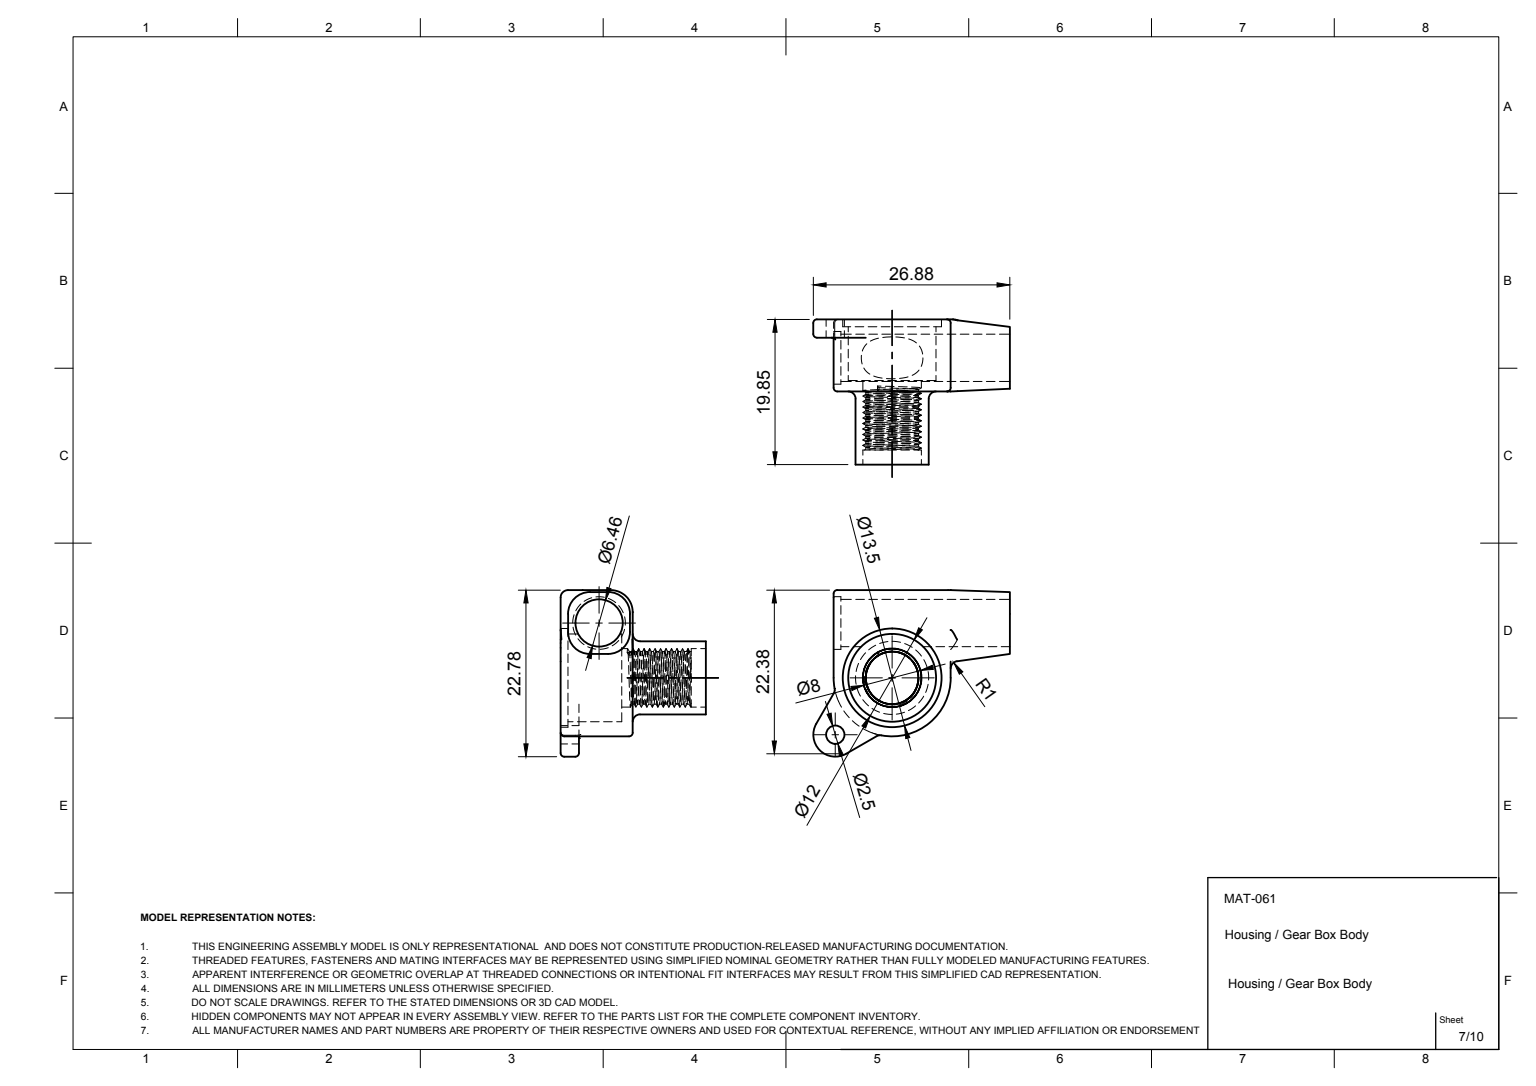
ISO-10303-21;
HEADER;
/* Generated by software containing ST-Developer
 * from STEP Tools, Inc. (www.steptools.com) 
 */

FILE_DESCRIPTION(
/* description */ ('', 'CAx-IF Rec.Pracs.---Representation and Presentation of Product Manufa
cturing Information (PMI)---4.0---2014-10-13'),
/* implementation_level */ '2;1');

FILE_NAME(
/* name */ 'Housing _ Gear Box Body.step',
/* time_stamp */ '2026-10-28T14:45:12+01:00',
/* author */ (''),
/* organization */ (''),
/* preprocessor_version */ 'ST-DEVELOPER v20.2',
/* originating_system */ 'Autodesk Translation Framework v15.17.0.0',
/* authorisation */ '');

FILE_SCHEMA (('AP242_MANAGED_MODEL_BASED_3D_ENGINEERING_MIM_LF { 1 0 10303 442 2 1 4 }'));
ENDSEC;

DATA;
#10=MECHANICAL_DESIGN_GEOMETRIC_PRESENTATION_REPRESENTATION('',(#265),#52164);
#116=ELLIPSE('',#10069,3.09185060411887,2.99998911300292);
#117=ELLIPSE('',#10070,0.558356536433831,0.540529130211527);
#118=ELLIPSE('',#10075,3.02534560825415,3.);
#119=ELLIPSE('',#10096,3.05201365986006,3.);
#120=ELLIPSE('',#10097,3.03164154875039,3.);
#121=ELLIPSE('',#10098,3.00479269659654,3.);
#122=ELLIPSE('',#10104,3.05599112671771,2.99998273953943);
#123=ELLIPSE('',#10106,0.477842904086099,0.430473129723059);
#124=ELLIPSE('',#10110,0.470434252195438,0.436250539297532);
#125=ELLIPSE('',#10111,0.502233427925589,0.501933027798313);
#126=ELLIPSE('',#10115,0.0333294784166319,0.012380355937192);
#180=(
BOUNDED_SURFACE()
B_SPLINE_SURFACE(3,3,((#43761,#43762,#43763,#43764,#43765,#43766,#43767,
#43768,#43769,#43770,#43771,#43772,#43773,#43774,#43775),(#43776,#43777,
#43778,#43779,#43780,#43781,#43782,#43783,#43784,#43785,#43786,#43787,#43788,
#43789,#43790),(#43791,#43792,#43793,#43794,#43795,#43796,#43797,#43798,
#43799,#43800,#43801,#43802,#43803,#43804,#43805),(#43806,#43807,#43808,
#43809,#43810,#43811,#43812,#43813,#43814,#43815,#43816,#43817,#43818,#43819,
#43820)),.UNSPECIFIED.,.F.,.F.,.F.)
B_SPLINE_SURFACE_WITH_KNOTS((4,4),(4,1,1,1,1,1,1,1,1,1,1,1,4),(0.,1.),(-0.02367250505126,
0.,0.1568376273924,0.2958784950045,0.4193835102427,0.5294996966959,0.6286414323947,
0.7182158704286,0.7992496439752,0.8730760680591,0.9399209839788,1.,1.025375300283),
 .UNSPECIFIED.)
GEOMETRIC_REPRESENTATION_ITEM()
RATIONAL_B_SPLINE_SURFACE(((1.19686984414,1.19686984414,1.19686984414,1.19686984414,
1.19686984414,1.19686984414,1.19686984414,1.19686984414,1.19686984414,1.19686984414,
1.19686984414,1.19686984414,1.19686984414,1.19686984414,1.19686984414),
(0.9343767186201,0.9343767186201,0.9343767186201,0.9343767186201,0.9343767186201,
0.9343767186201,0.9343767186201,0.9343767186201,0.9343767186201,0.9343767186201,
0.9343767186201,0.9343767186201,0.9343767186201,0.9343767186201,0.9343767186201),
(0.9343767186201,0.9343767186201,0.9343767186201,0.9343767186201,0.9343767186201,
0.9343767186201,0.9343767186201,0.9343767186201,0.9343767186201,0.9343767186201,
0.9343767186201,0.9343767186201,0.9343767186201,0.9343767186201,0.9343767186201),
(1.19686984414,1.19686984414,1.19686984414,1.19686984414,1.19686984414,
1.19686984414,1.19686984414,1.19686984414,1.19686984414,1.19686984414,1.19686984414,
1.19686984414,1.19686984414,1.19686984414,1.19686984414)))
REPRESENTATION_ITEM('')
SURFACE()
);
#181=(
BOUNDED_SURFACE()
B_SPLINE_SURFACE(3,3,((#43843,#43844,#43845,#43846,#43847,#43848,#43849,
#43850,#43851,#43852,#43853,#43854,#43855,#43856,#43857),(#43858,#43859,
#43860,#43861,#43862,#43863,#43864,#43865,#43866,#43867,#43868,#43869,#43870,
#43871,#43872),(#43873,#43874,#43875,#43876,#43877,#43878,#43879,#43880,
#43881,#43882,#43883,#43884,#43885,#43886,#43887),(#43888,#43889,#43890,
#43891,#43892,#43893,#43894,#43895,#43896,#43897,#43898,#43899,#43900,#43901,
#43902)),.UNSPECIFIED.,.F.,.F.,.F.)
B_SPLINE_SURFACE_WITH_KNOTS((4,4),(4,1,1,1,1,1,1,1,1,1,1,1,4),(0.,1.),(-0.02541201080131,
0.,0.06012137477617,0.127023679674,0.2009097013355,0.2820155865859,0.3717063075714,
0.470928205433,0.5809950476801,0.7044646083568,0.8434955500304,1.,1.023466062398),
 .UNSPECIFIED.)
GEOMETRIC_REPRESENTATION_ITEM()
RATIONAL_B_SPLINE_SURFACE(((1.196861975576,1.196861975576,1.196861975576,
1.196861975576,1.196861975576,1.196861975576,1.196861975576,1.196861975576,
1.196861975576,1.196861975576,1.196861975576,1.196861975576,1.196861975576,
1.196861975576,1.196861975576),(0.9343793414748,0.9343793414748,0.9343793414748,
0.9343793414748,0.9343793414748,0.9343793414748,0.9343793414748,0.9343793414748,
0.9343793414748,0.9343793414748,0.9343793414748,0.9343793414748,0.9343793414748,
0.9343793414748,0.9343793414748),(0.9343793414748,0.9343793414748,0.9343793414748,
0.9343793414748,0.9343793414748,0.9343793414748,0.9343793414748,0.9343793414748,
0.9343793414748,0.9343793414748,0.9343793414748,0.9343793414748,0.9343793414748,
0.9343793414748,0.9343793414748),(1.196861975576,1.196861975576,1.196861975576,
1.196861975576,1.196861975576,1.196861975576,1.196861975576,1.196861975576,
1.196861975576,1.196861975576,1.196861975576,1.196861975576,1.196861975576,
1.196861975576,1.196861975576)))
REPRESENTATION_ITEM('')
SURFACE()
);
#182=(
BOUNDED_SURFACE()
B_SPLINE_SURFACE(3,3,((#44165,#44166,#44167,#44168,#44169,#44170,#44171,
#44172,#44173,#44174,#44175,#44176,#44177,#44178,#44179,#44180,#44181,#44182,
#44183,#44184,#44185),(#44186,#44187,#44188,#44189,#44190,#44191,#44192,
#44193,#44194,#44195,#44196,#44197,#44198,#44199,#44200,#44201,#44202,#44203,
#44204,#44205,#44206),(#44207,#44208,#44209,#44210,#44211,#44212,#44213,
#44214,#44215,#44216,#44217,#44218,#44219,#44220,#44221,#44222,#44223,#44224,
#44225,#44226,#44227),(#44228,#44229,#44230,#44231,#44232,#44233,#44234,
#44235,#44236,#44237,#44238,#44239,#44240,#44241,#44242,#44243,#44244,#44245,
#44246,#44247,#44248)),.UNSPECIFIED.,.F.,.F.,.F.)
B_SPLINE_SURFACE_WITH_KNOTS((4,4),(4,1,1,1,1,1,1,1,1,1,1,1,1,1,1,1,1,1,
4),(0.,1.),(-0.004474348485776,0.,0.02230597305244,0.04333157365729,0.06387325262822,
0.08408116383947,0.1041708278111,0.1243458370088,0.1448121265696,0.1657786860045,
0.187470853701,0.210486087144,0.2358855836333,0.2645487659469,0.2971408212892,
0.3344049750459,0.3761308583034,0.4203483673292,0.4513668076816),
 .UNSPECIFIED.)
GEOMETRIC_REPRESENTATION_ITEM()
RATIONAL_B_SPLINE_SURFACE(((1.162548312769,1.162548312769,1.162548312769,
1.162548312769,1.162548312769,1.162548312769,1.162548312769,1.162548312769,
1.162548312769,1.162548312769,1.162548312769,1.162548312769,1.162548312769,
1.162548312769,1.162548312769,1.162548312769,1.162548312769,1.162548312769,
1.162548312769,1.162548312769,1.162548312769),(0.9458172290769,0.9458172290769,
0.9458172290769,0.9458172290769,0.9458172290769,0.9458172290769,0.9458172290769,
0.9458172290769,0.9458172290769,0.9458172290769,0.9458172290769,0.9458172290769,
0.9458172290769,0.9458172290769,0.9458172290769,0.9458172290769,0.9458172290769,
0.9458172290769,0.9458172290769,0.9458172290769,0.9458172290769),(0.9458172290769,
0.9458172290769,0.9458172290769,0.9458172290769,0.9458172290769,0.9458172290769,
0.9458172290769,0.9458172290769,0.9458172290769,0.9458172290769,0.9458172290769,
0.9458172290769,0.9458172290769,0.9458172290769,0.9458172290769,0.9458172290769,
0.9458172290769,0.9458172290769,0.9458172290769,0.9458172290769,0.9458172290769),
(1.162548312769,1.162548312769,1.162548312769,1.162548312769,1.162548312769,
1.162548312769,1.162548312769,1.162548312769,1.162548312769,1.162548312769,
1.162548312769,1.162548312769,1.162548312769,1.162548312769,1.162548312769,
1.162548312769,1.162548312769,1.162548312769,1.162548312769,1.162548312769,
1.162548312769)))
REPRESENTATION_ITEM('')
SURFACE()
);
#183=(
BOUNDED_SURFACE()
B_SPLINE_SURFACE(3,3,((#44380,#44381,#44382,#44383,#44384,#44385,#44386,
#44387,#44388,#44389,#44390,#44391,#44392,#44393,#44394,#44395,#44396,#44397,
#44398,#44399,#44400,#44401,#44402),(#44403,#44404,#44405,#44406,#44407,
#44408,#44409,#44410,#44411,#44412,#44413,#44414,#44415,#44416,#44417,#44418,
#44419,#44420,#44421,#44422,#44423,#44424,#44425),(#44426,#44427,#44428,
#44429,#44430,#44431,#44432,#44433,#44434,#44435,#44436,#44437,#44438,#44439,
#44440,#44441,#44442,#44443,#44444,#44445,#44446,#44447,#44448),(#44449,
#44450,#44451,#44452,#44453,#44454,#44455,#44456,#44457,#44458,#44459,#44460,
#44461,#44462,#44463,#44464,#44465,#44466,#44467,#44468,#44469,#44470,#44471)),
 .UNSPECIFIED.,.F.,.F.,.F.)
B_SPLINE_SURFACE_WITH_KNOTS((4,4),(4,1,1,1,1,1,1,1,1,1,1,1,1,1,1,1,1,1,
1,1,4),(0.,1.),(0.4402361434422,0.4558088659294,0.476422669633,0.4969107659322,
0.5173847665671,0.5378040004898,0.5584587769075,0.5804853326365,0.6053681688744,
0.6337471320501,0.6648770320844,0.697628000239,0.7315220485564,0.7658606197272,
0.7995217313545,0.8327434657359,0.8676912667687,0.9066066156032,0.9504140537645,
1.,1.005363326625),.UNSPECIFIED.)
GEOMETRIC_REPRESENTATION_ITEM()
RATIONAL_B_SPLINE_SURFACE(((1.224498979605,1.224498979605,1.224498979605,
1.224498979605,1.224498979605,1.224498979605,1.224498979605,1.224498979605,
1.224498979605,1.224498979605,1.224498979605,1.224498979605,1.224498979605,
1.224498979605,1.224498979605,1.224498979605,1.224498979605,1.224498979605,
1.224498979605,1.224498979605,1.224498979605,1.224498979605,1.224498979605),
(0.9251670067983,0.9251670067983,0.9251670067983,0.9251670067983,0.9251670067983,
0.9251670067983,0.9251670067983,0.9251670067983,0.9251670067983,0.9251670067983,
0.9251670067983,0.9251670067983,0.9251670067983,0.9251670067983,0.9251670067983,
0.9251670067983,0.9251670067983,0.9251670067983,0.9251670067983,0.9251670067983,
0.9251670067983,0.9251670067983,0.9251670067983),(0.9251670067983,0.9251670067983,
0.9251670067983,0.9251670067983,0.9251670067983,0.9251670067983,0.9251670067983,
0.9251670067983,0.9251670067983,0.9251670067983,0.9251670067983,0.9251670067983,
0.9251670067983,0.9251670067983,0.9251670067983,0.9251670067983,0.9251670067983,
0.9251670067983,0.9251670067983,0.9251670067983,0.9251670067983,0.9251670067983,
0.9251670067983),(1.224498979605,1.224498979605,1.224498979605,1.224498979605,
1.224498979605,1.224498979605,1.224498979605,1.224498979605,1.224498979605,
1.224498979605,1.224498979605,1.224498979605,1.224498979605,1.224498979605,
1.224498979605,1.224498979605,1.224498979605,1.224498979605,1.224498979605,
1.224498979605,1.224498979605,1.224498979605,1.224498979605)))
REPRESENTATION_ITEM('')
SURFACE()
);
#184=(
BOUNDED_SURFACE()
B_SPLINE_SURFACE(3,3,((#44501,#44502,#44503,#44504,#44505,#44506,#44507,
#44508),(#44509,#44510,#44511,#44512,#44513,#44514,#44515,#44516),(#44517,
#44518,#44519,#44520,#44521,#44522,#44523,#44524),(#44525,#44526,#44527,
#44528,#44529,#44530,#44531,#44532)),.UNSPECIFIED.,.F.,.F.,.F.)
B_SPLINE_SURFACE_WITH_KNOTS((4,4),(4,1,1,1,1,4),(0.,1.),(-0.02000817581934,
0.,0.3335678568848,0.6667501113936,1.,1.020000171272),.UNSPECIFIED.)
GEOMETRIC_REPRESENTATION_ITEM()
RATIONAL_B_SPLINE_SURFACE(((1.001084776474,1.001084776474,1.001084776474,
1.001084776474,1.001084776474,1.001084776474,1.001084776474,1.001084776474),
(0.9996384078421,0.9996384078421,0.9996384078421,0.9996384078421,0.9996384078421,
0.9996384078421,0.9996384078421,0.9996384078421),(0.9996384078421,0.9996384078421,
0.9996384078421,0.9996384078421,0.9996384078421,0.9996384078421,0.9996384078421,
0.9996384078421),(1.001084776474,1.001084776474,1.001084776474,1.001084776474,
1.001084776474,1.001084776474,1.001084776474,1.001084776474)))
REPRESENTATION_ITEM('')
SURFACE()
);
#185=(
BOUNDED_SURFACE()
B_SPLINE_SURFACE(3,3,((#44717,#44718,#44719,#44720,#44721,#44722,#44723,
#44724,#44725),(#44726,#44727,#44728,#44729,#44730,#44731,#44732,#44733,
#44734),(#44735,#44736,#44737,#44738,#44739,#44740,#44741,#44742,#44743),
(#44744,#44745,#44746,#44747,#44748,#44749,#44750,#44751,#44752)),
 .UNSPECIFIED.,.F.,.F.,.F.)
B_SPLINE_SURFACE_WITH_KNOTS((4,4),(4,1,1,1,1,1,4),(0.,1.),(0.01341438395161,
0.2268259504049,0.4456307994234,0.6496269485443,0.8352622055157,1.,1.015518229442),
 .UNSPECIFIED.)
GEOMETRIC_REPRESENTATION_ITEM()
RATIONAL_B_SPLINE_SURFACE(((1.058064131412,1.058064131412,1.058064131412,
1.058064131412,1.058064131412,1.058064131412,1.058064131412,1.058064131412,
1.058064131412),(0.9806452895294,0.9806452895294,0.9806452895294,0.9806452895294,
0.9806452895294,0.9806452895294,0.9806452895294,0.9806452895294,0.9806452895294),
(0.9806452895294,0.9806452895294,0.9806452895294,0.9806452895294,0.9806452895294,
0.9806452895294,0.9806452895294,0.9806452895294,0.9806452895294),(1.058064131412,
1.058064131412,1.058064131412,1.058064131412,1.058064131412,1.058064131412,
1.058064131412,1.058064131412,1.058064131412)))
REPRESENTATION_ITEM('')
SURFACE()
);
#186=(
BOUNDED_SURFACE()
B_SPLINE_SURFACE(3,3,((#44798,#44799,#44800,#44801,#44802,#44803,#44804,
#44805,#44806,#44807,#44808),(#44809,#44810,#44811,#44812,#44813,#44814,
#44815,#44816,#44817,#44818,#44819),(#44820,#44821,#44822,#44823,#44824,
#44825,#44826,#44827,#44828,#44829,#44830),(#44831,#44832,#44833,#44834,
#44835,#44836,#44837,#44838,#44839,#44840,#44841)),.UNSPECIFIED.,.F.,.F.,
 .F.)
B_SPLINE_SURFACE_WITH_KNOTS((4,4),(4,1,1,1,1,1,1,1,4),(0.,1.),(-0.01514694021523,
0.,0.1434382549194,0.2925803126927,0.4539877256396,0.6288947339363,0.8127593843745,
1.,1.01468871823),.UNSPECIFIED.)
GEOMETRIC_REPRESENTATION_ITEM()
RATIONAL_B_SPLINE_SURFACE(((1.091722184379,1.091722184379,1.091722184379,
1.091722184379,1.091722184379,1.091722184379,1.091722184379,1.091722184379,
1.091722184379,1.091722184379,1.091722184379),(0.9694259385405,0.9694259385405,
0.9694259385405,0.9694259385405,0.9694259385405,0.9694259385405,0.9694259385405,
0.9694259385405,0.9694259385405,0.9694259385405,0.9694259385405),(0.9694259385405,
0.9694259385405,0.9694259385405,0.9694259385405,0.9694259385405,0.9694259385405,
0.9694259385405,0.9694259385405,0.9694259385405,0.9694259385405,0.9694259385405),
(1.091722184379,1.091722184379,1.091722184379,1.091722184379,1.091722184379,
1.091722184379,1.091722184379,1.091722184379,1.091722184379,1.091722184379,
1.091722184379)))
REPRESENTATION_ITEM('')
SURFACE()
);
#187=(
BOUNDED_SURFACE()
B_SPLINE_SURFACE(3,3,((#44843,#44844,#44845,#44846,#44847,#44848,#44849,
#44850,#44851,#44852),(#44853,#44854,#44855,#44856,#44857,#44858,#44859,
#44860,#44861,#44862),(#44863,#44864,#44865,#44866,#44867,#44868,#44869,
#44870,#44871,#44872),(#44873,#44874,#44875,#44876,#44877,#44878,#44879,
#44880,#44881,#44882)),.UNSPECIFIED.,.F.,.F.,.F.)
B_SPLINE_SURFACE_WITH_KNOTS((4,4),(4,1,1,1,1,1,1,4),(0.,1.),(-0.1017343672885,
0.,0.1958839083417,0.3858642890747,0.5744654073669,0.7741715521339,1.,1.116420456884),
 .UNSPECIFIED.)
GEOMETRIC_REPRESENTATION_ITEM()
RATIONAL_B_SPLINE_SURFACE(((1.126722516535,1.126722516535,1.126722516535,
1.126722516535,1.126722516535,1.126722516535,1.126722516535,1.126722516535,
1.126722516535,1.126722516535),(0.9577591611551,0.9577591611551,0.9577591611551,
0.9577591611551,0.9577591611551,0.9577591611551,0.9577591611551,0.9577591611551,
0.9577591611551,0.9577591611551),(0.9577591611551,0.9577591611551,0.9577591611551,
0.9577591611551,0.9577591611551,0.9577591611551,0.9577591611551,0.9577591611551,
0.9577591611551,0.9577591611551),(1.126722516535,1.126722516535,1.126722516535,
1.126722516535,1.126722516535,1.126722516535,1.126722516535,1.126722516535,
1.126722516535,1.126722516535)))
REPRESENTATION_ITEM('')
SURFACE()
);
#188=(
BOUNDED_SURFACE()
B_SPLINE_SURFACE(3,3,((#44916,#44917,#44918,#44919,#44920,#44921,#44922,
#44923,#44924,#44925,#44926,#44927,#44928,#44929),(#44930,#44931,#44932,
#44933,#44934,#44935,#44936,#44937,#44938,#44939,#44940,#44941,#44942,#44943),
(#44944,#44945,#44946,#44947,#44948,#44949,#44950,#44951,#44952,#44953,
#44954,#44955,#44956,#44957),(#44958,#44959,#44960,#44961,#44962,#44963,
#44964,#44965,#44966,#44967,#44968,#44969,#44970,#44971)),.UNSPECIFIED.,
 .F.,.F.,.F.)
B_SPLINE_SURFACE_WITH_KNOTS((4,4),(4,1,1,1,1,1,1,1,1,1,1,4),(0.,1.),(-0.01844658935295,
0.,0.1044814008579,0.2134723510049,0.3264520754444,0.4425667333534,0.5596708840584,
0.6752555152391,0.7879010159006,0.8964334098892,1.,1.018329622104),
 .UNSPECIFIED.)
GEOMETRIC_REPRESENTATION_ITEM()
RATIONAL_B_SPLINE_SURFACE(((1.093920437843,1.093920437843,1.093920437843,
1.093920437843,1.093920437843,1.093920437843,1.093920437843,1.093920437843,
1.093920437843,1.093920437843,1.093920437843,1.093920437843,1.093920437843,
1.093920437843),(0.9686931873855,0.9686931873855,0.9686931873855,0.9686931873855,
0.9686931873855,0.9686931873855,0.9686931873855,0.9686931873855,0.9686931873855,
0.9686931873855,0.9686931873855,0.9686931873855,0.9686931873855,0.9686931873855),
(0.9686931873855,0.9686931873855,0.9686931873855,0.9686931873855,0.9686931873855,
0.9686931873855,0.9686931873855,0.9686931873855,0.9686931873855,0.9686931873855,
0.9686931873855,0.9686931873855,0.9686931873855,0.9686931873855),(1.093920437843,
1.093920437843,1.093920437843,1.093920437843,1.093920437843,1.093920437843,
1.093920437843,1.093920437843,1.093920437843,1.093920437843,1.093920437843,
1.093920437843,1.093920437843,1.093920437843)))
REPRESENTATION_ITEM('')
SURFACE()
);
#189=(
BOUNDED_SURFACE()
B_SPLINE_SURFACE(3,3,((#45064,#45065,#45066,#45067,#45068,#45069,#45070,
#45071,#45072,#45073,#45074,#45075),(#45076,#45077,#45078,#45079,#45080,
#45081,#45082,#45083,#45084,#45085,#45086,#45087),(#45088,#45089,#45090,
#45091,#45092,#45093,#45094,#45095,#45096,#45097,#45098,#45099),(#45100,
#45101,#45102,#45103,#45104,#45105,#45106,#45107,#45108,#45109,#45110,#45111)),
 .UNSPECIFIED.,.F.,.F.,.F.)
B_SPLINE_SURFACE_WITH_KNOTS((4,4),(4,1,1,1,1,1,1,1,1,4),(0.,1.),(-0.030614617578,
0.,0.1495462512719,0.2937414136624,0.4389937202877,0.5830269670076,0.7175783131859,
0.8510090101071,1.,1.030661227764),.UNSPECIFIED.)
GEOMETRIC_REPRESENTATION_ITEM()
RATIONAL_B_SPLINE_SURFACE(((1.129761691476,1.129761691476,1.129761691476,
1.129761691476,1.129761691476,1.129761691476,1.129761691476,1.129761691476,
1.129761691476,1.129761691476,1.129761691476,1.129761691476),(0.9567461028415,
0.9567461028415,0.9567461028415,0.9567461028415,0.9567461028415,0.9567461028415,
0.9567461028415,0.9567461028415,0.9567461028415,0.9567461028415,0.9567461028415,
0.9567461028415),(0.9567461028415,0.9567461028415,0.9567461028415,0.9567461028415,
0.9567461028415,0.9567461028415,0.9567461028415,0.9567461028415,0.9567461028415,
0.9567461028415,0.9567461028415,0.9567461028415),(1.129761691476,1.129761691476,
1.129761691476,1.129761691476,1.129761691476,1.129761691476,1.129761691476,
1.129761691476,1.129761691476,1.129761691476,1.129761691476,1.129761691476)))
REPRESENTATION_ITEM('')
SURFACE()
);
#190=(
BOUNDED_SURFACE()
B_SPLINE_SURFACE(2,2,((#45185,#45186,#45187),(#45188,#45189,#45190),(#45191,
#45192,#45193)),.UNSPECIFIED.,.F.,.F.,.F.)
B_SPLINE_SURFACE_WITH_KNOTS((3,3),(3,3),(-1.57079632679603,1.03155351707746E-11),
(-0.78539816371462,0.785398163714621),.UNSPECIFIED.)
GEOMETRIC_REPRESENTATION_ITEM()
RATIONAL_B_SPLINE_SURFACE(((1.,0.707106780962273,1.),(0.707106781182504,
0.499999999838555,0.707106781182504),(1.,0.707106780962273,1.)))
REPRESENTATION_ITEM('')
SURFACE()
);
#191=(
BOUNDED_SURFACE()
B_SPLINE_SURFACE(3,3,((#45244,#45245,#45246,#45247,#45248,#45249,#45250,
#45251,#45252,#45253,#45254,#45255,#45256,#45257,#45258,#45259,#45260,#45261,
#45262,#45263),(#45264,#45265,#45266,#45267,#45268,#45269,#45270,#45271,
#45272,#45273,#45274,#45275,#45276,#45277,#45278,#45279,#45280,#45281,#45282,
#45283),(#45284,#45285,#45286,#45287,#45288,#45289,#45290,#45291,#45292,
#45293,#45294,#45295,#45296,#45297,#45298,#45299,#45300,#45301,#45302,#45303),
(#45304,#45305,#45306,#45307,#45308,#45309,#45310,#45311,#45312,#45313,
#45314,#45315,#45316,#45317,#45318,#45319,#45320,#45321,#45322,#45323)),
 .UNSPECIFIED.,.F.,.F.,.F.)
B_SPLINE_SURFACE_WITH_KNOTS((4,4),(4,1,1,1,1,1,1,1,1,1,1,1,1,1,1,1,1,4),
(0.,1.),(0.5974830130601,0.6214330811425,0.6582317938511,0.6909396382487,
0.7201206288693,0.746316287089,0.7702754291775,0.7929187871877,0.814921182593,
0.8365329597553,0.8579099550699,0.8792500682455,0.9008111437527,0.9227739349606,
0.9458934201391,0.9712943791051,1.,1.003985211551),.UNSPECIFIED.)
GEOMETRIC_REPRESENTATION_ITEM()
RATIONAL_B_SPLINE_SURFACE(((1.163141288766,1.163141288766,1.163141288766,
1.163141288766,1.163141288766,1.163141288766,1.163141288766,1.163141288766,
1.163141288766,1.163141288766,1.163141288766,1.163141288766,1.163141288766,
1.163141288766,1.163141288766,1.163141288766,1.163141288766,1.163141288766,
1.163141288766,1.163141288766),(0.9456195704113,0.9456195704113,0.9456195704113,
0.9456195704113,0.9456195704113,0.9456195704113,0.9456195704113,0.9456195704113,
0.9456195704113,0.9456195704113,0.9456195704113,0.9456195704113,0.9456195704113,
0.9456195704113,0.9456195704113,0.9456195704113,0.9456195704113,0.9456195704113,
0.9456195704113,0.9456195704113),(0.9456195704113,0.9456195704113,0.9456195704113,
0.9456195704113,0.9456195704113,0.9456195704113,0.9456195704113,0.9456195704113,
0.9456195704113,0.9456195704113,0.9456195704113,0.9456195704113,0.9456195704113,
0.9456195704113,0.9456195704113,0.9456195704113,0.9456195704113,0.9456195704113,
0.9456195704113,0.9456195704113),(1.163141288766,1.163141288766,1.163141288766,
1.163141288766,1.163141288766,1.163141288766,1.163141288766,1.163141288766,
1.163141288766,1.163141288766,1.163141288766,1.163141288766,1.163141288766,
1.163141288766,1.163141288766,1.163141288766,1.163141288766,1.163141288766,
1.163141288766,1.163141288766)))
REPRESENTATION_ITEM('')
SURFACE()
);
#192=(
BOUNDED_SURFACE()
B_SPLINE_SURFACE(3,3,((#45441,#45442,#45443,#45444,#45445,#45446,#45447,
#45448,#45449,#45450,#45451,#45452,#45453,#45454,#45455,#45456,#45457,#45458),
(#45459,#45460,#45461,#45462,#45463,#45464,#45465,#45466,#45467,#45468,
#45469,#45470,#45471,#45472,#45473,#45474,#45475,#45476),(#45477,#45478,
#45479,#45480,#45481,#45482,#45483,#45484,#45485,#45486,#45487,#45488,#45489,
#45490,#45491,#45492,#45493,#45494),(#45495,#45496,#45497,#45498,#45499,
#45500,#45501,#45502,#45503,#45504,#45505,#45506,#45507,#45508,#45509,#45510,
#45511,#45512)),.UNSPECIFIED.,.F.,.F.,.F.)
B_SPLINE_SURFACE_WITH_KNOTS((4,4),(4,1,1,1,1,1,1,1,1,1,1,1,1,1,1,4),(0.,
1.),(-0.003641476161696,0.,0.03996584306645,0.07565969810702,0.107705792552,
0.1364673868443,0.1623976598809,0.1860106967015,0.2078779981353,0.2287055315989,
0.2494804366836,0.2705832190163,0.2914915459405,0.3122164361973,0.3338956761934,
0.3478416898621),.UNSPECIFIED.)
GEOMETRIC_REPRESENTATION_ITEM()
RATIONAL_B_SPLINE_SURFACE(((1.224501069917,1.224501069917,1.224501069917,
1.224501069917,1.224501069917,1.224501069917,1.224501069917,1.224501069917,
1.224501069917,1.224501069917,1.224501069917,1.224501069917,1.224501069917,
1.224501069917,1.224501069917,1.224501069917,1.224501069917,1.224501069917),
(0.9251663100277,0.9251663100277,0.9251663100277,0.9251663100277,0.9251663100277,
0.9251663100277,0.9251663100277,0.9251663100277,0.9251663100277,0.9251663100277,
0.9251663100277,0.9251663100277,0.9251663100277,0.9251663100277,0.9251663100277,
0.9251663100277,0.9251663100277,0.9251663100277),(0.9251663100277,0.9251663100277,
0.9251663100277,0.9251663100277,0.9251663100277,0.9251663100277,0.9251663100277,
0.9251663100277,0.9251663100277,0.9251663100277,0.9251663100277,0.9251663100277,
0.9251663100277,0.9251663100277,0.9251663100277,0.9251663100277,0.9251663100277,
0.9251663100277),(1.224501069917,1.224501069917,1.224501069917,1.224501069917,
1.224501069917,1.224501069917,1.224501069917,1.224501069917,1.224501069917,
1.224501069917,1.224501069917,1.224501069917,1.224501069917,1.224501069917,
1.224501069917,1.224501069917,1.224501069917,1.224501069917)))
REPRESENTATION_ITEM('')
SURFACE()
);
#193=(
BOUNDED_SURFACE()
B_SPLINE_SURFACE(3,3,((#45594,#45595,#45596,#45597,#45598,#45599,#45600,
#45601,#45602,#45603,#45604,#45605,#45606),(#45607,#45608,#45609,#45610,
#45611,#45612,#45613,#45614,#45615,#45616,#45617,#45618,#45619),(#45620,
#45621,#45622,#45623,#45624,#45625,#45626,#45627,#45628,#45629,#45630,#45631,
#45632),(#45633,#45634,#45635,#45636,#45637,#45638,#45639,#45640,#45641,
#45642,#45643,#45644,#45645)),.UNSPECIFIED.,.F.,.F.,.F.)
B_SPLINE_SURFACE_WITH_KNOTS((4,4),(4,1,1,1,1,1,1,1,1,1,4),(0.,1.),(-0.0103387915936,
0.,0.1251367424062,0.2492492298603,0.3735032958992,0.4979081598552,0.6224043335643,
0.7477267861541,0.8737422387189,1.,1.010148865997),.UNSPECIFIED.)
GEOMETRIC_REPRESENTATION_ITEM()
RATIONAL_B_SPLINE_SURFACE(((1.000215851129,1.000215851129,1.000215851129,
1.000215851129,1.000215851129,1.000215851129,1.000215851129,1.000215851129,
1.000215851129,1.000215851129,1.000215851129,1.000215851129,1.000215851129),
(0.9999280496237,0.9999280496237,0.9999280496237,0.9999280496237,0.9999280496237,
0.9999280496237,0.9999280496237,0.9999280496237,0.9999280496237,0.9999280496237,
0.9999280496237,0.9999280496237,0.9999280496237),(0.9999280496237,0.9999280496237,
0.9999280496237,0.9999280496237,0.9999280496237,0.9999280496237,0.9999280496237,
0.9999280496237,0.9999280496237,0.9999280496237,0.9999280496237,0.9999280496237,
0.9999280496237),(1.000215851129,1.000215851129,1.000215851129,1.000215851129,
1.000215851129,1.000215851129,1.000215851129,1.000215851129,1.000215851129,
1.000215851129,1.000215851129,1.000215851129,1.000215851129)))
REPRESENTATION_ITEM('')
SURFACE()
);
#194=(
BOUNDED_SURFACE()
B_SPLINE_SURFACE(3,3,((#45713,#45714,#45715,#45716,#45717,#45718,#45719,
#45720),(#45721,#45722,#45723,#45724,#45725,#45726,#45727,#45728),(#45729,
#45730,#45731,#45732,#45733,#45734,#45735,#45736),(#45737,#45738,#45739,
#45740,#45741,#45742,#45743,#45744)),.UNSPECIFIED.,.F.,.F.,.F.)
B_SPLINE_SURFACE_WITH_KNOTS((4,4),(4,1,1,1,1,4),(0.,1.),(-0.02002688240655,
0.,0.3332292460223,0.6664005931354,1.,1.020557756204),.UNSPECIFIED.)
GEOMETRIC_REPRESENTATION_ITEM()
RATIONAL_B_SPLINE_SURFACE(((1.00007870989,1.00007870989,1.00007870989,1.00007870989,
1.00007870989,1.00007870989,1.00007870989,1.00007870989),(0.9999737633701,
0.9999737633701,0.9999737633701,0.9999737633701,0.9999737633701,0.9999737633701,
0.9999737633701,0.9999737633701),(0.9999737633701,0.9999737633701,0.9999737633701,
0.9999737633701,0.9999737633701,0.9999737633701,0.9999737633701,0.9999737633701),
(1.00007870989,1.00007870989,1.00007870989,1.00007870989,1.00007870989,
1.00007870989,1.00007870989,1.00007870989)))
REPRESENTATION_ITEM('')
SURFACE()
);
#195=(
BOUNDED_SURFACE()
B_SPLINE_SURFACE(3,3,((#45748,#45749,#45750,#45751,#45752,#45753,#45754,
#45755,#45756,#45757,#45758,#45759,#45760,#45761,#45762,#45763,#45764,#45765,
#45766),(#45767,#45768,#45769,#45770,#45771,#45772,#45773,#45774,#45775,
#45776,#45777,#45778,#45779,#45780,#45781,#45782,#45783,#45784,#45785),
(#45786,#45787,#45788,#45789,#45790,#45791,#45792,#45793,#45794,#45795,
#45796,#45797,#45798,#45799,#45800,#45801,#45802,#45803,#45804),(#45805,
#45806,#45807,#45808,#45809,#45810,#45811,#45812,#45813,#45814,#45815,#45816,
#45817,#45818,#45819,#45820,#45821,#45822,#45823)),.UNSPECIFIED.,.F.,.F.,
 .F.)
B_SPLINE_SURFACE_WITH_KNOTS((4,4),(4,1,1,1,1,1,1,1,1,1,1,1,1,1,1,1,4),(0.,
1.),(-0.01435280055262,0.,0.1052237534203,0.2024514847669,0.2919074772468,
0.3731001338908,0.4462221459727,0.5125974112795,0.574182113677,0.6331082197362,
0.6912681104287,0.7496322505172,0.8078577516813,0.8672149095682,0.9304407269683,
1.,1.014830854834),.UNSPECIFIED.)
GEOMETRIC_REPRESENTATION_ITEM()
RATIONAL_B_SPLINE_SURFACE(((1.087955100757,1.087955100757,1.087955100757,
1.087955100757,1.087955100757,1.087955100757,1.087955100757,1.087955100757,
1.087955100757,1.087955100757,1.087955100757,1.087955100757,1.087955100757,
1.087955100757,1.087955100757,1.087955100757,1.087955100757,1.087955100757,
1.087955100757),(0.970681633081,0.970681633081,0.970681633081,0.970681633081,
0.970681633081,0.970681633081,0.970681633081,0.970681633081,0.970681633081,
0.970681633081,0.970681633081,0.970681633081,0.970681633081,0.970681633081,
0.970681633081,0.970681633081,0.970681633081,0.970681633081,0.970681633081),
(0.970681633081,0.970681633081,0.970681633081,0.970681633081,0.970681633081,
0.970681633081,0.970681633081,0.970681633081,0.970681633081,0.970681633081,
0.970681633081,0.970681633081,0.970681633081,0.970681633081,0.970681633081,
0.970681633081,0.970681633081,0.970681633081,0.970681633081),(1.087955100757,
1.087955100757,1.087955100757,1.087955100757,1.087955100757,1.087955100757,
1.087955100757,1.087955100757,1.087955100757,1.087955100757,1.087955100757,
1.087955100757,1.087955100757,1.087955100757,1.087955100757,1.087955100757,
1.087955100757,1.087955100757,1.087955100757)))
REPRESENTATION_ITEM('')
SURFACE()
);
#196=(
BOUNDED_SURFACE()
B_SPLINE_SURFACE(3,3,((#45942,#45943,#45944,#45945,#45946,#45947,#45948,
#45949,#45950,#45951),(#45952,#45953,#45954,#45955,#45956,#45957,#45958,
#45959,#45960,#45961),(#45962,#45963,#45964,#45965,#45966,#45967,#45968,
#45969,#45970,#45971),(#45972,#45973,#45974,#45975,#45976,#45977,#45978,
#45979,#45980,#45981)),.UNSPECIFIED.,.F.,.F.,.F.)
B_SPLINE_SURFACE_WITH_KNOTS((4,4),(4,1,1,1,1,1,1,4),(0.,1.),(-0.01569017456562,
0.,0.1634721590841,0.348317956625,0.5531428960446,0.7725802144006,1.,1.008112438365),
 .UNSPECIFIED.)
GEOMETRIC_REPRESENTATION_ITEM()
RATIONAL_B_SPLINE_SURFACE(((1.059581909356,1.059581909356,1.059581909356,
1.059581909356,1.059581909356,1.059581909356,1.059581909356,1.059581909356,
1.059581909356,1.059581909356),(0.9801393635479,0.9801393635479,0.9801393635479,
0.9801393635479,0.9801393635479,0.9801393635479,0.9801393635479,0.9801393635479,
0.9801393635479,0.9801393635479),(0.9801393635479,0.9801393635479,0.9801393635479,
0.9801393635479,0.9801393635479,0.9801393635479,0.9801393635479,0.9801393635479,
0.9801393635479,0.9801393635479),(1.059581909356,1.059581909356,1.059581909356,
1.059581909356,1.059581909356,1.059581909356,1.059581909356,1.059581909356,
1.059581909356,1.059581909356)))
REPRESENTATION_ITEM('')
SURFACE()
);
#197=(
BOUNDED_SURFACE()
B_SPLINE_SURFACE(3,3,((#45982,#45983,#45984,#45985,#45986,#45987,#45988,
#45989,#45990,#45991),(#45992,#45993,#45994,#45995,#45996,#45997,#45998,
#45999,#46000,#46001),(#46002,#46003,#46004,#46005,#46006,#46007,#46008,
#46009,#46010,#46011),(#46012,#46013,#46014,#46015,#46016,#46017,#46018,
#46019,#46020,#46021)),.UNSPECIFIED.,.F.,.F.,.F.)
B_SPLINE_SURFACE_WITH_KNOTS((4,4),(4,1,1,1,1,1,1,4),(0.,1.),(-0.1276752045009,
0.,0.177977214136,0.3579508099613,0.5526671794136,0.7657440822575,1.,1.101553192821),
 .UNSPECIFIED.)
GEOMETRIC_REPRESENTATION_ITEM()
RATIONAL_B_SPLINE_SURFACE(((1.12652088875,1.12652088875,1.12652088875,1.12652088875,
1.12652088875,1.12652088875,1.12652088875,1.12652088875,1.12652088875,1.12652088875),
(0.9578263704167,0.9578263704167,0.9578263704167,0.9578263704167,0.9578263704167,
0.9578263704167,0.9578263704167,0.9578263704167,0.9578263704167,0.9578263704167),
(0.9578263704167,0.9578263704167,0.9578263704167,0.9578263704167,0.9578263704167,
0.9578263704167,0.9578263704167,0.9578263704167,0.9578263704167,0.9578263704167),
(1.12652088875,1.12652088875,1.12652088875,1.12652088875,1.12652088875,
1.12652088875,1.12652088875,1.12652088875,1.12652088875,1.12652088875)))
REPRESENTATION_ITEM('')
SURFACE()
);
#220=TOROIDAL_SURFACE('',#9991,6.,1.);
#221=TOROIDAL_SURFACE('',#10030,9.,1.);
#222=TOROIDAL_SURFACE('',#10036,1.5,0.5);
#223=TOROIDAL_SURFACE('',#10044,2.5,0.5);
#224=TOROIDAL_SURFACE('',#10048,2.5,0.5);
#225=TOROIDAL_SURFACE('',#10055,1.5,0.5);
#226=TOROIDAL_SURFACE('',#10057,7.5,0.5);
#227=TOROIDAL_SURFACE('',#10063,7.5,0.5);
#228=TOROIDAL_SURFACE('',#10121,2.5,0.5);
#229=TOROIDAL_SURFACE('',#10126,7.5,0.5);
#239=SHAPE_REPRESENTATION_RELATIONSHIP('SRR','None',#52218,#252);
#252=ADVANCED_BREP_SHAPE_REPRESENTATION('',(#278),#52158);
#265=STYLED_ITEM('',(#52297),#278);
#278=MANIFOLD_SOLID_BREP('Body1',#9125);
#304=FACE_BOUND('',#1477,.T.);
#305=FACE_BOUND('',#1481,.T.);
#306=FACE_BOUND('',#1499,.T.);
#307=FACE_BOUND('',#1501,.T.);
#308=FACE_BOUND('',#1503,.T.);
#309=FACE_BOUND('',#1506,.T.);
#310=FACE_BOUND('',#1507,.T.);
#311=FACE_BOUND('',#1510,.T.);
#312=FACE_BOUND('',#1545,.T.);
#313=FACE_BOUND('',#1548,.T.);
#314=FACE_BOUND('',#1551,.T.);
#388=B_SPLINE_SURFACE_WITH_KNOTS('',3,3,((#40199,#40200,#40201,#40202,#40203,
#40204,#40205,#40206,#40207,#40208,#40209,#40210,#40211,#40212,#40213,#40214,
#40215,#40216,#40217),(#40218,#40219,#40220,#40221,#40222,#40223,#40224,
#40225,#40226,#40227,#40228,#40229,#40230,#40231,#40232,#40233,#40234,#40235,
#40236),(#40237,#40238,#40239,#40240,#40241,#40242,#40243,#40244,#40245,
#40246,#40247,#40248,#40249,#40250,#40251,#40252,#40253,#40254,#40255),
(#40256,#40257,#40258,#40259,#40260,#40261,#40262,#40263,#40264,#40265,
#40266,#40267,#40268,#40269,#40270,#40271,#40272,#40273,#40274)),
 .UNSPECIFIED.,.F.,.F.,.F.,(4,4),(4,1,1,1,1,1,1,1,1,1,1,1,1,1,1,1,4),(-0.1077744783079,
1.107774478308),(0.7017764360683,0.7207808788678,0.7397853216674,0.758789764467,
0.7777942072665,0.7967986500661,0.8158030928657,0.8348075356653,0.8538119784648,
0.8728164212644,0.891820864064,0.9108253068635,0.9298297496631,0.9488341924627,
0.9678386352623,0.9868430780618,1.005847520861),.UNSPECIFIED.);
#389=B_SPLINE_SURFACE_WITH_KNOTS('',3,3,((#40368,#40369,#40370,#40371,#40372,
#40373,#40374,#40375,#40376,#40377,#40378,#40379,#40380,#40381,#40382,#40383,
#40384,#40385,#40386),(#40387,#40388,#40389,#40390,#40391,#40392,#40393,
#40394,#40395,#40396,#40397,#40398,#40399,#40400,#40401,#40402,#40403,#40404,
#40405),(#40406,#40407,#40408,#40409,#40410,#40411,#40412,#40413,#40414,
#40415,#40416,#40417,#40418,#40419,#40420,#40421,#40422,#40423,#40424),
(#40425,#40426,#40427,#40428,#40429,#40430,#40431,#40432,#40433,#40434,
#40435,#40436,#40437,#40438,#40439,#40440,#40441,#40442,#40443)),
 .UNSPECIFIED.,.F.,.F.,.F.,(4,4),(4,1,1,1,1,1,1,1,1,1,1,1,1,1,1,1,4),(-0.1077744783079,
1.107774478308),(0.49,0.5225,0.555,0.5875,0.62,0.6525,0.685,0.7175,0.75,
0.7825,0.815,0.8475,0.88,0.9125,0.945,0.9775,1.01),.UNSPECIFIED.);
#390=B_SPLINE_SURFACE_WITH_KNOTS('',3,3,((#40584,#40585,#40586,#40587,#40588,
#40589,#40590,#40591,#40592,#40593,#40594,#40595,#40596,#40597,#40598,#40599,
#40600,#40601,#40602),(#40603,#40604,#40605,#40606,#40607,#40608,#40609,
#40610,#40611,#40612,#40613,#40614,#40615,#40616,#40617,#40618,#40619,#40620,
#40621),(#40622,#40623,#40624,#40625,#40626,#40627,#40628,#40629,#40630,
#40631,#40632,#40633,#40634,#40635,#40636,#40637,#40638,#40639,#40640),
(#40641,#40642,#40643,#40644,#40645,#40646,#40647,#40648,#40649,#40650,
#40651,#40652,#40653,#40654,#40655,#40656,#40657,#40658,#40659)),
 .UNSPECIFIED.,.F.,.F.,.F.,(4,4),(4,1,1,1,1,1,1,1,1,1,1,1,1,1,1,1,4),(-0.1727715412221,
1.172771541222),(0.5842235639317,0.6107191211322,0.6372146783326,0.663710235533,
0.6902057927335,0.7167013499339,0.7431969071343,0.7696924643347,0.7961880215352,
0.8226835787356,0.849179135936,0.8756746931365,0.9021702503369,0.9286658075373,
0.9551613647377,0.9816569219382,1.008152479139),.UNSPECIFIED.);
#391=B_SPLINE_SURFACE_WITH_KNOTS('',3,3,((#40661,#40662,#40663,#40664,#40665,
#40666,#40667,#40668,#40669,#40670,#40671,#40672,#40673,#40674,#40675,#40676,
#40677,#40678,#40679,#40680,#40681,#40682,#40683,#40684,#40685,#40686,#40687,
#40688,#40689,#40690,#40691,#40692,#40693,#40694,#40695),(#40696,#40697,
#40698,#40699,#40700,#40701,#40702,#40703,#40704,#40705,#40706,#40707,#40708,
#40709,#40710,#40711,#40712,#40713,#40714,#40715,#40716,#40717,#40718,#40719,
#40720,#40721,#40722,#40723,#40724,#40725,#40726,#40727,#40728,#40729,#40730),
(#40731,#40732,#40733,#40734,#40735,#40736,#40737,#40738,#40739,#40740,
#40741,#40742,#40743,#40744,#40745,#40746,#40747,#40748,#40749,#40750,#40751,
#40752,#40753,#40754,#40755,#40756,#40757,#40758,#40759,#40760,#40761,#40762,
#40763,#40764,#40765),(#40766,#40767,#40768,#40769,#40770,#40771,#40772,
#40773,#40774,#40775,#40776,#40777,#40778,#40779,#40780,#40781,#40782,#40783,
#40784,#40785,#40786,#40787,#40788,#40789,#40790,#40791,#40792,#40793,#40794,
#40795,#40796,#40797,#40798,#40799,#40800)),.UNSPECIFIED.,.F.,.F.,.F.,(4,
4),(4,1,1,1,1,1,1,1,1,1,1,1,1,1,1,1,1,1,1,1,1,1,1,1,1,1,1,1,1,1,1,1,4),
(-0.1727715412221,1.172771541222),(-0.02,0.0125,0.045,0.0775,0.11,0.1425,
0.175,0.2075,0.24,0.2725,0.305,0.3375,0.37,0.4025,0.435,0.4675,0.5,0.5325,
0.565,0.5975,0.63,0.6625,0.695,0.7275,0.76,0.7925,0.825,0.8575,0.89,0.9225,
0.955,0.9875,1.02),.UNSPECIFIED.);
#392=B_SPLINE_SURFACE_WITH_KNOTS('',3,3,((#41024,#41025,#41026,#41027,#41028,
#41029,#41030,#41031,#41032,#41033,#41034,#41035,#41036,#41037,#41038,#41039,
#41040,#41041,#41042,#41043,#41044,#41045,#41046,#41047,#41048,#41049,#41050,
#41051,#41052,#41053,#41054,#41055,#41056,#41057,#41058),(#41059,#41060,
#41061,#41062,#41063,#41064,#41065,#41066,#41067,#41068,#41069,#41070,#41071,
#41072,#41073,#41074,#41075,#41076,#41077,#41078,#41079,#41080,#41081,#41082,
#41083,#41084,#41085,#41086,#41087,#41088,#41089,#41090,#41091,#41092,#41093),
(#41094,#41095,#41096,#41097,#41098,#41099,#41100,#41101,#41102,#41103,
#41104,#41105,#41106,#41107,#41108,#41109,#41110,#41111,#41112,#41113,#41114,
#41115,#41116,#41117,#41118,#41119,#41120,#41121,#41122,#41123,#41124,#41125,
#41126,#41127,#41128),(#41129,#41130,#41131,#41132,#41133,#41134,#41135,
#41136,#41137,#41138,#41139,#41140,#41141,#41142,#41143,#41144,#41145,#41146,
#41147,#41148,#41149,#41150,#41151,#41152,#41153,#41154,#41155,#41156,#41157,
#41158,#41159,#41160,#41161,#41162,#41163)),.UNSPECIFIED.,.F.,.F.,.F.,(4,
4),(4,1,1,1,1,1,1,1,1,1,1,1,1,1,1,1,1,1,1,1,1,1,1,1,1,1,1,1,1,1,1,1,4),
(-0.1077744783079,1.107774478308),(-0.02,0.0125,0.045,0.0775,0.11,0.1425,
0.175,0.2075,0.24,0.2725,0.305,0.3375,0.37,0.4025,0.435,0.4675,0.5,0.5325,
0.565,0.5975,0.63,0.6625,0.695,0.7275,0.76,0.7925,0.825,0.8575,0.89,0.9225,
0.955,0.9875,1.02),.UNSPECIFIED.);
#393=B_SPLINE_SURFACE_WITH_KNOTS('',3,3,((#41346,#41347,#41348,#41349,#41350,
#41351,#41352,#41353,#41354,#41355,#41356,#41357,#41358,#41359,#41360,#41361,
#41362,#41363,#41364,#41365,#41366,#41367,#41368,#41369,#41370,#41371,#41372,
#41373,#41374,#41375,#41376,#41377,#41378,#41379,#41380),(#41381,#41382,
#41383,#41384,#41385,#41386,#41387,#41388,#41389,#41390,#41391,#41392,#41393,
#41394,#41395,#41396,#41397,#41398,#41399,#41400,#41401,#41402,#41403,#41404,
#41405,#41406,#41407,#41408,#41409,#41410,#41411,#41412,#41413,#41414,#41415),
(#41416,#41417,#41418,#41419,#41420,#41421,#41422,#41423,#41424,#41425,
#41426,#41427,#41428,#41429,#41430,#41431,#41432,#41433,#41434,#41435,#41436,
#41437,#41438,#41439,#41440,#41441,#41442,#41443,#41444,#41445,#41446,#41447,
#41448,#41449,#41450),(#41451,#41452,#41453,#41454,#41455,#41456,#41457,
#41458,#41459,#41460,#41461,#41462,#41463,#41464,#41465,#41466,#41467,#41468,
#41469,#41470,#41471,#41472,#41473,#41474,#41475,#41476,#41477,#41478,#41479,
#41480,#41481,#41482,#41483,#41484,#41485)),.UNSPECIFIED.,.F.,.F.,.F.,(4,
4),(4,1,1,1,1,1,1,1,1,1,1,1,1,1,1,1,1,1,1,1,1,1,1,1,1,1,1,1,1,1,1,1,4),
(-0.1077744783079,1.107774478308),(-0.02,0.0125,0.045,0.0775,0.11,0.1425,
0.175,0.2075,0.24,0.2725,0.305,0.3375,0.37,0.4025,0.435,0.4675,0.5,0.5325,
0.565,0.5975,0.63,0.6625,0.695,0.7275,0.76,0.7925,0.825,0.8575,0.89,0.9225,
0.955,0.9875,1.02),.UNSPECIFIED.);
#394=B_SPLINE_SURFACE_WITH_KNOTS('',3,3,((#41598,#41599,#41600,#41601,#41602,
#41603,#41604,#41605,#41606,#41607,#41608,#41609,#41610,#41611,#41612,#41613,
#41614,#41615,#41616,#41617,#41618,#41619,#41620,#41621,#41622,#41623,#41624,
#41625,#41626,#41627,#41628,#41629,#41630,#41631,#41632),(#41633,#41634,
#41635,#41636,#41637,#41638,#41639,#41640,#41641,#41642,#41643,#41644,#41645,
#41646,#41647,#41648,#41649,#41650,#41651,#41652,#41653,#41654,#41655,#41656,
#41657,#41658,#41659,#41660,#41661,#41662,#41663,#41664,#41665,#41666,#41667),
(#41668,#41669,#41670,#41671,#41672,#41673,#41674,#41675,#41676,#41677,
#41678,#41679,#41680,#41681,#41682,#41683,#41684,#41685,#41686,#41687,#41688,
#41689,#41690,#41691,#41692,#41693,#41694,#41695,#41696,#41697,#41698,#41699,
#41700,#41701,#41702),(#41703,#41704,#41705,#41706,#41707,#41708,#41709,
#41710,#41711,#41712,#41713,#41714,#41715,#41716,#41717,#41718,#41719,#41720,
#41721,#41722,#41723,#41724,#41725,#41726,#41727,#41728,#41729,#41730,#41731,
#41732,#41733,#41734,#41735,#41736,#41737)),.UNSPECIFIED.,.F.,.F.,.F.,(4,
4),(4,1,1,1,1,1,1,1,1,1,1,1,1,1,1,1,1,1,1,1,1,1,1,1,1,1,1,1,1,1,1,1,4),
(-0.1077744783079,1.107774478308),(-0.02,0.0125,0.045,0.0775,0.11,0.1425,
0.175,0.2075,0.24,0.2725,0.305,0.3375,0.37,0.4025,0.435,0.4675,0.5,0.5325,
0.565,0.5975,0.63,0.6625,0.695,0.7275,0.76,0.7925,0.825,0.8575,0.89,0.9225,
0.955,0.9875,1.02),.UNSPECIFIED.);
#395=B_SPLINE_SURFACE_WITH_KNOTS('',3,3,((#42140,#42141,#42142,#42143,#42144,
#42145,#42146,#42147,#42148,#42149,#42150,#42151,#42152,#42153,#42154,#42155,
#42156,#42157,#42158,#42159,#42160,#42161,#42162,#42163,#42164,#42165,#42166,
#42167,#42168,#42169,#42170,#42171,#42172,#42173,#42174),(#42175,#42176,
#42177,#42178,#42179,#42180,#42181,#42182,#42183,#42184,#42185,#42186,#42187,
#42188,#42189,#42190,#42191,#42192,#42193,#42194,#42195,#42196,#42197,#42198,
#42199,#42200,#42201,#42202,#42203,#42204,#42205,#42206,#42207,#42208,#42209),
(#42210,#42211,#42212,#42213,#42214,#42215,#42216,#42217,#42218,#42219,
#42220,#42221,#42222,#42223,#42224,#42225,#42226,#42227,#42228,#42229,#42230,
#42231,#42232,#42233,#42234,#42235,#42236,#42237,#42238,#42239,#42240,#42241,
#42242,#42243,#42244),(#42245,#42246,#42247,#42248,#42249,#42250,#42251,
#42252,#42253,#42254,#42255,#42256,#42257,#42258,#42259,#42260,#42261,#42262,
#42263,#42264,#42265,#42266,#42267,#42268,#42269,#42270,#42271,#42272,#42273,
#42274,#42275,#42276,#42277,#42278,#42279)),.UNSPECIFIED.,.F.,.F.,.F.,(4,
4),(4,1,1,1,1,1,1,1,1,1,1,1,1,1,1,1,1,1,1,1,1,1,1,1,1,1,1,1,1,1,1,1,4),
(-0.1077744783079,1.107774478308),(-0.02,0.0125,0.045,0.0775,0.11,0.1425,
0.175,0.2075,0.24,0.2725,0.305,0.3375,0.37,0.4025,0.435,0.4675,0.5,0.5325,
0.565,0.5975,0.63,0.6625,0.695,0.7275,0.76,0.7925,0.825,0.8575,0.89,0.9225,
0.955,0.9875,1.02),.UNSPECIFIED.);
#396=B_SPLINE_SURFACE_WITH_KNOTS('',3,3,((#42392,#42393,#42394,#42395,#42396,
#42397,#42398,#42399,#42400,#42401,#42402,#42403,#42404,#42405,#42406,#42407,
#42408,#42409,#42410,#42411,#42412,#42413,#42414,#42415,#42416,#42417,#42418,
#42419,#42420,#42421,#42422,#42423,#42424,#42425,#42426),(#42427,#42428,
#42429,#42430,#42431,#42432,#42433,#42434,#42435,#42436,#42437,#42438,#42439,
#42440,#42441,#42442,#42443,#42444,#42445,#42446,#42447,#42448,#42449,#42450,
#42451,#42452,#42453,#42454,#42455,#42456,#42457,#42458,#42459,#42460,#42461),
(#42462,#42463,#42464,#42465,#42466,#42467,#42468,#42469,#42470,#42471,
#42472,#42473,#42474,#42475,#42476,#42477,#42478,#42479,#42480,#42481,#42482,
#42483,#42484,#42485,#42486,#42487,#42488,#42489,#42490,#42491,#42492,#42493,
#42494,#42495,#42496),(#42497,#42498,#42499,#42500,#42501,#42502,#42503,
#42504,#42505,#42506,#42507,#42508,#42509,#42510,#42511,#42512,#42513,#42514,
#42515,#42516,#42517,#42518,#42519,#42520,#42521,#42522,#42523,#42524,#42525,
#42526,#42527,#42528,#42529,#42530,#42531)),.UNSPECIFIED.,.F.,.F.,.F.,(4,
4),(4,1,1,1,1,1,1,1,1,1,1,1,1,1,1,1,1,1,1,1,1,1,1,1,1,1,1,1,1,1,1,1,4),
(-0.1077744783079,1.107774478308),(-0.02,0.0125,0.045,0.0775,0.11,0.1425,
0.175,0.2075,0.24,0.2725,0.305,0.3375,0.37,0.4025,0.435,0.4675,0.5,0.5325,
0.565,0.5975,0.63,0.6625,0.695,0.7275,0.76,0.7925,0.825,0.8575,0.89,0.9225,
0.955,0.9875,1.02),.UNSPECIFIED.);
#397=B_SPLINE_SURFACE_WITH_KNOTS('',3,3,((#42827,#42828,#42829,#42830,#42831,
#42832,#42833,#42834,#42835,#42836,#42837,#42838,#42839,#42840,#42841,#42842,
#42843,#42844,#42845,#42846,#42847,#42848,#42849,#42850,#42851,#42852,#42853,
#42854,#42855,#42856,#42857,#42858,#42859,#42860,#42861),(#42862,#42863,
#42864,#42865,#42866,#42867,#42868,#42869,#42870,#42871,#42872,#42873,#42874,
#42875,#42876,#42877,#42878,#42879,#42880,#42881,#42882,#42883,#42884,#42885,
#42886,#42887,#42888,#42889,#42890,#42891,#42892,#42893,#42894,#42895,#42896),
(#42897,#42898,#42899,#42900,#42901,#42902,#42903,#42904,#42905,#42906,
#42907,#42908,#42909,#42910,#42911,#42912,#42913,#42914,#42915,#42916,#42917,
#42918,#42919,#42920,#42921,#42922,#42923,#42924,#42925,#42926,#42927,#42928,
#42929,#42930,#42931),(#42932,#42933,#42934,#42935,#42936,#42937,#42938,
#42939,#42940,#42941,#42942,#42943,#42944,#42945,#42946,#42947,#42948,#42949,
#42950,#42951,#42952,#42953,#42954,#42955,#42956,#42957,#42958,#42959,#42960,
#42961,#42962,#42963,#42964,#42965,#42966)),.UNSPECIFIED.,.F.,.F.,.F.,(4,
4),(4,1,1,1,1,1,1,1,1,1,1,1,1,1,1,1,1,1,1,1,1,1,1,1,1,1,1,1,1,1,1,1,4),
(-0.1077744783079,1.107774478308),(-0.02,0.0125,0.045,0.0775,0.11,0.1425,
0.175,0.2075,0.24,0.2725,0.305,0.3375,0.37,0.4025,0.435,0.4675,0.5,0.5325,
0.565,0.5975,0.63,0.6625,0.695,0.7275,0.76,0.7925,0.825,0.8575,0.89,0.9225,
0.955,0.9875,1.02),.UNSPECIFIED.);
#398=B_SPLINE_SURFACE_WITH_KNOTS('',3,3,((#43084,#43085,#43086,#43087,#43088,
#43089,#43090,#43091,#43092,#43093,#43094,#43095,#43096,#43097,#43098,#43099,
#43100,#43101,#43102,#43103,#43104,#43105,#43106,#43107,#43108,#43109,#43110,
#43111,#43112,#43113,#43114,#43115,#43116,#43117,#43118),(#43119,#43120,
#43121,#43122,#43123,#43124,#43125,#43126,#43127,#43128,#43129,#43130,#43131,
#43132,#43133,#43134,#43135,#43136,#43137,#43138,#43139,#43140,#43141,#43142,
#43143,#43144,#43145,#43146,#43147,#43148,#43149,#43150,#43151,#43152,#43153),
(#43154,#43155,#43156,#43157,#43158,#43159,#43160,#43161,#43162,#43163,
#43164,#43165,#43166,#43167,#43168,#43169,#43170,#43171,#43172,#43173,#43174,
#43175,#43176,#43177,#43178,#43179,#43180,#43181,#43182,#43183,#43184,#43185,
#43186,#43187,#43188),(#43189,#43190,#43191,#43192,#43193,#43194,#43195,
#43196,#43197,#43198,#43199,#43200,#43201,#43202,#43203,#43204,#43205,#43206,
#43207,#43208,#43209,#43210,#43211,#43212,#43213,#43214,#43215,#43216,#43217,
#43218,#43219,#43220,#43221,#43222,#43223)),.UNSPECIFIED.,.F.,.F.,.F.,(4,
4),(4,1,1,1,1,1,1,1,1,1,1,1,1,1,1,1,1,1,1,1,1,1,1,1,1,1,1,1,1,1,1,1,4),
(-0.1727715412221,1.172771541222),(-0.02,0.0125,0.045,0.0775,0.11,0.1425,
0.175,0.2075,0.24,0.2725,0.305,0.3375,0.37,0.4025,0.435,0.4675,0.5,0.5325,
0.565,0.5975,0.63,0.6625,0.695,0.7275,0.76,0.7925,0.825,0.8575,0.89,0.9225,
0.955,0.9875,1.02),.UNSPECIFIED.);
#399=B_SPLINE_SURFACE_WITH_KNOTS('',3,3,((#43231,#43232,#43233,#43234,#43235,
#43236,#43237,#43238,#43239,#43240,#43241,#43242,#43243,#43244,#43245,#43246,
#43247,#43248,#43249,#43250,#43251,#43252,#43253,#43254,#43255,#43256,#43257,
#43258,#43259,#43260,#43261,#43262,#43263,#43264,#43265),(#43266,#43267,
#43268,#43269,#43270,#43271,#43272,#43273,#43274,#43275,#43276,#43277,#43278,
#43279,#43280,#43281,#43282,#43283,#43284,#43285,#43286,#43287,#43288,#43289,
#43290,#43291,#43292,#43293,#43294,#43295,#43296,#43297,#43298,#43299,#43300),
(#43301,#43302,#43303,#43304,#43305,#43306,#43307,#43308,#43309,#43310,
#43311,#43312,#43313,#43314,#43315,#43316,#43317,#43318,#43319,#43320,#43321,
#43322,#43323,#43324,#43325,#43326,#43327,#43328,#43329,#43330,#43331,#43332,
#43333,#43334,#43335),(#43336,#43337,#43338,#43339,#43340,#43341,#43342,
#43343,#43344,#43345,#43346,#43347,#43348,#43349,#43350,#43351,#43352,#43353,
#43354,#43355,#43356,#43357,#43358,#43359,#43360,#43361,#43362,#43363,#43364,
#43365,#43366,#43367,#43368,#43369,#43370)),.UNSPECIFIED.,.F.,.F.,.F.,(4,
4),(4,1,1,1,1,1,1,1,1,1,1,1,1,1,1,1,1,1,1,1,1,1,1,1,1,1,1,1,1,1,1,1,4),
(-0.1727715412221,1.172771541222),(-0.02,0.0125,0.045,0.0775,0.11,0.1425,
0.175,0.2075,0.24,0.2725,0.305,0.3375,0.37,0.4025,0.435,0.4675,0.5,0.5325,
0.565,0.5975,0.63,0.6625,0.695,0.7275,0.76,0.7925,0.825,0.8575,0.89,0.9225,
0.955,0.9875,1.02),.UNSPECIFIED.);
#484=PLANE('',#9988);
#485=PLANE('',#9997);
#486=PLANE('',#10004);
#487=PLANE('',#10005);
#488=PLANE('',#10006);
#489=PLANE('',#10010);
#490=PLANE('',#10014);
#491=PLANE('',#10023);
#492=PLANE('',#10041);
#493=PLANE('',#10052);
#494=PLANE('',#10067);
#495=PLANE('',#10086);
#496=PLANE('',#10091);
#497=PLANE('',#10095);
#498=PLANE('',#10100);
#499=PLANE('',#10101);
#500=PLANE('',#10107);
#501=PLANE('',#10114);
#502=PLANE('',#10118);
#923=FACE_OUTER_BOUND('',#1476,.T.);
#924=FACE_OUTER_BOUND('',#1478,.T.);
#925=FACE_OUTER_BOUND('',#1479,.T.);
#926=FACE_OUTER_BOUND('',#1480,.T.);
#927=FACE_OUTER_BOUND('',#1482,.T.);
#928=FACE_OUTER_BOUND('',#1483,.T.);
#929=FACE_OUTER_BOUND('',#1484,.T.);
#930=FACE_OUTER_BOUND('',#1485,.T.);
#931=FACE_OUTER_BOUND('',#1486,.T.);
#932=FACE_OUTER_BOUND('',#1487,.T.);
#933=FACE_OUTER_BOUND('',#1488,.T.);
#934=FACE_OUTER_BOUND('',#1489,.T.);
#935=FACE_OUTER_BOUND('',#1490,.T.);
#936=FACE_OUTER_BOUND('',#1491,.T.);
#937=FACE_OUTER_BOUND('',#1492,.T.);
#938=FACE_OUTER_BOUND('',#1493,.T.);
#939=FACE_OUTER_BOUND('',#1494,.T.);
#940=FACE_OUTER_BOUND('',#1495,.T.);
#941=FACE_OUTER_BOUND('',#1496,.T.);
#942=FACE_OUTER_BOUND('',#1497,.T.);
#943=FACE_OUTER_BOUND('',#1498,.T.);
#944=FACE_OUTER_BOUND('',#1500,.T.);
#945=FACE_OUTER_BOUND('',#1502,.T.);
#946=FACE_OUTER_BOUND('',#1504,.T.);
#947=FACE_OUTER_BOUND('',#1505,.T.);
#948=FACE_OUTER_BOUND('',#1508,.T.);
#949=FACE_OUTER_BOUND('',#1509,.T.);
#950=FACE_OUTER_BOUND('',#1511,.T.);
#951=FACE_OUTER_BOUND('',#1512,.T.);
#952=FACE_OUTER_BOUND('',#1513,.T.);
#953=FACE_OUTER_BOUND('',#1514,.T.);
#954=FACE_OUTER_BOUND('',#1515,.T.);
#955=FACE_OUTER_BOUND('',#1516,.T.);
#956=FACE_OUTER_BOUND('',#1517,.T.);
#957=FACE_OUTER_BOUND('',#1518,.T.);
#958=FACE_OUTER_BOUND('',#1519,.T.);
#959=FACE_OUTER_BOUND('',#1520,.T.);
#960=FACE_OUTER_BOUND('',#1521,.T.);
#961=FACE_OUTER_BOUND('',#1522,.T.);
#962=FACE_OUTER_BOUND('',#1523,.T.);
#963=FACE_OUTER_BOUND('',#1524,.T.);
#964=FACE_OUTER_BOUND('',#1525,.T.);
#965=FACE_OUTER_BOUND('',#1526,.T.);
#966=FACE_OUTER_BOUND('',#1527,.T.);
#967=FACE_OUTER_BOUND('',#1528,.T.);
#968=FACE_OUTER_BOUND('',#1529,.T.);
#969=FACE_OUTER_BOUND('',#1530,.T.);
#970=FACE_OUTER_BOUND('',#1531,.T.);
#971=FACE_OUTER_BOUND('',#1532,.T.);
#972=FACE_OUTER_BOUND('',#1533,.T.);
#973=FACE_OUTER_BOUND('',#1534,.T.);
#974=FACE_OUTER_BOUND('',#1535,.T.);
#975=FACE_OUTER_BOUND('',#1536,.T.);
#976=FACE_OUTER_BOUND('',#1537,.T.);
#977=FACE_OUTER_BOUND('',#1538,.T.);
#978=FACE_OUTER_BOUND('',#1539,.T.);
#979=FACE_OUTER_BOUND('',#1540,.T.);
#980=FACE_OUTER_BOUND('',#1541,.T.);
#981=FACE_OUTER_BOUND('',#1542,.T.);
#982=FACE_OUTER_BOUND('',#1543,.T.);
#983=FACE_OUTER_BOUND('',#1544,.T.);
#984=FACE_OUTER_BOUND('',#1546,.T.);
#985=FACE_OUTER_BOUND('',#1547,.T.);
#986=FACE_OUTER_BOUND('',#1549,.T.);
#987=FACE_OUTER_BOUND('',#1550,.T.);
#988=FACE_OUTER_BOUND('',#1552,.T.);
#989=FACE_OUTER_BOUND('',#1553,.T.);
#990=FACE_OUTER_BOUND('',#1554,.T.);
#991=FACE_OUTER_BOUND('',#1555,.T.);
#992=FACE_OUTER_BOUND('',#1556,.T.);
#993=FACE_OUTER_BOUND('',#1557,.T.);
#994=FACE_OUTER_BOUND('',#1558,.T.);
#995=FACE_OUTER_BOUND('',#1559,.T.);
#996=FACE_OUTER_BOUND('',#1560,.T.);
#997=FACE_OUTER_BOUND('',#1561,.T.);
#998=FACE_OUTER_BOUND('',#1562,.T.);
#999=FACE_OUTER_BOUND('',#1563,.T.);
#1000=FACE_OUTER_BOUND('',#1564,.T.);
#1001=FACE_OUTER_BOUND('',#1565,.T.);
#1002=FACE_OUTER_BOUND('',#1566,.T.);
#1003=FACE_OUTER_BOUND('',#1567,.T.);
#1004=FACE_OUTER_BOUND('',#1568,.T.);
#1005=FACE_OUTER_BOUND('',#1569,.T.);
#1006=FACE_OUTER_BOUND('',#1570,.T.);
#1007=FACE_OUTER_BOUND('',#1571,.T.);
#1008=FACE_OUTER_BOUND('',#1572,.T.);
#1009=FACE_OUTER_BOUND('',#1573,.T.);
#1010=FACE_OUTER_BOUND('',#1574,.T.);
#1011=FACE_OUTER_BOUND('',#1575,.T.);
#1012=FACE_OUTER_BOUND('',#1576,.T.);
#1476=EDGE_LOOP('',(#7732,#7733,#7734,#7735,#7736,#7737));
#1477=EDGE_LOOP('',(#7738));
#1478=EDGE_LOOP('',(#7739,#7740,#7741,#7742,#7743));
#1479=EDGE_LOOP('',(#7744,#7745,#7746,#7747,#7748));
#1480=EDGE_LOOP('',(#7749));
#1481=EDGE_LOOP('',(#7750));
#1482=EDGE_LOOP('',(#7751,#7752,#7753,#7754,#7755));
#1483=EDGE_LOOP('',(#7756,#7757,#7758,#7759,#7760,#7761));
#1484=EDGE_LOOP('',(#7762,#7763,#7764,#7765,#7766));
#1485=EDGE_LOOP('',(#7767,#7768,#7769,#7770,#7771,#7772));
#1486=EDGE_LOOP('',(#7773,#7774,#7775,#7776,#7777,#7778,#7779,#7780));
#1487=EDGE_LOOP('',(#7781,#7782,#7783,#7784));
#1488=EDGE_LOOP('',(#7785,#7786,#7787,#7788));
#1489=EDGE_LOOP('',(#7789,#7790,#7791,#7792,#7793,#7794));
#1490=EDGE_LOOP('',(#7795,#7796,#7797,#7798,#7799));
#1491=EDGE_LOOP('',(#7800,#7801,#7802,#7803,#7804));
#1492=EDGE_LOOP('',(#7805,#7806,#7807,#7808,#7809));
#1493=EDGE_LOOP('',(#7810,#7811,#7812,#7813,#7814));
#1494=EDGE_LOOP('',(#7815,#7816,#7817,#7818,#7819,#7820));
#1495=EDGE_LOOP('',(#7821,#7822,#7823,#7824));
#1496=EDGE_LOOP('',(#7825,#7826,#7827,#7828));
#1497=EDGE_LOOP('',(#7829,#7830,#7831,#7832));
#1498=EDGE_LOOP('',(#7833));
#1499=EDGE_LOOP('',(#7834));
#1500=EDGE_LOOP('',(#7835,#7836,#7837,#7838));
#1501=EDGE_LOOP('',(#7839,#7840));
#1502=EDGE_LOOP('',(#7841));
#1503=EDGE_LOOP('',(#7842));
#1504=EDGE_LOOP('',(#7843,#7844,#7845,#7846));
#1505=EDGE_LOOP('',(#7847,#7848,#7849,#7850,#7851,#7852,#7853,#7854,#7855,
#7856,#7857,#7858,#7859,#7860,#7861));
#1506=EDGE_LOOP('',(#7862));
#1507=EDGE_LOOP('',(#7863));
#1508=EDGE_LOOP('',(#7864,#7865,#7866,#7867));
#1509=EDGE_LOOP('',(#7868,#7869,#7870,#7871));
#1510=EDGE_LOOP('',(#7872));
#1511=EDGE_LOOP('',(#7873,#7874,#7875,#7876));
#1512=EDGE_LOOP('',(#7877,#7878,#7879,#7880));
#1513=EDGE_LOOP('',(#7881,#7882,#7883,#7884));
#1514=EDGE_LOOP('',(#7885,#7886,#7887,#7888));
#1515=EDGE_LOOP('',(#7889,#7890,#7891,#7892));
#1516=EDGE_LOOP('',(#7893,#7894,#7895,#7896));
#1517=EDGE_LOOP('',(#7897,#7898,#7899,#7900));
#1518=EDGE_LOOP('',(#7901,#7902,#7903,#7904));
#1519=EDGE_LOOP('',(#7905,#7906,#7907,#7908));
#1520=EDGE_LOOP('',(#7909,#7910,#7911,#7912));
#1521=EDGE_LOOP('',(#7913,#7914,#7915,#7916));
#1522=EDGE_LOOP('',(#7917,#7918,#7919,#7920));
#1523=EDGE_LOOP('',(#7921,#7922,#7923,#7924));
#1524=EDGE_LOOP('',(#7925,#7926,#7927,#7928));
#1525=EDGE_LOOP('',(#7929,#7930,#7931,#7932));
#1526=EDGE_LOOP('',(#7933,#7934,#7935,#7936));
#1527=EDGE_LOOP('',(#7937,#7938,#7939,#7940));
#1528=EDGE_LOOP('',(#7941,#7942,#7943,#7944,#7945,#7946,#7947,#7948,#7949,
#7950));
#1529=EDGE_LOOP('',(#7951,#7952,#7953,#7954));
#1530=EDGE_LOOP('',(#7955,#7956,#7957,#7958));
#1531=EDGE_LOOP('',(#7959,#7960,#7961,#7962,#7963,#7964));
#1532=EDGE_LOOP('',(#7965,#7966,#7967,#7968,#7969));
#1533=EDGE_LOOP('',(#7970,#7971,#7972,#7973,#7974));
#1534=EDGE_LOOP('',(#7975,#7976,#7977,#7978));
#1535=EDGE_LOOP('',(#7979,#7980,#7981,#7982));
#1536=EDGE_LOOP('',(#7983,#7984,#7985,#7986,#7987,#7988,#7989,#7990));
#1537=EDGE_LOOP('',(#7991,#7992,#7993));
#1538=EDGE_LOOP('',(#7994,#7995,#7996,#7997));
#1539=EDGE_LOOP('',(#7998,#7999,#8000,#8001));
#1540=EDGE_LOOP('',(#8002,#8003,#8004,#8005,#8006,#8007));
#1541=EDGE_LOOP('',(#8008,#8009,#8010,#8011));
#1542=EDGE_LOOP('',(#8012,#8013,#8014,#8015));
#1543=EDGE_LOOP('',(#8016,#8017,#8018,#8019));
#1544=EDGE_LOOP('',(#8020,#8021,#8022,#8023,#8024,#8025));
#1545=EDGE_LOOP('',(#8026));
#1546=EDGE_LOOP('',(#8027,#8028,#8029,#8030));
#1547=EDGE_LOOP('',(#8031));
#1548=EDGE_LOOP('',(#8032));
#1549=EDGE_LOOP('',(#8033,#8034,#8035,#8036,#8037,#8038,#8039,#8040));
#1550=EDGE_LOOP('',(#8041,#8042,#8043,#8044,#8045,#8046,#8047,#8048));
#1551=EDGE_LOOP('',(#8049));
#1552=EDGE_LOOP('',(#8050,#8051,#8052,#8053));
#1553=EDGE_LOOP('',(#8054,#8055,#8056,#8057,#8058,#8059));
#1554=EDGE_LOOP('',(#8060,#8061,#8062,#8063));
#1555=EDGE_LOOP('',(#8064,#8065,#8066,#8067));
#1556=EDGE_LOOP('',(#8068,#8069,#8070,#8071,#8072));
#1557=EDGE_LOOP('',(#8073,#8074,#8075,#8076,#8077));
#1558=EDGE_LOOP('',(#8078,#8079,#8080,#8081,#8082,#8083));
#1559=EDGE_LOOP('',(#8084,#8085,#8086,#8087));
#1560=EDGE_LOOP('',(#8088,#8089,#8090,#8091));
#1561=EDGE_LOOP('',(#8092,#8093,#8094,#8095));
#1562=EDGE_LOOP('',(#8096,#8097,#8098,#8099));
#1563=EDGE_LOOP('',(#8100,#8101,#8102,#8103));
#1564=EDGE_LOOP('',(#8104,#8105,#8106,#8107));
#1565=EDGE_LOOP('',(#8108,#8109,#8110,#8111));
#1566=EDGE_LOOP('',(#8112,#8113,#8114));
#1567=EDGE_LOOP('',(#8115,#8116,#8117,#8118));
#1568=EDGE_LOOP('',(#8119,#8120,#8121,#8122,#8123,#8124,#8125));
#1569=EDGE_LOOP('',(#8126,#8127,#8128,#8129));
#1570=EDGE_LOOP('',(#8130,#8131,#8132,#8133));
#1571=EDGE_LOOP('',(#8134,#8135,#8136,#8137));
#1572=EDGE_LOOP('',(#8138,#8139,#8140,#8141));
#1573=EDGE_LOOP('',(#8142,#8143,#8144,#8145));
#1574=EDGE_LOOP('',(#8146,#8147,#8148,#8149));
#1575=EDGE_LOOP('',(#8150,#8151,#8152,#8153));
#1576=EDGE_LOOP('',(#8154,#8155,#8156,#8157));
#1993=CIRCLE('',#9989,7.5);
#1994=CIRCLE('',#9990,6.);
#1995=CIRCLE('',#9992,5.);
#1996=CIRCLE('',#9993,5.);
#1997=CIRCLE('',#9994,1.);
#1998=CIRCLE('',#9996,5.);
#1999=CIRCLE('',#9998,4.);
#2000=CIRCLE('',#10000,4.);
#2001=CIRCLE('',#10001,4.);
#2002=CIRCLE('',#10003,4.);
#2003=CIRCLE('',#10007,6.);
#2004=CIRCLE('',#10009,6.);
#2005=CIRCLE('',#10011,6.75);
#2006=CIRCLE('',#10013,6.75);
#2007=CIRCLE('',#10015,7.5);
#2008=CIRCLE('',#10016,1.5);
#2009=CIRCLE('',#10017,2.5);
#2010=CIRCLE('',#10018,1.5);
#2011=CIRCLE('',#10019,7.5);
#2012=CIRCLE('',#10020,1.25);
#2013=CIRCLE('',#10022,1.25);
#2014=CIRCLE('',#10024,9.);
#2015=CIRCLE('',#10025,2.5);
#2016=CIRCLE('',#10027,0.5);
#2017=CIRCLE('',#10028,1.);
#2018=CIRCLE('',#10029,1.);
#2019=CIRCLE('',#10031,1.);
#2020=CIRCLE('',#10032,8.);
#2021=CIRCLE('',#10033,1.);
#2022=CIRCLE('',#10035,1.);
#2023=CIRCLE('',#10037,0.5);
#2024=CIRCLE('',#10038,0.5);
#2025=CIRCLE('',#10040,0.5);
#2026=CIRCLE('',#10043,0.5);
#2027=CIRCLE('',#10045,3.);
#2028=CIRCLE('',#10047,3.);
#2029=CIRCLE('',#10049,0.5);
#2030=CIRCLE('',#10051,0.5);
#2031=CIRCLE('',#10054,1.);
#2032=CIRCLE('',#10056,0.5);
#2033=CIRCLE('',#10058,8.);
#2034=CIRCLE('',#10059,0.5);
#2035=CIRCLE('',#10061,8.);
#2036=CIRCLE('',#10062,8.);
#2037=CIRCLE('',#10064,0.5);
#2038=CIRCLE('',#10066,0.5);
#2039=CIRCLE('',#10068,1.);
#2040=CIRCLE('',#10072,0.5);
#2041=CIRCLE('',#10073,0.4999999959631);
#2042=CIRCLE('',#10076,0.9999999999978);
#2043=CIRCLE('',#10077,0.5000000000709);
#2044=CIRCLE('',#10078,0.5);
#2045=CIRCLE('',#10079,1.);
#2046=CIRCLE('',#10080,0.5000000000042);
#2047=CIRCLE('',#10082,1.);
#2048=CIRCLE('',#10083,0.5);
#2049=CIRCLE('',#10084,0.5);
#2050=CIRCLE('',#10085,0.5);
#2051=CIRCLE('',#10087,2.5);
#2052=CIRCLE('',#10088,3.6);
#2053=CIRCLE('',#10090,3.6);
#2054=CIRCLE('',#10092,3.23);
#2055=CIRCLE('',#10094,3.23);
#2056=CIRCLE('',#10103,1.);
#2057=CIRCLE('',#10105,0.50000015263);
#2058=CIRCLE('',#10113,0.5000000000013);
#2059=CIRCLE('',#10116,0.5000003490389);
#2060=CIRCLE('',#10117,0.5000000000992);
#2061=CIRCLE('',#10120,0.5);
#2062=CIRCLE('',#10122,3.);
#2063=CIRCLE('',#10123,0.5);
#2064=CIRCLE('',#10125,0.5);
#2065=CIRCLE('',#10127,0.5);
#2368=B_SPLINE_CURVE_WITH_KNOTS('',3,(#39908,#39909,#39910,#39911,#39912,
#39913,#39914,#39915,#39916,#39917,#39918),.UNSPECIFIED.,.F.,.F.,(4,1,1,
1,1,1,1,1,4),(1.74506463504632E-7,0.125,0.25,0.375,0.5,0.625,0.75,0.875,
1.),.UNSPECIFIED.);
#2369=B_SPLINE_CURVE_WITH_KNOTS('',3,(#39949,#39950,#39951,#39952,#39953,
#39954,#39955,#39956,#39957,#39958,#39959,#39960,#39961,#39962,#39963,#39964,
#39965,#39966,#39967,#39968),.UNSPECIFIED.,.F.,.F.,(4,2,2,2,2,2,2,2,2,4),
(-0.419307317134397,-0.376446924920619,-0.33249018087809,-0.280553953647668,
-0.23721700391194,-0.211165835567419,-0.176188829306431,-0.103876860558225,
-0.0598885228554427,-7.92473299855586E-5),.UNSPECIFIED.);
#2370=B_SPLINE_CURVE_WITH_KNOTS('',3,(#39971,#39972,#39973,#39974,#39975,
#39976,#39977,#39978,#39979,#39980,#39981,#39982,#39983,#39984,#39985,#39986,
#39987,#39988,#39989,#39990,#39991,#39992,#39993,#39994,#39995,#39996,#39997,
#39998,#39999,#40000,#40001,#40002,#40003,#40004,#40005,#40006,#40007,#40008,
#40009,#40010,#40011,#40012,#40013,#40014,#40015,#40016,#40017,#40018,#40019,
#40020,#40021,#40022,#40023,#40024,#40025,#40026,#40027,#40028,#40029,#40030,
#40031,#40032,#40033,#40034,#40035,#40036,#40037,#40038,#40039,#40040,#40041,
#40042,#40043,#40044,#40045,#40046,#40047,#40048,#40049,#40050,#40051,#40052,
#40053,#40054,#40055,#40056,#40057,#40058,#40059,#40060,#40061,#40062,#40063,
#40064),.UNSPECIFIED.,.F.,.F.,(4,2,2,2,2,2,2,2,2,2,2,2,2,2,2,2,2,2,2,2,
2,2,2,2,2,2,2,2,2,2,2,2,2,2,2,2,2,2,2,2,2,2,2,2,2,2,4),(-2.51522491911469,
-2.43371628670848,-2.40614105864553,-2.35503484951906,-2.3067707648452,
-2.26453305057241,-2.20227928383436,-2.16148265557214,-2.13390997902887,
-2.08957850490265,-2.03646371047655,-1.9919948120233,-1.92062186138243,
-1.88521373290542,-1.85899856608694,-1.81624253543225,-1.76404253816429,
-1.72004994921576,-1.64679859763786,-1.61217885105375,-1.58623349108635,
-1.5444488533066,-1.49182130376262,-1.44768968772001,-1.37404101789524,
-1.33957277358892,-1.31365851369137,-1.25749939461323,-1.19246119704988,
-1.14800016017443,-1.09411985945728,-1.05158498284418,-1.02338208188437,
-0.98085216957734,-0.921983788777027,-0.878231883102996,-0.827079325501673,
-0.7819718511449,-0.755826821261395,-0.720496555599507,-0.649110885847386,
-0.60522036792117,-0.553537634951159,-0.509637222343958,-0.483557930911433,
-0.448474158791355,-0.419307317134397),.UNSPECIFIED.);
#2371=B_SPLINE_CURVE_WITH_KNOTS('',3,(#40067,#40068,#40069,#40070,#40071,
#40072,#40073,#40074,#40075,#40076,#40077,#40078,#40079,#40080),
 .UNSPECIFIED.,.F.,.F.,(4,2,2,2,2,2,4),(0.000102940691851845,0.105922775754071,
0.210135463685387,0.343012105338019,0.449458054020239,0.527761272578075,
0.61650116285291),.UNSPECIFIED.);
#2372=B_SPLINE_CURVE_WITH_KNOTS('',3,(#40082,#40083,#40084,#40085,#40086,
#40087,#40088,#40089,#40090,#40091,#40092,#40093,#40094,#40095),
 .UNSPECIFIED.,.F.,.F.,(4,2,2,2,2,2,4),(5.24774905396007E-5,0.102919223275153,
0.200207974164601,0.331136583215735,0.463939911457513,0.553292170439522,
0.637797491354806),.UNSPECIFIED.);
#2373=B_SPLINE_CURVE_WITH_KNOTS('',3,(#40096,#40097,#40098,#40099,#40100,
#40101,#40102,#40103,#40104,#40105,#40106,#40107,#40108,#40109,#40110,#40111,
#40112,#40113,#40114,#40115,#40116,#40117,#40118,#40119,#40120,#40121,#40122,
#40123,#40124,#40125,#40126,#40127,#40128,#40129,#40130,#40131,#40132,#40133,
#40134,#40135,#40136,#40137,#40138,#40139,#40140,#40141,#40142,#40143,#40144,
#40145,#40146,#40147,#40148,#40149,#40150,#40151,#40152,#40153,#40154,#40155,
#40156,#40157,#40158,#40159,#40160,#40161,#40162,#40163,#40164,#40165,#40166,
#40167,#40168,#40169,#40170,#40171,#40172,#40173,#40174,#40175,#40176,#40177,
#40178,#40179,#40180,#40181,#40182,#40183,#40184,#40185,#40186,#40187,#40188,
#40189,#40190,#40191,#40192,#40193,#40194,#40195,#40196,#40197,#40198),
 .UNSPECIFIED.,.F.,.F.,(4,3,3,3,3,3,3,3,3,3,3,3,3,3,3,3,3,3,3,3,3,3,3,3,
3,3,3,3,3,3,3,3,3,3,4),(2.32323281300321E-5,0.0263338187849373,0.0528930048012295,
0.0775527614301843,0.119264862169425,0.151532031317049,0.178160167750092,
0.208545348730825,0.230146401786176,0.259521454361925,0.289979534064853,
0.307566150720886,0.338352589115474,0.370211365474543,0.381353773173637,
0.401064064510986,0.443757841669673,0.487322691796688,0.518553003926838,
0.542684984551173,0.578781121546917,0.611023690584681,0.626943865232523,
0.66435333949954,0.690413260713517,0.720854398171208,0.762829179862876,
0.796341399568512,0.840816408102127,0.873251888090859,0.904910640783385,
0.922121378589668,0.946130264709519,0.973008581785241,0.999886898860964),
 .UNSPECIFIED.);
#2374=B_SPLINE_CURVE_WITH_KNOTS('',3,(#40276,#40277,#40278,#40279,#40280,
#40281,#40282,#40283,#40284,#40285,#40286,#40287,#40288,#40289,#40290,#40291,
#40292,#40293,#40294,#40295,#40296,#40297,#40298,#40299,#40300,#40301,#40302,
#40303,#40304,#40305,#40306,#40307,#40308,#40309,#40310,#40311,#40312,#40313,
#40314,#40315,#40316,#40317,#40318,#40319,#40320,#40321,#40322,#40323,#40324,
#40325),.UNSPECIFIED.,.F.,.F.,(4,2,2,2,2,2,2,2,2,2,2,2,2,2,2,2,2,2,2,2,
2,2,2,2,4),(-0.971724970861776,-0.96224259779374,-0.952818323332198,-0.933893341089848,
-0.921462843293419,-0.89460619776171,-0.871724738068697,-0.85365992165184,
-0.81998862327022,-0.787153942616391,-0.779148549923685,-0.744697301863035,
-0.701771598759441,-0.687301558135749,-0.628830738460491,-0.599891230916682,
-0.570631735013558,-0.517566468648308,-0.458469083445789,-0.384209139007974,
-0.330398146101072,-0.213378846484283,-0.160737820237478,-0.0805171288285796,
-0.00012725556241822),.UNSPECIFIED.);
#2375=B_SPLINE_CURVE_WITH_KNOTS('',3,(#40329,#40330,#40331,#40332,#40333,
#40334,#40335,#40336),.UNSPECIFIED.,.F.,.F.,(4,2,2,4),(-0.209975020768575,
-0.157314244107572,-0.104768532932063,-0.000184589268263047),
 .UNSPECIFIED.);
#2376=B_SPLINE_CURVE_WITH_KNOTS('',3,(#40338,#40339,#40340,#40341,#40342,
#40343,#40344,#40345,#40346,#40347,#40348,#40349,#40350,#40351,#40352,#40353,
#40354,#40355,#40356,#40357,#40358,#40359,#40360,#40361),.UNSPECIFIED.,
 .F.,.F.,(4,2,2,2,2,2,2,2,2,2,2,4),(-1.20838688604733,-1.02839026997692,
-0.883923566776128,-0.809599158177502,-0.752742598652501,-0.622907067493251,
-0.544861408462318,-0.469857238864126,-0.380271098777597,-0.22441099221183,
-0.11473204145142,-6.43510293987729E-5),.UNSPECIFIED.);
#2377=B_SPLINE_CURVE_WITH_KNOTS('',3,(#40362,#40363,#40364,#40365,#40366,
#40367),.UNSPECIFIED.,.F.,.F.,(4,2,4),(-0.210251406797625,-0.104231041931576,
-2.34000127149505E-5),.UNSPECIFIED.);
#2378=B_SPLINE_CURVE_WITH_KNOTS('',3,(#40445,#40446,#40447,#40448,#40449,
#40450,#40451,#40452,#40453,#40454,#40455,#40456,#40457,#40458,#40459,#40460,
#40461,#40462,#40463,#40464,#40465,#40466,#40467,#40468,#40469,#40470,#40471,
#40472),.UNSPECIFIED.,.F.,.F.,(4,2,2,2,2,2,2,2,2,2,2,2,2,4),(0.000185064574131046,
0.0602712190498164,0.0995806517125012,0.155361344960956,0.243764972296806,
0.328938012928217,0.44400330868783,0.523479738663989,0.636194951156639,
0.696271818136377,0.798069126561032,0.914768324732951,0.968509100593359,
1.0452089632934),.UNSPECIFIED.);
#2379=B_SPLINE_CURVE_WITH_KNOTS('',3,(#40474,#40475,#40476,#40477,#40478,
#40479,#40480,#40481,#40482,#40483,#40484,#40485,#40486,#40487,#40488,#40489,
#40490,#40491,#40492,#40493,#40494,#40495,#40496,#40497,#40498,#40499,#40500,
#40501,#40502,#40503,#40504,#40505,#40506,#40507,#40508,#40509,#40510,#40511),
 .UNSPECIFIED.,.F.,.F.,(4,2,2,2,2,2,2,2,2,2,2,2,2,2,2,2,2,2,4),(9.99999997513407E-7,
0.0303667674586334,0.141492987035643,0.19944954580558,0.303623465621176,
0.412366612058417,0.464341609383842,0.616716522689497,0.679112215291004,
0.7325047929673,0.817077506721457,0.960667112020537,1.01645812460288,1.07615291575373,
1.20142634084652,1.23728397080356,1.29083685108454,1.35242730915233,1.46720649961044),
 .UNSPECIFIED.);
#2380=B_SPLINE_CURVE_WITH_KNOTS('',3,(#40514,#40515,#40516,#40517,#40518,
#40519,#40520,#40521,#40522,#40523,#40524,#40525,#40526,#40527,#40528,#40529,
#40530,#40531,#40532,#40533,#40534,#40535,#40536,#40537,#40538,#40539,#40540,
#40541,#40542,#40543,#40544,#40545,#40546,#40547,#40548,#40549,#40550,#40551,
#40552,#40553,#40554,#40555,#40556,#40557,#40558,#40559,#40560,#40561,#40562,
#40563,#40564,#40565,#40566,#40567,#40568,#40569,#40570,#40571,#40572,#40573,
#40574,#40575,#40576,#40577,#40578,#40579,#40580,#40581,#40582,#40583),
 .UNSPECIFIED.,.F.,.F.,(4,2,2,2,2,2,2,2,2,2,2,2,2,2,2,2,2,2,2,2,2,2,2,2,
2,2,2,2,2,2,2,2,2,2,4),(0.000157510224987102,0.0993438493857167,0.188679914346204,
0.251784653428834,0.325862121808707,0.396147813640377,0.465938047156506,
0.526407126825593,0.693172362540282,0.884298387388191,1.03992644234621,
1.1210001397561,1.26371285847868,1.34200253030502,1.42337789123169,1.50196743316852,
1.66711606180234,1.73823621187051,1.81027162284586,1.89143678561552,1.97120519965067,
2.08594346219961,2.16818425450836,2.37346759844623,2.53001217453886,2.68063586602847,
2.89513436904536,3.28430649623881,3.51460467191784,4.14852019298852,4.82236598808902,
5.27439622507704,5.66498526255755,6.25935444338318,6.85318641309348),
 .UNSPECIFIED.);
#2381=B_SPLINE_CURVE_WITH_KNOTS('',3,(#40802,#40803,#40804,#40805,#40806,
#40807,#40808,#40809,#40810,#40811,#40812,#40813,#40814,#40815,#40816,#40817,
#40818,#40819,#40820,#40821,#40822,#40823,#40824,#40825,#40826,#40827,#40828,
#40829,#40830,#40831,#40832,#40833,#40834,#40835,#40836,#40837,#40838,#40839,
#40840,#40841,#40842,#40843,#40844,#40845,#40846,#40847,#40848,#40849,#40850,
#40851,#40852,#40853,#40854,#40855,#40856,#40857,#40858,#40859,#40860,#40861,
#40862,#40863,#40864,#40865,#40866,#40867,#40868,#40869,#40870,#40871,#40872,
#40873,#40874,#40875,#40876,#40877,#40878,#40879,#40880,#40881,#40882,#40883,
#40884,#40885,#40886,#40887,#40888,#40889,#40890,#40891,#40892,#40893,#40894,
#40895,#40896,#40897,#40898,#40899,#40900,#40901,#40902,#40903,#40904,#40905,
#40906,#40907,#40908,#40909,#40910,#40911),.UNSPECIFIED.,.F.,.F.,(4,2,2,
2,2,2,2,2,2,2,2,2,2,2,2,2,2,2,2,2,2,2,2,2,2,2,2,2,2,2,2,2,2,2,2,2,2,2,2,
2,2,2,2,2,2,2,2,2,2,2,2,2,2,2,4),(0.000129114132454983,0.113390093891427,
0.218435321804352,0.324979934352919,0.428164360055101,0.552137859304061,
0.695073909918494,0.846441157571017,0.970455720707209,1.07899479568917,
1.18909049989486,1.29569784196736,1.42371115790198,1.57122215461547,1.72750515786628,
1.85545991638375,1.9674643599747,2.08103983160671,2.1910360991499,2.32304792646442,
2.47507422104983,2.63622907694774,2.76807562998618,2.88350978283409,3.00052157323439,
3.11386868051087,3.24982151808213,3.40628388628472,3.5627462544873,3.69869909205856,
3.81204619933504,3.92905798973533,4.04449214258324,4.17633869562168,4.3374935515196,
4.48951984610501,4.62153167341952,4.73152794096275,4.84510341259479,4.95710785618572,
5.08506261470318,5.24134561795402,5.38885661466752,5.51686993060214,5.62347727267468,
5.7335729768804,5.84211205186234,5.96612661499854,6.11749386265112,6.26042991326557,
6.38440341251452,6.48758783821671,6.59413245076532,6.69917767867827,6.81244210168984),
 .UNSPECIFIED.);
#2382=B_SPLINE_CURVE_WITH_KNOTS('',3,(#40914,#40915,#40916,#40917,#40918,
#40919,#40920,#40921,#40922,#40923,#40924,#40925,#40926,#40927,#40928,#40929,
#40930,#40931,#40932,#40933,#40934,#40935,#40936,#40937,#40938,#40939,#40940,
#40941,#40942,#40943,#40944,#40945,#40946,#40947,#40948,#40949,#40950,#40951,
#40952,#40953,#40954,#40955,#40956,#40957,#40958,#40959,#40960,#40961,#40962,
#40963,#40964,#40965,#40966,#40967,#40968,#40969,#40970,#40971,#40972,#40973,
#40974,#40975,#40976,#40977,#40978,#40979,#40980,#40981,#40982,#40983,#40984,
#40985,#40986,#40987,#40988,#40989,#40990,#40991,#40992,#40993,#40994,#40995,
#40996,#40997,#40998,#40999,#41000,#41001,#41002,#41003,#41004,#41005,#41006,
#41007,#41008,#41009,#41010,#41011,#41012,#41013,#41014,#41015,#41016,#41017,
#41018,#41019,#41020,#41021,#41022,#41023),.UNSPECIFIED.,.F.,.F.,(4,2,2,
2,2,2,2,2,2,2,2,2,2,2,2,2,2,2,2,2,2,2,2,2,2,2,2,2,2,2,2,2,2,2,2,2,2,2,2,
2,2,2,2,2,2,2,2,2,2,2,2,2,2,2,4),(-6.81071791048935,-6.69748642459302,-6.59246866459779,
-6.48595191203587,-6.38279446767657,-6.25885338583429,-6.1159547110793,
-5.96462704393112,-5.84064490893926,-5.73213421546912,-5.6220672998129,
-5.51548783412999,-5.38750799195991,-5.24003556739288,-5.08379343005054,
-4.95587212998563,-4.84389697405391,-4.73035120088386,-4.62038369588879,
-4.48840638789589,-4.33641984614675,-4.17530713008141,-4.04349505314758,
-3.92809108478184,-3.81110989139477,-3.69779242286604,-3.5618751351377,
-3.40545367974512,-3.24903222435254,-3.1131149366242,-2.99979746809548,
-2.8828162747084,-2.76741230634266,-2.63560022940884,-2.47448751334349,
-2.32250097159435,-2.19052366360146,-2.08055615860636,-1.96701038543629,
-1.85503522950457,-1.72711392943967,-1.5708717920973,-1.42339936753026,
-1.29541952536018,-1.18884005967721,-1.07877314402097,-0.970262450550858,
-0.846280315558988,-0.694952648410747,-0.552053973655728,-0.428112891813464,
-0.324955447454145,-0.218438694892192,-0.113420934896934,-0.000186114852025488),
 .UNSPECIFIED.);
#2383=B_SPLINE_CURVE_WITH_KNOTS('',3,(#41166,#41167,#41168,#41169,#41170,
#41171,#41172,#41173,#41174,#41175,#41176,#41177,#41178,#41179,#41180,#41181,
#41182,#41183,#41184,#41185,#41186,#41187,#41188,#41189,#41190,#41191,#41192,
#41193,#41194,#41195,#41196,#41197,#41198,#41199,#41200,#41201,#41202,#41203,
#41204,#41205,#41206,#41207,#41208,#41209,#41210,#41211,#41212,#41213,#41214,
#41215,#41216,#41217,#41218,#41219,#41220,#41221,#41222,#41223,#41224,#41225,
#41226,#41227,#41228,#41229,#41230,#41231,#41232,#41233,#41234,#41235,#41236,
#41237,#41238,#41239,#41240,#41241,#41242,#41243,#41244,#41245,#41246,#41247,
#41248,#41249,#41250,#41251,#41252,#41253,#41254,#41255,#41256,#41257,#41258,
#41259,#41260,#41261,#41262,#41263,#41264,#41265,#41266,#41267,#41268,#41269,
#41270,#41271,#41272,#41273,#41274,#41275,#41276,#41277,#41278,#41279,#41280,
#41281,#41282,#41283,#41284,#41285,#41286,#41287,#41288,#41289,#41290,#41291,
#41292,#41293,#41294,#41295,#41296,#41297,#41298,#41299,#41300,#41301,#41302,
#41303,#41304,#41305,#41306,#41307,#41308,#41309,#41310,#41311,#41312,#41313,
#41314,#41315,#41316,#41317,#41318,#41319,#41320,#41321,#41322,#41323,#41324,
#41325,#41326,#41327,#41328,#41329,#41330,#41331,#41332,#41333,#41334,#41335,
#41336,#41337,#41338,#41339,#41340,#41341,#41342,#41343,#41344,#41345),
 .UNSPECIFIED.,.F.,.F.,(4,2,2,2,2,2,2,2,2,2,2,2,2,2,2,2,2,2,2,2,2,2,2,2,
2,2,2,2,2,2,2,2,2,2,2,2,2,2,2,2,2,2,2,2,2,2,2,2,2,2,2,2,2,2,2,2,2,2,2,2,
2,2,2,2,2,2,2,2,2,2,2,2,2,2,2,2,2,2,2,2,2,2,2,2,2,2,2,2,2,4),(-5.86988290593197,
-5.83799332401546,-5.79410197724347,-5.73947964729276,-5.62977741049655,
-5.57972122260326,-5.51896918907118,-5.47512868052878,-5.35958775805997,
-5.30757022918753,-5.24754404245887,-5.20428195828346,-5.07801471872521,
-5.02875474902955,-4.97324450334103,-4.93014937845045,-4.80416147096541,
-4.7550384082473,-4.6997479903665,-4.65670129543007,-4.53092765933326,-4.48187016125483,
-4.42666019747262,-4.38368480638791,-4.25812788045421,-4.20914763124866,
-4.15399926806423,-4.11109081074757,-3.98580328536774,-3.93688802667624,
-3.88176062631921,-3.83890805816712,-3.71404101847719,-3.66515154462887,
-3.60985929431661,-3.56702816116338,-3.44313083149954,-3.39412861872233,
-3.33802934768471,-3.29508939030358,-3.17422274637664,-3.12456077020254,
-3.06526182537254,-3.02164022195564,-2.91325098632136,-2.85041530839486,
-2.80367996750775,-2.77122802009947,-2.72111557671893,-2.65878038666057,
-2.57421680926107,-2.52981130868839,-2.46204933981601,-2.4091686270665,
-2.30227765142875,-2.25801195797186,-2.19063687866087,-2.1378305403487,
-2.03047221215058,-1.98620174494898,-1.91885234144652,-1.86602471087127,
-1.75851326634842,-1.71421318079729,-1.64682064027922,-1.5939543206139,
-1.48634182173124,-1.4420067412229,-1.37457067592944,-1.32166044695823,
-1.21396913119586,-1.16959665799744,-1.10210581435966,-1.04916806628168,
-0.941379231431628,-0.896990858089643,-0.829343262584152,-0.776309816913608,
-0.668367641255489,-0.623859599579781,-0.556774519076718,-0.503805192902935,
-0.396308068918789,-0.351980356323967,-0.288013742466906,-0.237877191458961,
-0.129159111742741,-0.075595333196945,-0.031302567710868,-0.000193940477510359),
 .UNSPECIFIED.);
#2384=B_SPLINE_CURVE_WITH_KNOTS('',3,(#41487,#41488,#41489,#41490,#41491,
#41492,#41493,#41494,#41495,#41496,#41497,#41498,#41499,#41500,#41501,#41502,
#41503,#41504,#41505,#41506,#41507,#41508,#41509,#41510,#41511,#41512,#41513,
#41514,#41515,#41516,#41517,#41518,#41519,#41520,#41521,#41522,#41523,#41524,
#41525,#41526,#41527,#41528,#41529,#41530,#41531,#41532,#41533,#41534,#41535,
#41536,#41537,#41538,#41539,#41540,#41541,#41542,#41543,#41544,#41545,#41546,
#41547,#41548,#41549,#41550,#41551,#41552,#41553,#41554,#41555,#41556,#41557,
#41558,#41559,#41560,#41561,#41562,#41563,#41564,#41565,#41566,#41567,#41568,
#41569,#41570,#41571,#41572,#41573,#41574,#41575,#41576,#41577,#41578,#41579,
#41580,#41581,#41582,#41583,#41584,#41585,#41586,#41587,#41588,#41589,#41590,
#41591,#41592,#41593,#41594,#41595,#41596),.UNSPECIFIED.,.F.,.F.,(4,2,2,
2,2,2,2,2,2,2,2,2,2,2,2,2,2,2,2,2,2,2,2,2,2,2,2,2,2,2,2,2,2,2,2,2,2,2,2,
2,2,2,2,2,2,2,2,2,2,2,2,2,2,2,4),(-2.49584851444866,-2.42086616323668,-2.38614802829034,
-2.32969252891064,-2.28689945253446,-2.25395120746466,-2.19725039548955,
-2.14933335428152,-2.11468560901464,-2.06295576638154,-2.01712270260594,
-1.9832659184357,-1.92918001564781,-1.87970035978081,-1.84448761932614,
-1.7909980855805,-1.7462609286404,-1.71281222802058,-1.65811618243505,-1.60936580617528,
-1.5744861659387,-1.52084660708105,-1.47650724803446,-1.44321711480835,
-1.38159961844885,-1.33711580712783,-1.3035798530162,-1.2440853340121,-1.19077695863606,
-1.15694577714375,-1.11233093085342,-1.05023681326708,-1.01665656842421,
-0.970997769558366,-0.919431423775674,-0.883873349329957,-0.834016049267621,
-0.780973472692911,-0.747397098791494,-0.702008621311116,-0.649456920662372,
-0.613558084171164,-0.562951419053681,-0.510583395420632,-0.476597773425144,
-0.430104647279553,-0.379361620258774,-0.344100444554333,-0.295183740065816,
-0.240012225361866,-0.207030628428394,-0.163797587969506,-0.107959271216929,
-0.0724909230265645,-0.000105906793946138),.UNSPECIFIED.);
#2385=B_SPLINE_CURVE_WITH_KNOTS('',3,(#41739,#41740,#41741,#41742,#41743,
#41744,#41745,#41746,#41747,#41748,#41749,#41750,#41751,#41752,#41753,#41754,
#41755,#41756,#41757,#41758,#41759,#41760,#41761,#41762,#41763,#41764,#41765,
#41766,#41767,#41768,#41769,#41770,#41771,#41772,#41773,#41774,#41775,#41776,
#41777,#41778,#41779,#41780,#41781,#41782,#41783,#41784,#41785,#41786,#41787,
#41788,#41789,#41790,#41791,#41792,#41793,#41794,#41795,#41796,#41797,#41798,
#41799,#41800,#41801,#41802,#41803,#41804,#41805,#41806,#41807,#41808,#41809,
#41810,#41811,#41812,#41813,#41814,#41815,#41816,#41817,#41818,#41819,#41820,
#41821,#41822,#41823,#41824,#41825,#41826,#41827,#41828,#41829,#41830,#41831,
#41832,#41833,#41834,#41835,#41836,#41837,#41838,#41839,#41840,#41841,#41842,
#41843,#41844,#41845,#41846,#41847,#41848,#41849,#41850,#41851,#41852,#41853,
#41854,#41855,#41856,#41857,#41858,#41859,#41860,#41861,#41862,#41863,#41864,
#41865,#41866,#41867,#41868,#41869,#41870,#41871,#41872,#41873,#41874,#41875,
#41876,#41877,#41878,#41879,#41880,#41881,#41882,#41883,#41884,#41885,#41886,
#41887,#41888,#41889,#41890,#41891,#41892,#41893,#41894,#41895,#41896,#41897,
#41898,#41899,#41900,#41901,#41902,#41903,#41904,#41905,#41906,#41907,#41908,
#41909,#41910,#41911,#41912,#41913,#41914,#41915,#41916),.UNSPECIFIED.,
 .F.,.F.,(4,2,2,2,2,2,2,2,2,2,2,2,2,2,2,2,2,2,2,2,2,2,2,2,2,2,2,2,2,2,2,
2,2,2,2,2,2,2,2,2,2,2,2,2,2,2,2,2,2,2,2,2,2,2,2,2,2,2,2,2,2,2,2,2,2,2,2,
2,2,2,2,2,2,2,2,2,2,2,2,2,2,2,2,2,2,2,2,2,4),(-5.81343192393955,-5.78194346696491,
-5.73860415445271,-5.68466898290961,-5.57634666406845,-5.52692010070965,
-5.46693218365186,-5.4236431138491,-5.30955586922977,-5.25819254093151,
-5.19892102074225,-5.15620304728678,-5.03152512823552,-4.98288452023335,
-4.92807128029553,-4.88551799894344,-4.761118517748,-4.71261244572808,-4.65801319340276,
-4.61550715243308,-4.49132836731065,-4.44288477248686,-4.38835425229245,
-4.34591659340536,-4.22198359917362,-4.17360838650696,-4.11910134060711,
-4.07672268689262,-3.95316704188153,-3.90482827128912,-3.85021123988982,
-3.80786268380277,-3.68511673907705,-3.63670402666718,-3.58146188061304,
-3.53904198777237,-3.41871675745947,-3.36980866685654,-3.31206741735705,
-3.26914721180126,-3.15695262661369,-3.10594423568562,-3.0396793434762,
-2.99407929884949,-2.91424701825505,-2.82416604159401,-2.78115665183707,
-2.71647252526577,-2.66484413909547,-2.55173705551146,-2.51017912487732,
-2.45062249495088,-2.40013388510142,-2.28229703494248,-2.2409509298103,
-2.18252957317486,-2.13221307248469,-2.01310169337678,-1.97173795571909,
-1.91349444879949,-1.86313974466627,-1.74354587650129,-1.70211444989438,
-1.64382017524692,-1.59337849490485,-1.47348244784259,-1.43197037520573,
-1.3735829242948,-1.32304103988193,-1.20289737935556,-1.16130054378407,
-1.10279889411852,-1.05216928238786,-0.931771617962573,-0.890109738866415,
-0.8313818925562,-0.780597212044168,-0.659883751882108,-0.618052880715235,
-0.559845381164947,-0.509078297483705,-0.388637749176731,-0.346952093505117,
-0.286460606447632,-0.235650373603816,-0.127852847589458,-0.0744147835208843,
-0.0312981374707393,-0.000207727027547122),.UNSPECIFIED.);
#2386=B_SPLINE_CURVE_WITH_KNOTS('',3,(#41918,#41919,#41920,#41921,#41922,
#41923,#41924,#41925,#41926,#41927,#41928,#41929,#41930,#41931,#41932,#41933,
#41934,#41935,#41936,#41937,#41938,#41939,#41940,#41941,#41942,#41943,#41944,
#41945,#41946,#41947,#41948,#41949,#41950,#41951,#41952,#41953,#41954,#41955,
#41956,#41957,#41958,#41959,#41960,#41961,#41962,#41963,#41964,#41965,#41966,
#41967,#41968,#41969,#41970,#41971,#41972,#41973,#41974,#41975,#41976,#41977,
#41978,#41979,#41980,#41981,#41982,#41983,#41984,#41985,#41986,#41987,#41988,
#41989,#41990,#41991,#41992,#41993,#41994,#41995,#41996,#41997,#41998,#41999,
#42000,#42001,#42002,#42003,#42004,#42005,#42006,#42007,#42008,#42009,#42010,
#42011,#42012,#42013,#42014,#42015,#42016,#42017,#42018,#42019,#42020,#42021,
#42022,#42023,#42024,#42025,#42026,#42027),.UNSPECIFIED.,.F.,.F.,(4,2,2,
2,2,2,2,2,2,2,2,2,2,2,2,2,2,2,2,2,2,2,2,2,2,2,2,2,2,2,2,2,2,2,2,2,2,2,2,
2,2,2,2,2,2,2,2,2,2,2,2,2,2,2,4),(-2.49855388017476,-2.42342814551093,-2.3886436215689,
-2.33208016642435,-2.28920525988184,-2.25619401022828,-2.19938477359639,
-2.1513761038903,-2.11666210416291,-2.06483328147968,-2.01891261002298,
-1.98499109214821,-1.9308014529537,-1.88122737363105,-1.84594735686781,
-1.79236561780895,-1.74753713913737,-1.71402314799028,-1.65928344444008,
-1.61040262535647,-1.57544496390384,-1.5201610388553,-1.47660780572407,
-1.44344956811401,-1.38267536477288,-1.33782063810444,-1.30413387384197,
-1.24902398769069,-1.18682567208135,-1.1497092469778,-1.09474953306849,
-1.04753155189499,-1.01198397316158,-0.958727816046237,-0.917591786477728,
-0.880296196817386,-0.824910897146943,-0.780056305587087,-0.74596103696419,
-0.698528616918437,-0.649434328880524,-0.613516472675831,-0.562850084374765,
-0.51057844847517,-0.476590111852955,-0.430086093677056,-0.379361558957249,
-0.34410033730707,-0.295183489536067,-0.240012217833707,-0.207030618161296,
-0.163797566109981,-0.107959290444451,-0.0724909555157676,-0.000105906793936821),
 .UNSPECIFIED.);
#2387=B_SPLINE_CURVE_WITH_KNOTS('',3,(#42030,#42031,#42032,#42033,#42034,
#42035,#42036,#42037,#42038,#42039,#42040,#42041,#42042,#42043,#42044,#42045,
#42046,#42047,#42048,#42049,#42050,#42051,#42052,#42053,#42054,#42055,#42056,
#42057,#42058,#42059,#42060,#42061,#42062,#42063,#42064,#42065,#42066,#42067,
#42068,#42069,#42070,#42071,#42072,#42073,#42074,#42075,#42076,#42077,#42078,
#42079,#42080,#42081,#42082,#42083,#42084,#42085,#42086,#42087,#42088,#42089,
#42090,#42091,#42092,#42093,#42094,#42095,#42096,#42097,#42098,#42099,#42100,
#42101,#42102,#42103,#42104,#42105,#42106,#42107,#42108,#42109,#42110,#42111,
#42112,#42113,#42114,#42115,#42116,#42117,#42118,#42119,#42120,#42121,#42122,
#42123,#42124,#42125,#42126,#42127,#42128,#42129,#42130,#42131,#42132,#42133,
#42134,#42135,#42136,#42137,#42138,#42139),.UNSPECIFIED.,.F.,.F.,(4,2,2,
2,2,2,2,2,2,2,2,2,2,2,2,2,2,2,2,2,2,2,2,2,2,2,2,2,2,2,2,2,2,2,2,2,2,2,2,
2,2,2,2,2,2,2,2,2,2,2,2,2,2,2,4),(0.000186114852028536,0.113420934897052,
0.218438694892283,0.32495544745418,0.428112891813475,0.552053973655751,
0.694952648410875,0.846280315559075,0.970262450550931,1.07877314402106,
1.18884005967728,1.29541952536018,1.42339936753021,1.57087179209733,1.72711392943967,
1.85503522950455,1.96701038543624,2.08055615860629,2.19052366360141,2.32250097159434,
2.47448751334346,2.63560022940877,2.76741230634255,2.88281627470825,2.99979746809535,
3.11311493662413,3.2490322243525,3.40545367974495,3.56187513513741,3.69779242286587,
3.81110989139468,3.92809108478164,4.04349505314729,4.17530713008115,4.33641984614643,
4.48840638789552,4.62038369588843,4.73035120088352,4.84389697405351,4.9558721299852,
5.08379343005007,5.24003556739236,5.38750799195943,5.51548783412943,5.6220672998123,
5.7321342154685,5.84064490893866,5.96462704393049,6.11595471107872,6.25885338583376,
6.382794467676,6.48595191203529,6.59246866459722,6.69748642459247,6.81072123047711),
 .UNSPECIFIED.);
#2388=B_SPLINE_CURVE_WITH_KNOTS('',3,(#42281,#42282,#42283,#42284,#42285,
#42286,#42287,#42288,#42289,#42290,#42291,#42292,#42293,#42294,#42295,#42296,
#42297,#42298,#42299,#42300,#42301,#42302,#42303,#42304,#42305,#42306,#42307,
#42308,#42309,#42310,#42311,#42312,#42313,#42314,#42315,#42316,#42317,#42318,
#42319,#42320,#42321,#42322,#42323,#42324,#42325,#42326,#42327,#42328,#42329,
#42330,#42331,#42332,#42333,#42334,#42335,#42336,#42337,#42338,#42339,#42340,
#42341,#42342,#42343,#42344,#42345,#42346,#42347,#42348,#42349,#42350,#42351,
#42352,#42353,#42354,#42355,#42356,#42357,#42358,#42359,#42360,#42361,#42362,
#42363,#42364,#42365,#42366,#42367,#42368,#42369,#42370,#42371,#42372,#42373,
#42374,#42375,#42376,#42377,#42378,#42379,#42380,#42381,#42382,#42383,#42384,
#42385,#42386,#42387,#42388,#42389,#42390),.UNSPECIFIED.,.F.,.F.,(4,2,2,
2,2,2,2,2,2,2,2,2,2,2,2,2,2,2,2,2,2,2,2,2,2,2,2,2,2,2,2,2,2,2,2,2,2,2,2,
2,2,2,2,2,2,2,2,2,2,2,2,2,2,2,4),(-6.81072123047651,-6.69748642459177,-6.59246866459655,
-6.48595191203466,-6.38279446767538,-6.25885338583311,-6.115954711078,-5.96462704392981,
-5.84064490893797,-5.73213421546785,-5.62206729981164,-5.51548783412876,
-5.38750799195874,-5.24003556739163,-5.08379343004931,-4.95587212998444,
-4.84389697405276,-4.73035120088272,-4.6203836958876,-4.4884063878947,-4.33641984614558,
-4.17530713008029,-4.04349505314652,-3.92809108478083,-3.81110989139374,
-3.69779242286497,-3.56187513513662,-3.40545367974418,-3.24903222435173,
-3.11311493662328,-2.99979746809448,-2.88281627470753,-2.76741230634189,
-2.63560022940804,-2.47448751334277,-2.3225009715937,-2.1905236636008,-2.08055615860572,
-1.96701038543575,-1.85503522950406,-1.7271139294392,-1.57087179209693,
-1.42339936752987,-1.29541952535988,-1.18884005967702,-1.07877314402082,
-0.970262450550672,-0.84628031555885,-0.694952648410639,-0.552053973655609,
-0.428112891813383,-0.324955447454098,-0.218438694892172,-0.113420934896926,
-0.000186114852029566),.UNSPECIFIED.);
#2389=B_SPLINE_CURVE_WITH_KNOTS('',3,(#42533,#42534,#42535,#42536,#42537,
#42538,#42539,#42540,#42541,#42542,#42543,#42544,#42545,#42546,#42547,#42548,
#42549,#42550,#42551,#42552,#42553,#42554,#42555,#42556,#42557,#42558,#42559,
#42560,#42561,#42562,#42563,#42564,#42565,#42566,#42567,#42568,#42569,#42570,
#42571,#42572,#42573,#42574,#42575,#42576,#42577,#42578,#42579,#42580,#42581,
#42582,#42583,#42584,#42585,#42586,#42587,#42588,#42589,#42590,#42591,#42592,
#42593,#42594,#42595,#42596,#42597,#42598,#42599,#42600,#42601,#42602,#42603,
#42604,#42605,#42606,#42607,#42608,#42609,#42610,#42611,#42612,#42613,#42614,
#42615,#42616,#42617,#42618,#42619,#42620,#42621,#42622,#42623,#42624,#42625,
#42626,#42627,#42628,#42629,#42630,#42631,#42632,#42633,#42634,#42635,#42636,
#42637,#42638,#42639,#42640,#42641,#42642),.UNSPECIFIED.,.F.,.F.,(4,2,2,
2,2,2,2,2,2,2,2,2,2,2,2,2,2,2,2,2,2,2,2,2,2,2,2,2,2,2,2,2,2,2,2,2,2,2,2,
2,2,2,2,2,2,2,2,2,2,2,2,2,2,2,4),(-6.81072186467709,-6.69748703256578,-6.59246924824708,
-6.48595247101454,-6.38279500276269,-6.25885389221412,-6.11595518436193,
-5.9646274821643,-5.84064531845661,-5.73213459985401,-5.62206765870493,
-5.51548816833691,-5.38750829652513,-5.24003583780158,-5.0837936642716,
-4.95587233457851,-4.84389715271197,-4.73035135324333,-4.62038382277836,
-4.48840648421781,-4.33641990726669,-4.17530715388565,-4.04349504642242,
-3.9280910513277,-3.81110983084635,-3.69779233607186,-3.56187501686334,
-3.40545352524158,-3.24903203361983,-3.11311471441129,-2.99979721963673,
-2.88281599915529,-2.76741200406055,-2.63559989659742,-2.47448714321635,
-2.32250056626518,-2.19052322770464,-2.08055569723965,-1.96700989777096,
-1.85503471590438,-1.72711338621126,-1.57087121268124,-1.42339875395765,
-1.29541888214586,-1.18883939177779,-1.07877245062866,-0.970261732026059,
-0.84627956831836,-0.694951866120717,-0.552053158268449,-0.428112047719832,
-0.324954579467925,-0.218437802235375,-0.113420017916685,-0.000184814530532018),
 .UNSPECIFIED.);
#2390=B_SPLINE_CURVE_WITH_KNOTS('',3,(#42643,#42644,#42645,#42646,#42647,
#42648),.UNSPECIFIED.,.F.,.F.,(4,2,4),(-0.0463376484595311,-0.0232792425040161,
-2.35223677633965E-5),.UNSPECIFIED.);
#2391=B_SPLINE_CURVE_WITH_KNOTS('',3,(#42649,#42650,#42651,#42652,#42653,
#42654,#42655,#42656,#42657,#42658,#42659,#42660,#42661,#42662,#42663,#42664,
#42665,#42666,#42667,#42668,#42669,#42670,#42671,#42672,#42673,#42674,#42675,
#42676,#42677,#42678,#42679,#42680,#42681,#42682,#42683,#42684,#42685,#42686,
#42687,#42688,#42689,#42690,#42691,#42692,#42693,#42694,#42695,#42696,#42697,
#42698,#42699,#42700,#42701,#42702,#42703,#42704,#42705,#42706,#42707,#42708,
#42709,#42710,#42711,#42712,#42713,#42714,#42715,#42716,#42717,#42718,#42719,
#42720,#42721,#42722,#42723,#42724,#42725,#42726,#42727,#42728,#42729,#42730,
#42731,#42732,#42733,#42734,#42735,#42736,#42737,#42738,#42739,#42740,#42741,
#42742,#42743,#42744,#42745,#42746,#42747,#42748,#42749,#42750,#42751,#42752,
#42753,#42754,#42755,#42756,#42757,#42758,#42759,#42760,#42761,#42762,#42763,
#42764,#42765,#42766,#42767,#42768,#42769,#42770,#42771,#42772,#42773,#42774,
#42775,#42776,#42777,#42778,#42779,#42780,#42781,#42782,#42783,#42784,#42785,
#42786,#42787,#42788,#42789,#42790,#42791,#42792,#42793,#42794,#42795,#42796,
#42797,#42798,#42799,#42800,#42801,#42802,#42803,#42804,#42805,#42806,#42807,
#42808,#42809,#42810,#42811,#42812,#42813,#42814,#42815,#42816,#42817,#42818,
#42819,#42820,#42821,#42822,#42823,#42824,#42825,#42826),.UNSPECIFIED.,
 .F.,.F.,(4,2,2,2,2,2,2,2,2,2,2,2,2,2,2,2,2,2,2,2,2,2,2,2,2,2,2,2,2,2,2,
2,2,2,2,2,2,2,2,2,2,2,2,2,2,2,2,2,2,2,2,2,2,2,2,2,2,2,2,2,2,2,2,2,2,2,2,
2,2,2,2,2,2,2,2,2,2,2,2,2,2,2,2,2,2,2,2,2,4),(-5.81158509839654,-5.78007408364135,
-5.73690027962185,-5.68285782741762,-5.57464154317438,-5.5252442398387,
-5.46529189609478,-5.42202845680168,-5.30800824915912,-5.25667545783596,
-5.19743952887423,-5.15474692022444,-5.03014130861183,-4.98152983756949,
-4.92675073446084,-4.88422295126807,-4.75989199425356,-4.7114158759881,
-4.65685488190427,-4.61437511286984,-4.49025212361444,-4.44184157097751,
-4.38736406263288,-4.3449554315813,-4.22103416306194,-4.17270285247783,
-4.11830038804471,-4.07596050565412,-3.95226274312296,-3.90400608326453,
-3.84967403192356,-3.80739874540725,-3.68396757439753,-3.6357733449824,
-3.58145273720433,-3.53923214088518,-3.41623040582683,-3.36805825972575,
-3.31355917139572,-3.27135621400733,-3.14936222041352,-3.10106551523939,
-3.03930670133814,-2.9934508296899,-2.91534231128656,-2.8237282641102,-2.78088320114212,
-2.71668216090014,-2.66517461717443,-2.55168867130034,-2.51014507494687,
-2.45064697615994,-2.40017133277286,-2.28228599391634,-2.2409429664815,
-2.1825352375726,-2.13222166770922,-2.0130990851343,-1.97173606397672,-1.91349579123466,
-1.8631417778932,-1.74354525541854,-1.70211399882852,-1.64382049510977,
-1.59337897915575,-1.47348229965046,-1.43197026753863,-1.37358300059391,
-1.32304115540395,-1.20289734397171,-1.1613005180707,-1.10279891231429,
-1.052169309939,-0.931771609500933,-0.890109732715275,-0.831381896884102,
-0.78059721860677,-0.659883749855692,-0.618052879239476,-0.559845382197793,
-0.50907829905577,-0.388637748692026,-0.346952093154151,-0.286460606693424,
-0.235650373973567,-0.127852847812578,-0.074414783243345,-0.031298137464462,
-0.000207727027570367),.UNSPECIFIED.);
#2392=B_SPLINE_CURVE_WITH_KNOTS('',3,(#42968,#42969,#42970,#42971,#42972,
#42973),.UNSPECIFIED.,.F.,.F.,(4,2,4),(-0.0464673921126319,-0.0232138500385779,
-5.92302360825546E-5),.UNSPECIFIED.);
#2393=B_SPLINE_CURVE_WITH_KNOTS('',3,(#42974,#42975,#42976,#42977,#42978,
#42979,#42980,#42981,#42982,#42983,#42984,#42985,#42986,#42987,#42988,#42989,
#42990,#42991,#42992,#42993,#42994,#42995,#42996,#42997,#42998,#42999,#43000,
#43001,#43002,#43003,#43004,#43005,#43006,#43007,#43008,#43009,#43010,#43011,
#43012,#43013,#43014,#43015,#43016,#43017,#43018,#43019,#43020,#43021,#43022,
#43023,#43024,#43025,#43026,#43027,#43028,#43029,#43030,#43031,#43032,#43033,
#43034,#43035,#43036,#43037,#43038,#43039,#43040,#43041,#43042,#43043,#43044,
#43045,#43046,#43047,#43048,#43049,#43050,#43051,#43052,#43053,#43054,#43055,
#43056,#43057,#43058,#43059,#43060,#43061,#43062,#43063,#43064,#43065,#43066,
#43067,#43068,#43069,#43070,#43071,#43072,#43073,#43074,#43075,#43076,#43077,
#43078,#43079,#43080,#43081,#43082,#43083),.UNSPECIFIED.,.F.,.F.,(4,2,2,
2,2,2,2,2,2,2,2,2,2,2,2,2,2,2,2,2,2,2,2,2,2,2,2,2,2,2,2,2,2,2,2,2,2,2,2,
2,2,2,2,2,2,2,2,2,2,2,2,2,2,2,4),(0.000186114852028654,0.113420934896994,
0.218438694892263,0.324955447454189,0.428112891813479,0.552053973655729,
0.69495264841079,0.846280315559027,0.970262450550892,1.07877314402105,1.18884005967725,
1.29541952536013,1.42339936753017,1.57087179209725,1.72711392943958,1.85503522950449,
1.96701038543619,2.08055615860619,2.1905236636013,2.32250097159425,2.47448751334338,
2.63560022940869,2.76741230634258,2.8828162747083,2.99979746809533,3.11311493662407,
3.24903222435243,3.40545367974502,3.56187513513759,3.69779242286599,3.81110989139479,
3.92809108478191,4.04349505314765,4.17530713008144,4.33641984614678,4.48840638789596,
4.6203836958889,4.73035120088403,4.84389697405409,4.95587212998582,5.08379343005076,
5.24003556739313,5.38750799196026,5.51548783413032,5.62206729981324,5.73213421546949,
5.84064490893965,5.96462704393152,6.11595471107978,6.25885338583492,6.38279446767723,
6.48595191203657,6.59246866459851,6.69748642459376,6.81072158854588),
 .UNSPECIFIED.);
#2394=B_SPLINE_CURVE_WITH_KNOTS('',3,(#43225,#43226,#43227,#43228,#43229,
#43230),.UNSPECIFIED.,.F.,.F.,(4,2,4),(-0.0289951303379412,-0.014591319104119,
-0.000183151741413589),.UNSPECIFIED.);
#2395=B_SPLINE_CURVE_WITH_KNOTS('',3,(#43381,#43382,#43383,#43384,#43385,
#43386,#43387,#43388,#43389,#43390,#43391,#43392,#43393,#43394,#43395,#43396,
#43397,#43398,#43399,#43400,#43401,#43402,#43403),.UNSPECIFIED.,.F.,.F.,
(4,2,2,2,2,3,2,2,2,2,4),(-0.599381390807594,-0.519369386765995,-0.439357382724396,
-0.329518037043297,-0.219678691362198,0.,0.219678691362198,0.329518037043297,
0.439357382724396,0.519369386765995,0.599381390807594),.UNSPECIFIED.);
#2396=B_SPLINE_CURVE_WITH_KNOTS('',3,(#43404,#43405,#43406,#43407,#43408,
#43409,#43410,#43411,#43412,#43413,#43414,#43415,#43416,#43417,#43418,#43419,
#43420,#43421,#43422,#43423,#43424,#43425),.UNSPECIFIED.,.F.,.F.,(4,2,2,
2,2,2,2,2,2,2,4),(0.599381390807594,0.679393394849193,0.759405398890792,
0.869244744571891,0.97908409025299,1.19876278161519,1.41844147297739,1.52828081865849,
1.63812016433958,1.71813216838118,1.79814417242278),.UNSPECIFIED.);
#2397=B_SPLINE_CURVE_WITH_KNOTS('',3,(#43436,#43437,#43438,#43439,#43440,
#43441,#43442,#43443,#43444,#43445,#43446,#43447,#43448,#43449,#43450,#43451,
#43452,#43453,#43454,#43455,#43456,#43457,#43458,#43459,#43460,#43461,#43462,
#43463,#43464,#43465,#43466,#43467,#43468,#43469,#43470,#43471,#43472,#43473,
#43474,#43475,#43476,#43477,#43478,#43479,#43480,#43481,#43482,#43483,#43484,
#43485,#43486,#43487,#43488,#43489,#43490,#43491,#43492,#43493,#43494,#43495,
#43496,#43497,#43498,#43499,#43500,#43501,#43502,#43503,#43504,#43505,#43506,
#43507,#43508,#43509,#43510,#43511,#43512,#43513,#43514,#43515,#43516,#43517,
#43518,#43519,#43520,#43521,#43522,#43523,#43524,#43525,#43526,#43527,#43528,
#43529,#43530,#43531,#43532,#43533,#43534,#43535,#43536,#43537,#43538,#43539,
#43540,#43541,#43542,#43543,#43544,#43545,#43546,#43547,#43548,#43549,#43550,
#43551,#43552,#43553,#43554,#43555,#43556,#43557,#43558,#43559,#43560,#43561,
#43562,#43563,#43564,#43565,#43566,#43567,#43568,#43569,#43570,#43571,#43572,
#43573,#43574,#43575,#43576,#43577,#43578,#43579,#43580,#43581,#43582,#43583,
#43584,#43585,#43586,#43587,#43588,#43589,#43590,#43591,#43592,#43593,#43594,
#43595,#43596,#43597,#43598),.UNSPECIFIED.,.F.,.F.,(4,3,3,3,3,3,3,3,3,3,
3,3,3,3,3,3,3,3,3,3,3,3,3,3,3,3,3,3,3,3,3,3,3,3,3,3,3,3,3,3,3,3,3,3,3,3,
3,3,3,3,3,3,3,3,4),(0.,0.0271485983010553,0.05263157894737,0.0811718380673146,
0.1052631578947,0.135206120413793,0.1578947368421,0.189291818846306,0.2105263157895,
0.243358105064165,0.2631578947368,0.294194908421614,0.297337794500015,0.3157894736842,
0.340129611785252,0.3513224823538,0.3684210526316,0.389398663890277,0.405409303715733,
0.4210526315789,0.443739980215653,0.459561087966757,0.4736842105263,0.493656585303444,
0.512541581707809,0.513628960080588,0.5263157894737,0.55624241470489,0.567623145833444,
0.5789473684211,0.606798151158574,0.621680971678114,0.6315789473684,0.661305928252685,
0.675748561652349,0.6842105263158,0.720695129581258,0.72974635703808,0.7368421052632,
0.765451968761437,0.783751433607901,0.7894736842105,0.813669118094079,0.837825750838692,
0.8421052631579,0.867000882414173,0.891896501670446,0.8947368421053,0.916009887512648,
0.936015949101071,0.945950981672964,0.9473684210526,0.9668595667857,0.985375475970587,
0.999999996167332),.UNSPECIFIED.);
#2398=B_SPLINE_CURVE_WITH_KNOTS('',3,(#43602,#43603,#43604,#43605,#43606,
#43607,#43608,#43609,#43610,#43611),.UNSPECIFIED.,.F.,.F.,(4,3,3,4),(0.,
0.3333333333333,0.6666666666667,1.),.UNSPECIFIED.);
#2399=B_SPLINE_CURVE_WITH_KNOTS('',3,(#43613,#43614,#43615,#43616,#43617,
#43618,#43619,#43620,#43621),.UNSPECIFIED.,.F.,.F.,(4,1,1,1,1,1,4),(2.5958560708529E-7,
0.1666666666667,0.3333333333333,0.5,0.6666666666667,0.8333333333333,0.999999934146645),
 .UNSPECIFIED.);
#2400=B_SPLINE_CURVE_WITH_KNOTS('',3,(#43623,#43624,#43625,#43626,#43627,
#43628,#43629,#43630),.UNSPECIFIED.,.F.,.F.,(4,1,1,1,1,4),(5.10274934168318E-8,
0.2,0.4,0.6,0.8,1.),.UNSPECIFIED.);
#2401=B_SPLINE_CURVE_WITH_KNOTS('',3,(#43670,#43671,#43672,#43673,#43674,
#43675,#43676,#43677,#43678,#43679,#43680,#43681,#43682,#43683,#43684,#43685,
#43686,#43687,#43688,#43689,#43690,#43691,#43692,#43693,#43694,#43695,#43696,
#43697,#43698,#43699,#43700,#43701,#43702,#43703,#43704,#43705,#43706,#43707,
#43708,#43709,#43710,#43711,#43712,#43713,#43714,#43715,#43716,#43717,#43718,
#43719,#43720,#43721,#43722,#43723,#43724,#43725,#43726,#43727,#43728,#43729,
#43730,#43731,#43732,#43733,#43734,#43735,#43736,#43737,#43738,#43739,#43740,
#43741,#43742,#43743,#43744,#43745,#43746,#43747,#43748,#43749,#43750,#43751,
#43752,#43753,#43754,#43755,#43756,#43757,#43758,#43759,#43760),
 .UNSPECIFIED.,.F.,.F.,(4,3,3,3,3,3,3,3,3,3,3,3,3,3,3,3,3,3,3,3,3,3,3,3,
3,3,3,3,3,3,4),(2.55444286463925E-6,3.59894613493354E-5,0.0376304039226987,
0.0778196513591974,0.09090909090909,0.100015854684267,0.149597044039808,
0.1818181818182,0.20002307736844,0.252770096807691,0.2727272727273,0.300045132044768,
0.356511609189304,0.3636363636364,0.399993667063145,0.4545454545455,0.500004431078461,
0.5454545454545,0.600029859440393,0.6363636363636,0.696679386572962,0.699994555111378,
0.7272727272727,0.779840762831178,0.800031874864246,0.8181818181818,0.873862262978403,
0.899972577418814,0.9090909090909,0.961329494918914,1.),.UNSPECIFIED.);
#2402=B_SPLINE_CURVE_WITH_KNOTS('',3,(#43825,#43826,#43827,#43828,#43829,
#43830,#43831,#43832,#43833,#43834,#43835,#43836,#43837,#43838),
 .UNSPECIFIED.,.F.,.F.,(4,1,1,1,1,1,1,1,1,1,1,4),(1.1830067436204E-6,0.09090909090909,
0.1818181818182,0.2727272727273,0.3636363636364,0.4545454545455,0.5454545454545,
0.6363636363636,0.7272727272727,0.8181818181818,0.9090909090909,1.),
 .UNSPECIFIED.);
#2403=B_SPLINE_CURVE_WITH_KNOTS('',3,(#43906,#43907,#43908,#43909,#43910,
#43911,#43912,#43913,#43914,#43915,#43916,#43917,#43918,#43919,#43920,#43921,
#43922,#43923,#43924,#43925,#43926,#43927,#43928,#43929,#43930,#43931,#43932,
#43933,#43934,#43935,#43936,#43937,#43938,#43939,#43940,#43941,#43942,#43943,
#43944,#43945,#43946,#43947,#43948,#43949,#43950,#43951,#43952,#43953,#43954,
#43955,#43956,#43957,#43958,#43959,#43960,#43961,#43962,#43963,#43964,#43965,
#43966,#43967,#43968,#43969,#43970,#43971,#43972,#43973,#43974,#43975,#43976,
#43977,#43978,#43979,#43980,#43981,#43982,#43983,#43984,#43985,#43986,#43987,
#43988,#43989,#43990,#43991,#43992,#43993),.UNSPECIFIED.,.F.,.F.,(4,3,3,
3,3,3,3,3,3,3,3,3,3,3,3,3,3,3,3,3,3,3,3,3,3,3,3,3,3,4),(0.,0.0521094210463995,
0.09090909090909,0.100029793188817,0.155493160568291,0.1818181818182,0.199972986695707,
0.25252274815469,0.2727272727273,0.300015130565433,0.3636363636364,0.399976334120297,
0.4545454545455,0.50000649866054,0.5454545454545,0.600029082805183,0.6363636363636,
0.693010325114171,0.699967328272808,0.7272727272727,0.779887482806084,0.799997660318204,
0.8181818181818,0.86860586501179,0.900008800503424,0.9090909090909,0.949304252134719,
0.986777025421057,0.999997850420203,0.999998520519915),.UNSPECIFIED.);
#2404=B_SPLINE_CURVE_WITH_KNOTS('',3,(#43994,#43995,#43996,#43997,#43998,
#43999,#44000,#44001,#44002,#44003,#44004,#44005,#44006,#44007,#44008,#44009,
#44010,#44011,#44012,#44013,#44014,#44015,#44016,#44017,#44018,#44019,#44020,
#44021,#44022,#44023,#44024,#44025,#44026,#44027,#44028,#44029,#44030,#44031,
#44032,#44033,#44034,#44035,#44036,#44037,#44038,#44039,#44040,#44041,#44042,
#44043,#44044,#44045,#44046,#44047,#44048),.UNSPECIFIED.,.F.,.F.,(4,3,3,
3,3,3,3,3,3,3,3,3,3,3,3,3,3,3,4),(0.,0.09090909090909,0.1818181818182,0.2727272727273,
0.3636363636364,0.448887126274961,0.4545454545455,0.538390793737757,0.5454545454545,
0.620795104544488,0.6363636363636,0.70236319270021,0.7272727272727,0.792436576680819,
0.8181818181818,0.883253394758865,0.9090909090909,0.979516285384546,0.999999999997833),
 .UNSPECIFIED.);
#2405=B_SPLINE_CURVE_WITH_KNOTS('',3,(#44110,#44111,#44112,#44113,#44114,
#44115,#44116,#44117,#44118,#44119,#44120,#44121,#44122,#44123,#44124,#44125,
#44126,#44127,#44128,#44129,#44130,#44131,#44132,#44133,#44134),
 .UNSPECIFIED.,.F.,.F.,(4,3,3,3,3,3,3,3,4),(0.,0.125,0.25,0.375,0.5,0.625,
0.75,0.875,1.),.UNSPECIFIED.);
#2406=B_SPLINE_CURVE_WITH_KNOTS('',3,(#44137,#44138,#44139,#44140,#44141,
#44142,#44143,#44144,#44145,#44146,#44147,#44148,#44149,#44150,#44151,#44152,
#44153,#44154,#44155,#44156,#44157,#44158,#44159,#44160,#44161,#44162,#44163,
#44164),.UNSPECIFIED.,.F.,.F.,(4,3,3,3,3,3,3,3,3,4),(0.,0.1111111111111,
0.2222222222222,0.3333333333333,0.4444444444444,0.5555555555556,0.6666666666667,
0.7777777777778,0.8888888888889,0.999999995464213),.UNSPECIFIED.);
#2407=B_SPLINE_CURVE_WITH_KNOTS('',3,(#44250,#44251,#44252,#44253,#44254,
#44255,#44256,#44257,#44258,#44259,#44260,#44261,#44262,#44263,#44264,#44265,
#44266,#44267,#44268,#44269,#44270,#44271,#44272,#44273,#44274,#44275,#44276,
#44277,#44278,#44279,#44280,#44281,#44282,#44283,#44284,#44285,#44286,#44287,
#44288,#44289,#44290,#44291,#44292,#44293,#44294,#44295,#44296,#44297,#44298,
#44299,#44300,#44301,#44302,#44303,#44304,#44305,#44306,#44307,#44308,#44309,
#44310,#44311,#44312,#44313,#44314,#44315,#44316,#44317,#44318,#44319,#44320,
#44321,#44322,#44323,#44324,#44325,#44326,#44327,#44328,#44329,#44330,#44331,
#44332,#44333,#44334,#44335,#44336,#44337,#44338,#44339,#44340,#44341,#44342,
#44343,#44344,#44345,#44346,#44347,#44348,#44349,#44350,#44351,#44352,#44353,
#44354,#44355,#44356,#44357,#44358,#44359,#44360,#44361,#44362,#44363,#44364,
#44365,#44366,#44367),.UNSPECIFIED.,.F.,.F.,(4,3,3,3,3,3,3,3,3,3,3,3,3,
3,3,3,3,3,3,3,3,3,3,3,3,3,3,3,3,3,3,3,3,3,3,3,3,3,3,4),(2.86331152536071E-8,
0.0645615368166531,0.07142857142857,0.105823175263765,0.126783995341246,
0.1428571428571,0.196188267240046,0.2142857142857,0.245830118964743,0.276006551966036,
0.2857142857143,0.286907673257762,0.31962058114641,0.353834550293338,0.3571428571429,
0.410078570789993,0.420069072508489,0.4285714285714,0.485540140741139,0.5,
0.543491980185507,0.5714285714286,0.615772050421601,0.6428571428571,0.663598566580769,
0.696842541691307,0.7142857142857,0.746138463334994,0.777991212384288,0.7857142857143,
0.819589820812744,0.852305725672241,0.8571428571429,0.876162598148888,0.904048950216825,
0.9285714285714,0.952879545673236,0.963346746013781,0.986631905020373,1.),
 .UNSPECIFIED.);
#2408=B_SPLINE_CURVE_WITH_KNOTS('',3,(#44372,#44373,#44374,#44375,#44376,
#44377,#44378,#44379),.UNSPECIFIED.,.F.,.F.,(4,2,2,4),(1.00274854907622E-6,
0.034413002030414,0.062461027026842,0.0705842206571842),.UNSPECIFIED.);
#2409=B_SPLINE_CURVE_WITH_KNOTS('',3,(#44473,#44474,#44475,#44476,#44477,
#44478,#44479,#44480,#44481,#44482,#44483,#44484,#44485,#44486,#44487,#44488,
#44489,#44490,#44491,#44492,#44493,#44494,#44495),.UNSPECIFIED.,.F.,.F.,
(4,1,1,1,1,1,1,1,1,1,1,1,1,1,1,1,1,1,1,1,4),(0.,0.05,0.1,0.15,0.2,0.25,
0.3,0.35,0.4,0.45,0.5,0.55,0.6,0.65,0.7,0.75,0.8,0.85,0.9,0.95,1.),
 .UNSPECIFIED.);
#2410=B_SPLINE_CURVE_WITH_KNOTS('',3,(#44534,#44535,#44536,#44537,#44538,
#44539),.UNSPECIFIED.,.F.,.F.,(4,1,1,4),(0.,0.3333333333333,0.6666666666667,
1.),.UNSPECIFIED.);
#2411=B_SPLINE_CURVE_WITH_KNOTS('',3,(#44549,#44550,#44551,#44552,#44553,
#44554,#44555,#44556,#44557,#44558),.UNSPECIFIED.,.F.,.F.,(4,3,3,4),(0.,
0.3333333333333,0.6666666666667,1.),.UNSPECIFIED.);
#2412=B_SPLINE_CURVE_WITH_KNOTS('',3,(#44560,#44561,#44562,#44563,#44564,
#44565,#44566,#44567,#44568,#44569,#44570,#44571,#44572,#44573,#44574,#44575,
#44576,#44577,#44578,#44579,#44580,#44581,#44582,#44583,#44584,#44585,#44586,
#44587,#44588,#44589,#44590,#44591,#44592,#44593),.UNSPECIFIED.,.F.,.F.,
(4,3,3,3,3,3,3,3,3,3,3,4),(0.,0.128706181276151,0.2,0.32521503540555,0.4,
0.506081427734201,0.6,0.693453062106393,0.786170793391711,0.8,0.904195677401466,
0.99999863924574),.UNSPECIFIED.);
#2413=B_SPLINE_CURVE_WITH_KNOTS('',3,(#44595,#44596,#44597,#44598,#44599,
#44600,#44601,#44602,#44603,#44604,#44605,#44606,#44607,#44608,#44609,#44610,
#44611,#44612,#44613,#44614,#44615,#44616,#44617,#44618,#44619,#44620,#44621,
#44622,#44623,#44624,#44625,#44626,#44627,#44628,#44629,#44630,#44631,#44632,
#44633,#44634,#44635,#44636,#44637,#44638,#44639,#44640,#44641,#44642,#44643,
#44644,#44645,#44646,#44647,#44648,#44649,#44650,#44651,#44652,#44653,#44654,
#44655,#44656,#44657,#44658,#44659,#44660,#44661,#44662,#44663,#44664,#44665,
#44666,#44667),.UNSPECIFIED.,.F.,.F.,(4,3,3,3,3,3,3,3,3,3,3,3,3,3,3,3,3,
3,3,3,3,3,3,3,4),(0.,0.05555555555555,0.106924267986465,0.1111111111111,
0.161796567291066,0.212394385898786,0.2222222222222,0.27465541537399,0.327511260060941,
0.3333333333333,0.389820070129939,0.4444444444444,0.503505530229127,0.5555555555556,
0.612328691897827,0.6666666666667,0.72222222222225,0.774969127013547,0.7777777777778,
0.82835260149752,0.87870895459855,0.8888888888889,0.941118027379493,0.996727628424779,
1.),.UNSPECIFIED.);
#2414=B_SPLINE_CURVE_WITH_KNOTS('',3,(#44668,#44669,#44670,#44671,#44672,
#44673,#44674,#44675,#44676,#44677,#44678,#44679,#44680,#44681,#44682,#44683,
#44684,#44685,#44686,#44687,#44688,#44689,#44690,#44691,#44692,#44693,#44694,
#44695,#44696,#44697,#44698,#44699,#44700,#44701,#44702,#44703,#44704,#44705,
#44706,#44707,#44708,#44709,#44710,#44711,#44712,#44713,#44714,#44715,#44716),
 .UNSPECIFIED.,.F.,.F.,(4,3,3,3,3,3,3,3,3,3,3,3,3,3,3,3,4),(4.33800647388095E-8,
0.115672156634637,0.179199191820932,0.2,0.292238719088017,0.378853944193901,
0.384477438176035,0.4,0.504607292126722,0.589623488819915,0.6,0.691024217930037,
0.782473470110827,0.794807707256916,0.8,0.903113049573187,0.999999723429614),
 .UNSPECIFIED.);
#2415=B_SPLINE_CURVE_WITH_KNOTS('',3,(#44754,#44755,#44756,#44757,#44758,
#44759,#44760,#44761,#44762,#44763,#44764,#44765,#44766,#44767,#44768,#44769,
#44770,#44771,#44772,#44773,#44774,#44775,#44776,#44777,#44778,#44779,#44780,
#44781,#44782,#44783,#44784,#44785,#44786,#44787,#44788,#44789,#44790,#44791,
#44792,#44793,#44794,#44795,#44796),.UNSPECIFIED.,.F.,.F.,(4,3,3,3,3,3,
3,3,3,3,3,3,3,3,4),(1.02489136070401E-6,2.78892909788713E-6,0.0898895600139057,
0.1666666666667,0.16666735661307,0.250000344973185,0.3333333333333,0.460510299335861,
0.5,0.60992454588341,0.6666666666667,0.778760920788974,0.8333333333333,
0.964311512862908,0.999999944055817),.UNSPECIFIED.);
#2416=B_SPLINE_CURVE_WITH_KNOTS('',3,(#44884,#44885,#44886,#44887,#44888,
#44889,#44890,#44891,#44892,#44893,#44894,#44895,#44896,#44897,#44898,#44899,
#44900,#44901,#44902,#44903,#44904,#44905,#44906,#44907,#44908,#44909,#44910,
#44911,#44912,#44913,#44914),.UNSPECIFIED.,.F.,.F.,(4,3,3,3,3,3,3,3,3,3,
4),(0.,0.2,0.4,0.6,0.600006275012996,0.721742469521887,0.799981987265399,
0.8,0.912452142717923,0.999991024190224,1.),.UNSPECIFIED.);
#2417=B_SPLINE_CURVE_WITH_KNOTS('',3,(#44975,#44976,#44977,#44978,#44979,
#44980,#44981,#44982,#44983,#44984,#44985,#44986,#44987,#44988,#44989,#44990,
#44991,#44992,#44993,#44994,#44995,#44996,#44997,#44998,#44999,#45000,#45001,
#45002,#45003,#45004,#45005),.UNSPECIFIED.,.F.,.F.,(4,3,3,3,3,3,3,3,3,3,
4),(4.98087268739273E-6,0.149736166300919,0.2,0.315183284203544,0.4,0.403962239763029,
0.6,0.768315918661213,0.8,0.880495757642992,1.),.UNSPECIFIED.);
#2418=B_SPLINE_CURVE_WITH_KNOTS('',3,(#45006,#45007,#45008,#45009,#45010,
#45011,#45012,#45013,#45014,#45015,#45016,#45017,#45018,#45019,#45020,#45021,
#45022,#45023,#45024,#45025,#45026,#45027,#45028,#45029,#45030,#45031,#45032,
#45033,#45034,#45035,#45036,#45037,#45038,#45039,#45040,#45041,#45042,#45043,
#45044,#45045,#45046,#45047,#45048,#45049,#45050,#45051,#45052,#45053,#45054,
#45055,#45056,#45057,#45058,#45059,#45060,#45061,#45062,#45063),
 .UNSPECIFIED.,.F.,.F.,(4,3,3,3,3,3,3,3,3,3,3,3,3,3,3,3,3,3,3,4),(0.,0.0785005850502826,
0.1428571428571,0.152289983519359,0.224965657458616,0.2857142857143,0.365357998177071,
0.4285714285714,0.495413593720157,0.562079339149973,0.5714285714286,0.58250627313346,
0.653487828717598,0.7142857142857,0.774274923856638,0.815018706983836,0.8571428571429,
0.924946709565138,0.992791568957691,1.),.UNSPECIFIED.);
#2419=B_SPLINE_CURVE_WITH_KNOTS('',3,(#45114,#45115,#45116,#45117,#45118,
#45119,#45120,#45121,#45122,#45123,#45124,#45125,#45126,#45127,#45128,#45129,
#45130,#45131,#45132,#45133,#45134,#45135,#45136,#45137,#45138,#45139,#45140,
#45141,#45142,#45143,#45144,#45145,#45146,#45147,#45148,#45149,#45150,#45151,
#45152,#45153,#45154,#45155,#45156,#45157,#45158,#45159,#45160,#45161,#45162,
#45163,#45164,#45165,#45166,#45167,#45168,#45169,#45170,#45171,#45172,#45173,
#45174,#45175,#45176,#45177,#45178,#45179,#45180),.UNSPECIFIED.,.F.,.F.,
(4,3,3,3,3,3,3,3,3,3,3,3,3,3,3,3,3,3,3,3,3,3,4),(1.52199927505013E-7,0.0615976282481722,
0.123466697458492,0.1428571428571,0.198336877388203,0.254197653065242,0.2857142857143,
0.351407196402381,0.416990445187705,0.4285714285714,0.476573915420894,0.524965880688773,
0.5714285714286,0.627091486629155,0.684253122670088,0.7142857142857,0.759626312948552,
0.804674497897221,0.848776226530048,0.8571428571429,0.911252892719779,0.96436009832331,
1.),.UNSPECIFIED.);
#2420=B_SPLINE_CURVE_WITH_KNOTS('',3,(#45325,#45326,#45327,#45328,#45329,
#45330,#45331,#45332,#45333,#45334,#45335,#45336,#45337,#45338,#45339,#45340,
#45341,#45342,#45343,#45344,#45345,#45346,#45347,#45348,#45349,#45350,#45351,
#45352,#45353,#45354,#45355,#45356,#45357,#45358,#45359,#45360,#45361,#45362,
#45363,#45364,#45365,#45366,#45367,#45368,#45369,#45370,#45371,#45372,#45373,
#45374,#45375,#45376,#45377,#45378,#45379,#45380,#45381,#45382,#45383,#45384,
#45385,#45386,#45387,#45388,#45389,#45390,#45391,#45392,#45393,#45394,#45395,
#45396,#45397,#45398,#45399,#45400,#45401,#45402,#45403,#45404,#45405,#45406,
#45407,#45408,#45409,#45410,#45411,#45412,#45413,#45414,#45415,#45416,#45417,
#45418,#45419,#45420,#45421,#45422,#45423,#45424,#45425,#45426,#45427,#45428,
#45429,#45430),.UNSPECIFIED.,.F.,.F.,(4,3,3,3,3,3,3,3,3,3,3,3,3,3,3,3,3,
3,3,3,3,3,3,3,3,3,3,3,3,3,3,3,3,3,3,4),(4.07533832038655E-8,0.0285863583342577,
0.0561745109866684,0.07142857142857,0.103500023873821,0.136613116776887,
0.1428571428571,0.164726875357122,0.203610380996657,0.2142857142857,0.255318345978842,
0.281307398781265,0.2857142857143,0.330530146034011,0.3571428571429,0.40506357525368,
0.414638109539121,0.4285714285714,0.4808296111022,0.5,0.549245837571629,
0.5714285714286,0.572143480381714,0.627101769658719,0.6428571428571,0.7102100620386,
0.7142857142857,0.742403038961964,0.7857142857143,0.839203130289171,0.8571428571429,
0.898082398123236,0.920731769414707,0.9285714285714,0.977975463981205,0.999993896438902),
 .UNSPECIFIED.);
#2421=B_SPLINE_CURVE_WITH_KNOTS('',3,(#45432,#45433,#45434,#45435,#45436,
#45437,#45438,#45439),.UNSPECIFIED.,.F.,.F.,(4,2,2,4),(-0.0527156059695698,
-0.0448511032213948,-0.0273145742577129,0.),.UNSPECIFIED.);
#2422=B_SPLINE_CURVE_WITH_KNOTS('',3,(#45514,#45515,#45516,#45517,#45518,
#45519,#45520,#45521,#45522,#45523,#45524,#45525,#45526,#45527),
 .UNSPECIFIED.,.F.,.F.,(4,2,2,2,2,2,4),(2.91925194763159E-6,0.0934696392563499,
0.166869193276301,0.18008495547347,0.185834312297566,0.188453342685018,
0.190941477315289),.UNSPECIFIED.);
#2423=B_SPLINE_CURVE_WITH_KNOTS('',3,(#45538,#45539,#45540,#45541,#45542,
#45543,#45544,#45545,#45546,#45547,#45548,#45549,#45550,#45551,#45552,#45553,
#45554,#45555,#45556,#45557,#45558,#45559,#45560,#45561,#45562,#45563,#45564,
#45565,#45566,#45567,#45568,#45569,#45570,#45571,#45572,#45573,#45574,#45575,
#45576,#45577,#45578,#45579,#45580,#45581,#45582,#45583,#45584,#45585,#45586,
#45587,#45588,#45589,#45590,#45591,#45592),.UNSPECIFIED.,.F.,.F.,(4,3,3,
3,3,3,3,3,3,3,3,3,3,3,3,3,3,3,4),(0.,0.0590659964221531,0.118210774712157,
0.125,0.215580128193309,0.25,0.3125,0.375,0.4375,0.5,0.606604025388335,
0.625,0.6875,0.75,0.805504989390552,0.860991155263171,0.875,0.943021966926566,
1.),.UNSPECIFIED.);
#2424=B_SPLINE_CURVE_WITH_KNOTS('',3,(#45648,#45649,#45650,#45651,#45652,
#45653,#45654,#45655,#45656,#45657,#45658,#45659,#45660,#45661,#45662,#45663,
#45664,#45665,#45666,#45667,#45668,#45669,#45670,#45671,#45672,#45673,#45674,
#45675,#45676,#45677,#45678,#45679,#45680,#45681,#45682,#45683,#45684,#45685,
#45686,#45687,#45688,#45689,#45690,#45691,#45692,#45693,#45694,#45695,#45696,
#45697,#45698,#45699,#45700,#45701,#45702,#45703,#45704,#45705),
 .UNSPECIFIED.,.F.,.F.,(4,3,3,3,3,3,3,3,3,3,3,3,3,3,3,3,3,3,3,4),(0.,0.000317629015129917,
0.0773853855433874,0.125,0.17861003880418,0.232539979538112,0.25,0.328925013375417,
0.375,0.46719173907792,0.5,0.563115540635534,0.625,0.706667897106718,0.75,
0.826211882215789,0.875,0.945358955314075,0.99986711918626,1.),
 .UNSPECIFIED.);
#2425=B_SPLINE_CURVE_WITH_KNOTS('',3,(#45824,#45825,#45826,#45827,#45828,
#45829,#45830,#45831,#45832,#45833,#45834,#45835,#45836,#45837,#45838,#45839,
#45840,#45841,#45842,#45843,#45844,#45845,#45846,#45847,#45848,#45849,#45850,
#45851,#45852,#45853,#45854,#45855,#45856,#45857,#45858,#45859,#45860,#45861,
#45862,#45863,#45864,#45865,#45866,#45867,#45868,#45869,#45870,#45871,#45872,
#45873,#45874,#45875,#45876,#45877,#45878,#45879,#45880,#45881,#45882,#45883,
#45884,#45885,#45886,#45887),.UNSPECIFIED.,.F.,.F.,(4,3,3,3,3,3,3,3,3,3,
3,3,3,3,3,3,3,3,3,3,3,4),(1.1164216272441E-6,1.64886277366089E-6,0.0294346969467261,
0.0615346142090942,0.07142857142857,0.122235287796492,0.1428571428571,0.2142857142857,
0.2857142857143,0.3571428571429,0.4285714285714,0.5,0.5714285714286,0.6428571428571,
0.7142857142857,0.7857142857143,0.842909114801495,0.8571428571429,0.904173100246843,
0.9285714285714,0.993096032114401,1.),.UNSPECIFIED.);
#2426=B_SPLINE_CURVE_WITH_KNOTS('',3,(#45889,#45890,#45891,#45892,#45893,
#45894,#45895,#45896,#45897,#45898,#45899,#45900,#45901,#45902,#45903,#45904,
#45905,#45906,#45907,#45908,#45909,#45910,#45911,#45912,#45913,#45914,#45915,
#45916,#45917,#45918,#45919,#45920,#45921,#45922,#45923,#45924,#45925,#45926,
#45927,#45928,#45929,#45930,#45931,#45932,#45933,#45934,#45935,#45936,#45937,
#45938,#45939,#45940),.UNSPECIFIED.,.F.,.F.,(4,3,3,3,3,3,3,3,3,3,3,3,3,
3,3,3,3,4),(8.6778036994424E-7,0.0586819159367273,0.07142857142857,0.1428571428571,
0.2142857142857,0.2857142857143,0.3571428571429,0.4285714285714,0.5,0.5714285714286,
0.6428571428571,0.7142857142857,0.7857142857143,0.8571428571429,0.920068145469386,
0.9285714285714,0.994698303801108,1.),.UNSPECIFIED.);
#2427=B_SPLINE_CURVE_WITH_KNOTS('',3,(#46022,#46023,#46024,#46025,#46026,
#46027,#46028,#46029),.UNSPECIFIED.,.F.,.F.,(4,1,1,1,1,4),(8.18300672274726E-6,
0.2,0.4,0.6,0.8,1.),.UNSPECIFIED.);
#2826=LINE('',#39902,#3291);
#2827=LINE('',#39904,#3292);
#2828=LINE('',#39906,#3293);
#2829=LINE('',#39920,#3294);
#2830=LINE('',#39933,#3295);
#2831=LINE('',#39942,#3296);
#2832=LINE('',#39947,#3297);
#2833=LINE('',#39970,#3298);
#2834=LINE('',#40327,#3299);
#2835=LINE('',#40513,#3300);
#2836=LINE('',#40660,#3301);
#2837=LINE('',#40913,#3302);
#2838=LINE('',#41165,#3303);
#2839=LINE('',#41597,#3304);
#2840=LINE('',#42029,#3305);
#2841=LINE('',#42391,#3306);
#2842=LINE('',#43224,#3307);
#2843=LINE('',#43377,#3308);
#2844=LINE('',#43431,#3309);
#2845=LINE('',#43600,#3310);
#2846=LINE('',#43632,#3311);
#2847=LINE('',#43634,#3312);
#2848=LINE('',#43640,#3313);
#2849=LINE('',#43644,#3314);
#2850=LINE('',#43649,#3315);
#2851=LINE('',#43655,#3316);
#2852=LINE('',#43659,#3317);
#2853=LINE('',#43663,#3318);
#2854=LINE('',#43669,#3319);
#2855=LINE('',#44053,#3320);
#2856=LINE('',#44054,#3321);
#2857=LINE('',#44060,#3322);
#2858=LINE('',#44064,#3323);
#2859=LINE('',#44065,#3324);
#2860=LINE('',#44073,#3325);
#2861=LINE('',#44078,#3326);
#2862=LINE('',#44081,#3327);
#2863=LINE('',#44085,#3328);
#2864=LINE('',#44096,#3329);
#2865=LINE('',#44099,#3330);
#2866=LINE('',#44104,#3331);
#2867=LINE('',#44108,#3332);
#2868=LINE('',#44136,#3333);
#2869=LINE('',#44499,#3334);
#2870=LINE('',#44543,#3335);
#2871=LINE('',#44547,#3336);
#2872=LINE('',#45184,#3337);
#2873=LINE('',#45200,#3338);
#2874=LINE('',#45202,#3339);
#2875=LINE('',#45205,#3340);
#2876=LINE('',#45211,#3341);
#2877=LINE('',#45218,#3342);
#2878=LINE('',#45219,#3343);
#2879=LINE('',#45225,#3344);
#2880=LINE('',#45229,#3345);
#2881=LINE('',#45232,#3346);
#2882=LINE('',#45233,#3347);
#2883=LINE('',#45235,#3348);
#2884=LINE('',#45236,#3349);
#2885=LINE('',#45240,#3350);
#2886=LINE('',#45241,#3351);
#2887=LINE('',#45532,#3352);
#2888=LINE('',#45533,#3353);
#2889=LINE('',#45534,#3354);
#2890=LINE('',#45593,#3355);
#2891=LINE('',#45708,#3356);
#2892=LINE('',#45710,#3357);
#2893=LINE('',#46032,#3358);
#2894=LINE('',#46033,#3359);
#3291=VECTOR('',#12002,8.999999999839);
#3292=VECTOR('',#12003,15.48856626783);
#3293=VECTOR('',#12004,5.09731398179822);
#3294=VECTOR('',#12005,2.18647853617101);
#3295=VECTOR('',#12022,5.);
#3296=VECTOR('',#12033,4.);
#3297=VECTOR('',#12038,4.);
#3298=VECTOR('',#12039,0.75);
#3299=VECTOR('',#12042,0.461880215351696);
#3300=VECTOR('',#12043,0.461880215351696);
#3301=VECTOR('',#12044,0.2881197846483);
#3302=VECTOR('',#12045,0.2881197846483);
#3303=VECTOR('',#12046,0.461880215351696);
#3304=VECTOR('',#12047,0.461880215351696);
#3305=VECTOR('',#12048,0.461880215351684);
#3306=VECTOR('',#12049,0.461880215351684);
#3307=VECTOR('',#12050,0.2881197846483);
#3308=VECTOR('',#12059,6.);
#3309=VECTOR('',#12068,6.75);
#3310=VECTOR('',#12073,2.473089489284);
#3311=VECTOR('',#12074,15.15835238946);
#3312=VECTOR('',#12075,10.99999999936);
#3313=VECTOR('',#12080,4.78408308320006);
#3314=VECTOR('',#12083,4.78408308319393);
#3315=VECTOR('',#12088,2.22834709131601);
#3316=VECTOR('',#12095,1.25);
#3317=VECTOR('',#12098,3.38573837870217);
#3318=VECTOR('',#12101,3.38573819298811);
#3319=VECTOR('',#12108,4.78408308337184);
#3320=VECTOR('',#12125,1.5);
#3321=VECTOR('',#12126,1.5);
#3322=VECTOR('',#12135,4.78408308309884);
#3323=VECTOR('',#12140,1.5);
#3324=VECTOR('',#12141,4.78408308336584);
#3325=VECTOR('',#12154,1.5);
#3326=VECTOR('',#12161,4.78408308310784);
#3327=VECTOR('',#12166,1.5);
#3328=VECTOR('',#12171,1.5);
#3329=VECTOR('',#12186,8.85);
#3330=VECTOR('',#12189,8.85);
#3331=VECTOR('',#12196,2.22834723186102);
#3332=VECTOR('',#12201,2.18647846971201);
#3333=VECTOR('',#12202,3.745592232445);
#3334=VECTOR('',#12211,2.459549577106);
#3335=VECTOR('',#12218,8.13705833981064);
#3336=VECTOR('',#12221,8.16003640112219);
#3337=VECTOR('',#12236,15.16332099539);
#3338=VECTOR('',#12245,11.);
#3339=VECTOR('',#12246,5.85);
#3340=VECTOR('',#12249,8.999999999998);
#3341=VECTOR('',#12256,3.6);
#3342=VECTOR('',#12265,3.23);
#3343=VECTOR('',#12266,3.23);
#3344=VECTOR('',#12271,2.503692708007);
#3345=VECTOR('',#12274,2.453282759045);
#3346=VECTOR('',#12277,2.450330288028);
#3347=VECTOR('',#12278,2.494111584205);
#3348=VECTOR('',#12281,7.36244219026491);
#3349=VECTOR('',#12282,7.35020412958116);
#3350=VECTOR('',#12287,3.745592232442);
#3351=VECTOR('',#12288,7.31329808179909);
#3352=VECTOR('',#12301,5.10538702111419);
#3353=VECTOR('',#12302,8.10150600096205);
#3354=VECTOR('',#12303,7.22099758100766);
#3355=VECTOR('',#12308,8.10459673698465);
#3356=VECTOR('',#12315,3.838901255888);
#3357=VECTOR('',#12316,3.83784463984698);
#3358=VECTOR('',#12329,5.849999999044);
#3359=VECTOR('',#12330,15.49166557366);
#4065=VERTEX_POINT('',#39900);
#4066=VERTEX_POINT('',#39901);
#4067=VERTEX_POINT('',#39903);
#4068=VERTEX_POINT('',#39905);
#4069=VERTEX_POINT('',#39907);
#4070=VERTEX_POINT('',#39919);
#4071=VERTEX_POINT('',#39922);
#4072=VERTEX_POINT('',#39925);
#4073=VERTEX_POINT('',#39926);
#4074=VERTEX_POINT('',#39931);
#4075=VERTEX_POINT('',#39935);
#4076=VERTEX_POINT('',#39938);
#4077=VERTEX_POINT('',#39939);
#4078=VERTEX_POINT('',#39944);
#4079=VERTEX_POINT('',#39946);
#4080=VERTEX_POINT('',#39948);
#4081=VERTEX_POINT('',#39969);
#4082=VERTEX_POINT('',#40066);
#4083=VERTEX_POINT('',#40081);
#4084=VERTEX_POINT('',#40275);
#4085=VERTEX_POINT('',#40326);
#4086=VERTEX_POINT('',#40328);
#4087=VERTEX_POINT('',#40337);
#4088=VERTEX_POINT('',#40444);
#4089=VERTEX_POINT('',#40473);
#4090=VERTEX_POINT('',#40512);
#4091=VERTEX_POINT('',#40801);
#4092=VERTEX_POINT('',#40912);
#4093=VERTEX_POINT('',#41164);
#4094=VERTEX_POINT('',#41486);
#4095=VERTEX_POINT('',#41738);
#4096=VERTEX_POINT('',#41917);
#4097=VERTEX_POINT('',#42028);
#4098=VERTEX_POINT('',#42280);
#4099=VERTEX_POINT('',#42532);
#4100=VERTEX_POINT('',#42967);
#4101=VERTEX_POINT('',#43373);
#4102=VERTEX_POINT('',#43376);
#4103=VERTEX_POINT('',#43379);
#4104=VERTEX_POINT('',#43380);
#4105=VERTEX_POINT('',#43427);
#4106=VERTEX_POINT('',#43430);
#4107=VERTEX_POINT('',#43434);
#4108=VERTEX_POINT('',#43435);
#4109=VERTEX_POINT('',#43599);
#4110=VERTEX_POINT('',#43601);
#4111=VERTEX_POINT('',#43612);
#4112=VERTEX_POINT('',#43622);
#4113=VERTEX_POINT('',#43631);
#4114=VERTEX_POINT('',#43633);
#4115=VERTEX_POINT('',#43635);
#4116=VERTEX_POINT('',#43637);
#4117=VERTEX_POINT('',#43639);
#4118=VERTEX_POINT('',#43641);
#4119=VERTEX_POINT('',#43643);
#4120=VERTEX_POINT('',#43645);
#4121=VERTEX_POINT('',#43647);
#4122=VERTEX_POINT('',#43650);
#4123=VERTEX_POINT('',#43653);
#4124=VERTEX_POINT('',#43657);
#4125=VERTEX_POINT('',#43658);
#4126=VERTEX_POINT('',#43660);
#4127=VERTEX_POINT('',#43662);
#4128=VERTEX_POINT('',#43666);
#4129=VERTEX_POINT('',#43668);
#4130=VERTEX_POINT('',#43821);
#4131=VERTEX_POINT('',#43823);
#4132=VERTEX_POINT('',#43840);
#4133=VERTEX_POINT('',#43903);
#4134=VERTEX_POINT('',#43904);
#4135=VERTEX_POINT('',#44050);
#4136=VERTEX_POINT('',#44051);
#4137=VERTEX_POINT('',#44059);
#4138=VERTEX_POINT('',#44063);
#4139=VERTEX_POINT('',#44071);
#4140=VERTEX_POINT('',#44077);
#4141=VERTEX_POINT('',#44083);
#4142=VERTEX_POINT('',#44089);
#4143=VERTEX_POINT('',#44093);
#4144=VERTEX_POINT('',#44095);
#4145=VERTEX_POINT('',#44097);
#4146=VERTEX_POINT('',#44103);
#4147=VERTEX_POINT('',#44107);
#4148=VERTEX_POINT('',#44109);
#4149=VERTEX_POINT('',#44135);
#4150=VERTEX_POINT('',#44249);
#4151=VERTEX_POINT('',#44368);
#4152=VERTEX_POINT('',#44370);
#4153=VERTEX_POINT('',#44472);
#4154=VERTEX_POINT('',#44498);
#4155=VERTEX_POINT('',#44533);
#4156=VERTEX_POINT('',#44542);
#4157=VERTEX_POINT('',#44544);
#4158=VERTEX_POINT('',#44546);
#4159=VERTEX_POINT('',#44548);
#4160=VERTEX_POINT('',#44559);
#4161=VERTEX_POINT('',#44594);
#4162=VERTEX_POINT('',#44753);
#4163=VERTEX_POINT('',#44883);
#4164=VERTEX_POINT('',#44972);
#4165=VERTEX_POINT('',#44974);
#4166=VERTEX_POINT('',#45112);
#4167=VERTEX_POINT('',#45182);
#4168=VERTEX_POINT('',#45194);
#4169=VERTEX_POINT('',#45195);
#4170=VERTEX_POINT('',#45201);
#4171=VERTEX_POINT('',#45203);
#4172=VERTEX_POINT('',#45206);
#4173=VERTEX_POINT('',#45209);
#4174=VERTEX_POINT('',#45213);
#4175=VERTEX_POINT('',#45216);
#4176=VERTEX_POINT('',#45221);
#4177=VERTEX_POINT('',#45222);
#4178=VERTEX_POINT('',#45224);
#4179=VERTEX_POINT('',#45226);
#4180=VERTEX_POINT('',#45228);
#4181=VERTEX_POINT('',#45230);
#4182=VERTEX_POINT('',#45239);
#4183=VERTEX_POINT('',#45324);
#4184=VERTEX_POINT('',#45431);
#4185=VERTEX_POINT('',#45513);
#4186=VERTEX_POINT('',#45531);
#4187=VERTEX_POINT('',#45537);
#4188=VERTEX_POINT('',#45647);
#4189=VERTEX_POINT('',#45709);
#4190=VERTEX_POINT('',#45745);
#4191=VERTEX_POINT('',#45888);
#4192=VERTEX_POINT('',#46031);
#5312=EDGE_CURVE('',#4065,#4066,#2826,.T.);
#5313=EDGE_CURVE('',#4065,#4067,#2827,.T.);
#5314=EDGE_CURVE('',#4068,#4067,#2828,.T.);
#5315=EDGE_CURVE('',#4069,#4068,#2368,.T.);
#5316=EDGE_CURVE('',#4070,#4069,#2829,.T.);
#5317=EDGE_CURVE('',#4066,#4070,#1993,.T.);
#5318=EDGE_CURVE('',#4071,#4071,#1994,.T.);
#5319=EDGE_CURVE('',#4072,#4073,#1995,.T.);
#5320=EDGE_CURVE('',#4073,#4072,#1996,.T.);
#5321=EDGE_CURVE('',#4073,#4071,#1997,.T.);
#5322=EDGE_CURVE('',#4074,#4074,#1998,.T.);
#5323=EDGE_CURVE('',#4074,#4072,#2830,.T.);
#5324=EDGE_CURVE('',#4075,#4075,#1999,.T.);
#5325=EDGE_CURVE('',#4076,#4077,#2000,.T.);
#5326=EDGE_CURVE('',#4077,#4076,#2001,.T.);
#5327=EDGE_CURVE('',#4077,#4075,#2831,.T.);
#5328=EDGE_CURVE('',#4078,#4078,#2002,.T.);
#5329=EDGE_CURVE('',#4078,#4079,#2832,.T.);
#5330=EDGE_CURVE('',#4080,#4079,#2369,.F.);
#5331=EDGE_CURVE('',#4081,#4080,#2833,.T.);
#5332=EDGE_CURVE('',#4079,#4081,#2370,.F.);
#5333=EDGE_CURVE('',#4076,#4082,#2371,.T.);
#5334=EDGE_CURVE('',#4083,#4076,#2372,.T.);
#5335=EDGE_CURVE('',#4082,#4083,#2373,.T.);
#5336=EDGE_CURVE('',#4082,#4084,#2374,.T.);
#5337=EDGE_CURVE('',#4085,#4084,#2834,.T.);
#5338=EDGE_CURVE('',#4086,#4085,#2375,.T.);
#5339=EDGE_CURVE('',#4087,#4086,#2376,.T.);
#5340=EDGE_CURVE('',#4076,#4087,#2377,.T.);
#5341=EDGE_CURVE('',#4085,#4088,#2378,.T.);
#5342=EDGE_CURVE('',#4089,#4088,#2379,.F.);
#5343=EDGE_CURVE('',#4090,#4089,#2835,.T.);
#5344=EDGE_CURVE('',#4083,#4090,#2380,.T.);
#5345=EDGE_CURVE('',#4084,#4090,#2836,.T.);
#5346=EDGE_CURVE('',#4090,#4091,#2381,.T.);
#5347=EDGE_CURVE('',#4092,#4091,#2837,.T.);
#5348=EDGE_CURVE('',#4084,#4092,#2382,.T.);
#5349=EDGE_CURVE('',#4093,#4092,#2838,.T.);
#5350=EDGE_CURVE('',#4089,#4093,#2383,.F.);
#5351=EDGE_CURVE('',#4093,#4094,#2384,.T.);
#5352=EDGE_CURVE('',#4091,#4094,#2839,.T.);
#5353=EDGE_CURVE('',#4094,#4095,#2385,.T.);
#5354=EDGE_CURVE('',#4095,#4096,#2386,.T.);
#5355=EDGE_CURVE('',#4097,#4096,#2840,.T.);
#5356=EDGE_CURVE('',#4091,#4097,#2387,.T.);
#5357=EDGE_CURVE('',#4092,#4098,#2388,.T.);
#5358=EDGE_CURVE('',#4095,#4098,#2841,.T.);
#5359=EDGE_CURVE('',#4098,#4099,#2389,.T.);
#5360=EDGE_CURVE('',#4080,#4099,#2390,.T.);
#5361=EDGE_CURVE('',#4096,#4080,#2391,.F.);
#5362=EDGE_CURVE('',#4100,#4081,#2392,.T.);
#5363=EDGE_CURVE('',#4097,#4100,#2393,.T.);
#5364=EDGE_CURVE('',#4098,#4097,#2842,.T.);
#5365=EDGE_CURVE('',#4099,#4100,#2394,.T.);
#5366=EDGE_CURVE('',#4101,#4101,#2003,.T.);
#5367=EDGE_CURVE('',#4101,#4102,#2843,.T.);
#5368=EDGE_CURVE('',#4102,#4102,#2004,.T.);
#5369=EDGE_CURVE('',#4103,#4104,#2395,.T.);
#5370=EDGE_CURVE('',#4104,#4103,#2396,.T.);
#5371=EDGE_CURVE('',#4105,#4105,#2005,.T.);
#5372=EDGE_CURVE('',#4105,#4106,#2844,.T.);
#5373=EDGE_CURVE('',#4106,#4106,#2006,.T.);
#5374=EDGE_CURVE('',#4107,#4108,#2397,.T.);
#5375=EDGE_CURVE('',#4109,#4107,#2845,.T.);
#5376=EDGE_CURVE('',#4110,#4109,#2398,.T.);
#5377=EDGE_CURVE('',#4111,#4110,#2399,.T.);
#5378=EDGE_CURVE('',#4112,#4111,#2400,.T.);
#5379=EDGE_CURVE('',#4113,#4112,#2846,.T.);
#5380=EDGE_CURVE('',#4114,#4113,#2847,.T.);
#5381=EDGE_CURVE('',#4115,#4114,#2007,.T.);
#5382=EDGE_CURVE('',#4116,#4115,#2008,.T.);
#5383=EDGE_CURVE('',#4117,#4116,#2848,.T.);
#5384=EDGE_CURVE('',#4118,#4117,#2009,.T.);
#5385=EDGE_CURVE('',#4119,#4118,#2849,.T.);
#5386=EDGE_CURVE('',#4120,#4119,#2010,.T.);
#5387=EDGE_CURVE('',#4121,#4120,#2011,.T.);
#5388=EDGE_CURVE('',#4108,#4121,#2850,.T.);
#5389=EDGE_CURVE('',#4122,#4122,#2012,.T.);
#5390=EDGE_CURVE('',#4123,#4123,#2013,.T.);
#5391=EDGE_CURVE('',#4123,#4122,#2851,.T.);
#5392=EDGE_CURVE('',#4124,#4125,#2852,.T.);
#5393=EDGE_CURVE('',#4125,#4126,#2014,.T.);
#5394=EDGE_CURVE('',#4126,#4127,#2853,.T.);
#5395=EDGE_CURVE('',#4127,#4124,#2015,.T.);
#5396=EDGE_CURVE('',#4124,#4128,#2016,.T.);
#5397=EDGE_CURVE('',#4129,#4128,#2854,.T.);
#5398=EDGE_CURVE('',#4125,#4129,#2401,.T.);
#5399=EDGE_CURVE('',#4125,#4130,#2017,.T.);
#5400=EDGE_CURVE('',#4129,#4131,#2018,.T.);
#5401=EDGE_CURVE('',#4130,#4131,#2402,.T.);
#5402=EDGE_CURVE('',#4126,#4132,#2019,.T.);
#5403=EDGE_CURVE('',#4130,#4132,#2020,.T.);
#5404=EDGE_CURVE('',#4133,#4134,#2021,.T.);
#5405=EDGE_CURVE('',#4133,#4126,#2403,.T.);
#5406=EDGE_CURVE('',#4134,#4132,#2404,.T.);
#5407=EDGE_CURVE('',#4135,#4136,#2022,.T.);
#5408=EDGE_CURVE('',#4136,#4133,#2855,.T.);
#5409=EDGE_CURVE('',#4134,#4135,#2856,.T.);
#5410=EDGE_CURVE('',#4135,#4120,#2023,.T.);
#5411=EDGE_CURVE('',#4136,#4119,#2024,.T.);
#5412=EDGE_CURVE('',#4136,#4137,#2857,.T.);
#5413=EDGE_CURVE('',#4137,#4118,#2025,.T.);
#5414=EDGE_CURVE('',#4137,#4138,#2858,.T.);
#5415=EDGE_CURVE('',#4138,#4133,#2859,.T.);
#5416=EDGE_CURVE('',#4127,#4138,#2026,.T.);
#5417=EDGE_CURVE('',#4138,#4128,#2027,.T.);
#5418=EDGE_CURVE('',#4137,#4139,#2028,.T.);
#5419=EDGE_CURVE('',#4139,#4128,#2860,.T.);
#5420=EDGE_CURVE('',#4139,#4117,#2029,.T.);
#5421=EDGE_CURVE('',#4139,#4140,#2861,.T.);
#5422=EDGE_CURVE('',#4140,#4116,#2030,.T.);
#5423=EDGE_CURVE('',#4129,#4140,#2862,.T.);
#5424=EDGE_CURVE('',#4140,#4141,#2031,.T.);
#5425=EDGE_CURVE('',#4141,#4131,#2863,.T.);
#5426=EDGE_CURVE('',#4141,#4115,#2032,.T.);
#5427=EDGE_CURVE('',#4141,#4142,#2033,.T.);
#5428=EDGE_CURVE('',#4142,#4114,#2034,.T.);
#5429=EDGE_CURVE('',#4143,#4135,#2035,.T.);
#5430=EDGE_CURVE('',#4144,#4142,#2864,.T.);
#5431=EDGE_CURVE('',#4144,#4145,#2036,.T.);
#5432=EDGE_CURVE('',#4145,#4143,#2865,.T.);
#5433=EDGE_CURVE('',#4143,#4121,#2037,.T.);
#5434=EDGE_CURVE('',#4146,#4143,#2866,.T.);
#5435=EDGE_CURVE('',#4146,#4108,#2038,.T.);
#5436=EDGE_CURVE('',#4145,#4147,#2867,.T.);
#5437=EDGE_CURVE('',#4147,#4148,#2405,.T.);
#5438=EDGE_CURVE('',#4148,#4149,#2868,.T.);
#5439=EDGE_CURVE('',#4149,#4146,#2406,.T.);
#5440=EDGE_CURVE('',#4150,#4146,#2407,.T.);
#5441=EDGE_CURVE('',#4151,#4149,#2039,.T.);
#5442=EDGE_CURVE('',#4151,#4152,#116,.T.);
#5443=EDGE_CURVE('',#4150,#4152,#2408,.T.);
#5444=EDGE_CURVE('',#4153,#4150,#2409,.T.);
#5445=EDGE_CURVE('',#4153,#4107,#117,.T.);
#5446=EDGE_CURVE('',#4153,#4154,#2869,.T.);
#5447=EDGE_CURVE('',#4154,#4109,#2040,.T.);
#5448=EDGE_CURVE('',#4155,#4154,#2410,.T.);
#5449=EDGE_CURVE('',#4155,#4110,#2041,.T.);
#5450=EDGE_CURVE('',#4154,#4156,#2870,.T.);
#5451=EDGE_CURVE('',#4157,#4156,#118,.T.);
#5452=EDGE_CURVE('',#4158,#4157,#2871,.T.);
#5453=EDGE_CURVE('',#4158,#4159,#2411,.T.);
#5454=EDGE_CURVE('',#4160,#4159,#2412,.T.);
#5455=EDGE_CURVE('',#4161,#4160,#2413,.T.);
#5456=EDGE_CURVE('',#4155,#4161,#2414,.T.);
#5457=EDGE_CURVE('',#4162,#4155,#2415,.T.);
#5458=EDGE_CURVE('',#4161,#4162,#2042,.T.);
#5459=EDGE_CURVE('',#4162,#4111,#2043,.T.);
#5460=EDGE_CURVE('',#4163,#4162,#2416,.T.);
#5461=EDGE_CURVE('',#4163,#4112,#2044,.T.);
#5462=EDGE_CURVE('',#4160,#4164,#2045,.T.);
#5463=EDGE_CURVE('',#4164,#4165,#2417,.T.);
#5464=EDGE_CURVE('',#4165,#4163,#2418,.T.);
#5465=EDGE_CURVE('',#4165,#4166,#2046,.T.);
#5466=EDGE_CURVE('',#4166,#4112,#2419,.T.);
#5467=EDGE_CURVE('',#4113,#4167,#2047,.T.);
#5468=EDGE_CURVE('',#4167,#4166,#2872,.T.);
#5469=EDGE_CURVE('',#4168,#4169,#2048,.T.);
#5470=EDGE_CURVE('',#4168,#4113,#2049,.T.);
#5471=EDGE_CURVE('',#4169,#4167,#2050,.T.);
#5472=EDGE_CURVE('',#4142,#4168,#2873,.T.);
#5473=EDGE_CURVE('',#4169,#4170,#2874,.T.);
#5474=EDGE_CURVE('',#4170,#4171,#2051,.T.);
#5475=EDGE_CURVE('',#4171,#4144,#2875,.T.);
#5476=EDGE_CURVE('',#4172,#4172,#2052,.T.);
#5477=EDGE_CURVE('',#4173,#4173,#2053,.T.);
#5478=EDGE_CURVE('',#4173,#4172,#2876,.T.);
#5479=EDGE_CURVE('',#4174,#4174,#2054,.T.);
#5480=EDGE_CURVE('',#4175,#4175,#2055,.T.);
#5481=EDGE_CURVE('',#4175,#4103,#2877,.T.);
#5482=EDGE_CURVE('',#4104,#4174,#2878,.T.);
#5483=EDGE_CURVE('',#4176,#4177,#119,.T.);
#5484=EDGE_CURVE('',#4176,#4178,#2879,.T.);
#5485=EDGE_CURVE('',#4178,#4179,#120,.T.);
#5486=EDGE_CURVE('',#4180,#4179,#2880,.T.);
#5487=EDGE_CURVE('',#4181,#4180,#121,.T.);
#5488=EDGE_CURVE('',#4157,#4181,#2881,.T.);
#5489=EDGE_CURVE('',#4156,#4177,#2882,.T.);
#5490=EDGE_CURVE('',#4176,#4151,#2883,.T.);
#5491=EDGE_CURVE('',#4177,#4152,#2884,.T.);
#5492=EDGE_CURVE('',#4182,#4151,#2885,.T.);
#5493=EDGE_CURVE('',#4182,#4178,#2886,.T.);
#5494=EDGE_CURVE('',#4182,#4148,#2056,.T.);
#5495=EDGE_CURVE('',#4147,#4183,#2420,.T.);
#5496=EDGE_CURVE('',#4184,#4183,#2421,.T.);
#5497=EDGE_CURVE('',#4184,#4182,#122,.T.);
#5498=EDGE_CURVE('',#4183,#4185,#2422,.T.);
#5499=EDGE_CURVE('',#4147,#4069,#2057,.T.);
#5500=EDGE_CURVE('',#4185,#4068,#123,.T.);
#5501=EDGE_CURVE('',#4185,#4186,#2887,.T.);
#5502=EDGE_CURVE('',#4180,#4186,#2888,.T.);
#5503=EDGE_CURVE('',#4184,#4179,#2889,.T.);
#5504=EDGE_CURVE('',#4186,#4187,#2423,.T.);
#5505=EDGE_CURVE('',#4181,#4187,#2890,.T.);
#5506=EDGE_CURVE('',#4186,#4067,#124,.T.);
#5507=EDGE_CURVE('',#4067,#4188,#2424,.T.);
#5508=EDGE_CURVE('',#4187,#4188,#125,.T.);
#5509=EDGE_CURVE('',#4187,#4158,#2891,.T.);
#5510=EDGE_CURVE('',#4188,#4189,#2892,.T.);
#5511=EDGE_CURVE('',#4158,#4189,#2058,.T.);
#5512=EDGE_CURVE('',#4189,#4190,#126,.T.);
#5513=EDGE_CURVE('',#4159,#4190,#2059,.T.);
#5514=EDGE_CURVE('',#4159,#4164,#2425,.T.);
#5515=EDGE_CURVE('',#4190,#4191,#2426,.T.);
#5516=EDGE_CURVE('',#4164,#4191,#2060,.T.);
#5517=EDGE_CURVE('',#4191,#4166,#2427,.T.);
#5518=EDGE_CURVE('',#4167,#4192,#2893,.T.);
#5519=EDGE_CURVE('',#4192,#4188,#2894,.T.);
#5520=EDGE_CURVE('',#4170,#4192,#2061,.T.);
#5521=EDGE_CURVE('',#4192,#4065,#2062,.T.);
#5522=EDGE_CURVE('',#4171,#4065,#2063,.T.);
#5523=EDGE_CURVE('',#4144,#4066,#2064,.T.);
#5524=EDGE_CURVE('',#4145,#4070,#2065,.T.);
#7732=ORIENTED_EDGE('',*,*,#5312,.F.);
#7733=ORIENTED_EDGE('',*,*,#5313,.T.);
#7734=ORIENTED_EDGE('',*,*,#5314,.F.);
#7735=ORIENTED_EDGE('',*,*,#5315,.F.);
#7736=ORIENTED_EDGE('',*,*,#5316,.F.);
#7737=ORIENTED_EDGE('',*,*,#5317,.F.);
#7738=ORIENTED_EDGE('',*,*,#5318,.F.);
#7739=ORIENTED_EDGE('',*,*,#5319,.F.);
#7740=ORIENTED_EDGE('',*,*,#5320,.F.);
#7741=ORIENTED_EDGE('',*,*,#5321,.T.);
#7742=ORIENTED_EDGE('',*,*,#5318,.T.);
#7743=ORIENTED_EDGE('',*,*,#5321,.F.);
#7744=ORIENTED_EDGE('',*,*,#5322,.F.);
#7745=ORIENTED_EDGE('',*,*,#5323,.T.);
#7746=ORIENTED_EDGE('',*,*,#5319,.T.);
#7747=ORIENTED_EDGE('',*,*,#5320,.T.);
#7748=ORIENTED_EDGE('',*,*,#5323,.F.);
#7749=ORIENTED_EDGE('',*,*,#5322,.T.);
#7750=ORIENTED_EDGE('',*,*,#5324,.T.);
#7751=ORIENTED_EDGE('',*,*,#5325,.F.);
#7752=ORIENTED_EDGE('',*,*,#5326,.F.);
#7753=ORIENTED_EDGE('',*,*,#5327,.T.);
#7754=ORIENTED_EDGE('',*,*,#5324,.F.);
#7755=ORIENTED_EDGE('',*,*,#5327,.F.);
#7756=ORIENTED_EDGE('',*,*,#5328,.F.);
#7757=ORIENTED_EDGE('',*,*,#5329,.T.);
#7758=ORIENTED_EDGE('',*,*,#5330,.F.);
#7759=ORIENTED_EDGE('',*,*,#5331,.F.);
#7760=ORIENTED_EDGE('',*,*,#5332,.F.);
#7761=ORIENTED_EDGE('',*,*,#5329,.F.);
#7762=ORIENTED_EDGE('',*,*,#5333,.F.);
#7763=ORIENTED_EDGE('',*,*,#5325,.T.);
#7764=ORIENTED_EDGE('',*,*,#5326,.T.);
#7765=ORIENTED_EDGE('',*,*,#5334,.F.);
#7766=ORIENTED_EDGE('',*,*,#5335,.F.);
#7767=ORIENTED_EDGE('',*,*,#5333,.T.);
#7768=ORIENTED_EDGE('',*,*,#5336,.T.);
#7769=ORIENTED_EDGE('',*,*,#5337,.F.);
#7770=ORIENTED_EDGE('',*,*,#5338,.F.);
#7771=ORIENTED_EDGE('',*,*,#5339,.F.);
#7772=ORIENTED_EDGE('',*,*,#5340,.F.);
#7773=ORIENTED_EDGE('',*,*,#5334,.T.);
#7774=ORIENTED_EDGE('',*,*,#5340,.T.);
#7775=ORIENTED_EDGE('',*,*,#5339,.T.);
#7776=ORIENTED_EDGE('',*,*,#5338,.T.);
#7777=ORIENTED_EDGE('',*,*,#5341,.T.);
#7778=ORIENTED_EDGE('',*,*,#5342,.F.);
#7779=ORIENTED_EDGE('',*,*,#5343,.F.);
#7780=ORIENTED_EDGE('',*,*,#5344,.F.);
#7781=ORIENTED_EDGE('',*,*,#5335,.T.);
#7782=ORIENTED_EDGE('',*,*,#5344,.T.);
#7783=ORIENTED_EDGE('',*,*,#5345,.F.);
#7784=ORIENTED_EDGE('',*,*,#5336,.F.);
#7785=ORIENTED_EDGE('',*,*,#5345,.T.);
#7786=ORIENTED_EDGE('',*,*,#5346,.T.);
#7787=ORIENTED_EDGE('',*,*,#5347,.F.);
#7788=ORIENTED_EDGE('',*,*,#5348,.F.);
#7789=ORIENTED_EDGE('',*,*,#5342,.T.);
#7790=ORIENTED_EDGE('',*,*,#5341,.F.);
#7791=ORIENTED_EDGE('',*,*,#5337,.T.);
#7792=ORIENTED_EDGE('',*,*,#5348,.T.);
#7793=ORIENTED_EDGE('',*,*,#5349,.F.);
#7794=ORIENTED_EDGE('',*,*,#5350,.F.);
#7795=ORIENTED_EDGE('',*,*,#5350,.T.);
#7796=ORIENTED_EDGE('',*,*,#5351,.T.);
#7797=ORIENTED_EDGE('',*,*,#5352,.F.);
#7798=ORIENTED_EDGE('',*,*,#5346,.F.);
#7799=ORIENTED_EDGE('',*,*,#5343,.T.);
#7800=ORIENTED_EDGE('',*,*,#5353,.T.);
#7801=ORIENTED_EDGE('',*,*,#5354,.T.);
#7802=ORIENTED_EDGE('',*,*,#5355,.F.);
#7803=ORIENTED_EDGE('',*,*,#5356,.F.);
#7804=ORIENTED_EDGE('',*,*,#5352,.T.);
#7805=ORIENTED_EDGE('',*,*,#5353,.F.);
#7806=ORIENTED_EDGE('',*,*,#5351,.F.);
#7807=ORIENTED_EDGE('',*,*,#5349,.T.);
#7808=ORIENTED_EDGE('',*,*,#5357,.T.);
#7809=ORIENTED_EDGE('',*,*,#5358,.F.);
#7810=ORIENTED_EDGE('',*,*,#5354,.F.);
#7811=ORIENTED_EDGE('',*,*,#5358,.T.);
#7812=ORIENTED_EDGE('',*,*,#5359,.T.);
#7813=ORIENTED_EDGE('',*,*,#5360,.F.);
#7814=ORIENTED_EDGE('',*,*,#5361,.F.);
#7815=ORIENTED_EDGE('',*,*,#5361,.T.);
#7816=ORIENTED_EDGE('',*,*,#5330,.T.);
#7817=ORIENTED_EDGE('',*,*,#5332,.T.);
#7818=ORIENTED_EDGE('',*,*,#5362,.F.);
#7819=ORIENTED_EDGE('',*,*,#5363,.F.);
#7820=ORIENTED_EDGE('',*,*,#5355,.T.);
#7821=ORIENTED_EDGE('',*,*,#5364,.T.);
#7822=ORIENTED_EDGE('',*,*,#5363,.T.);
#7823=ORIENTED_EDGE('',*,*,#5365,.F.);
#7824=ORIENTED_EDGE('',*,*,#5359,.F.);
#7825=ORIENTED_EDGE('',*,*,#5347,.T.);
#7826=ORIENTED_EDGE('',*,*,#5356,.T.);
#7827=ORIENTED_EDGE('',*,*,#5364,.F.);
#7828=ORIENTED_EDGE('',*,*,#5357,.F.);
#7829=ORIENTED_EDGE('',*,*,#5360,.T.);
#7830=ORIENTED_EDGE('',*,*,#5365,.T.);
#7831=ORIENTED_EDGE('',*,*,#5362,.T.);
#7832=ORIENTED_EDGE('',*,*,#5331,.T.);
#7833=ORIENTED_EDGE('',*,*,#5366,.T.);
#7834=ORIENTED_EDGE('',*,*,#5328,.T.);
#7835=ORIENTED_EDGE('',*,*,#5366,.F.);
#7836=ORIENTED_EDGE('',*,*,#5367,.T.);
#7837=ORIENTED_EDGE('',*,*,#5368,.T.);
#7838=ORIENTED_EDGE('',*,*,#5367,.F.);
#7839=ORIENTED_EDGE('',*,*,#5369,.T.);
#7840=ORIENTED_EDGE('',*,*,#5370,.T.);
#7841=ORIENTED_EDGE('',*,*,#5371,.T.);
#7842=ORIENTED_EDGE('',*,*,#5368,.F.);
#7843=ORIENTED_EDGE('',*,*,#5371,.F.);
#7844=ORIENTED_EDGE('',*,*,#5372,.T.);
#7845=ORIENTED_EDGE('',*,*,#5373,.T.);
#7846=ORIENTED_EDGE('',*,*,#5372,.F.);
#7847=ORIENTED_EDGE('',*,*,#5374,.F.);
#7848=ORIENTED_EDGE('',*,*,#5375,.F.);
#7849=ORIENTED_EDGE('',*,*,#5376,.F.);
#7850=ORIENTED_EDGE('',*,*,#5377,.F.);
#7851=ORIENTED_EDGE('',*,*,#5378,.F.);
#7852=ORIENTED_EDGE('',*,*,#5379,.F.);
#7853=ORIENTED_EDGE('',*,*,#5380,.F.);
#7854=ORIENTED_EDGE('',*,*,#5381,.F.);
#7855=ORIENTED_EDGE('',*,*,#5382,.F.);
#7856=ORIENTED_EDGE('',*,*,#5383,.F.);
#7857=ORIENTED_EDGE('',*,*,#5384,.F.);
#7858=ORIENTED_EDGE('',*,*,#5385,.F.);
#7859=ORIENTED_EDGE('',*,*,#5386,.F.);
#7860=ORIENTED_EDGE('',*,*,#5387,.F.);
#7861=ORIENTED_EDGE('',*,*,#5388,.F.);
#7862=ORIENTED_EDGE('',*,*,#5389,.T.);
#7863=ORIENTED_EDGE('',*,*,#5373,.F.);
#7864=ORIENTED_EDGE('',*,*,#5390,.T.);
#7865=ORIENTED_EDGE('',*,*,#5391,.T.);
#7866=ORIENTED_EDGE('',*,*,#5389,.F.);
#7867=ORIENTED_EDGE('',*,*,#5391,.F.);
#7868=ORIENTED_EDGE('',*,*,#5392,.T.);
#7869=ORIENTED_EDGE('',*,*,#5393,.T.);
#7870=ORIENTED_EDGE('',*,*,#5394,.T.);
#7871=ORIENTED_EDGE('',*,*,#5395,.T.);
#7872=ORIENTED_EDGE('',*,*,#5390,.F.);
#7873=ORIENTED_EDGE('',*,*,#5392,.F.);
#7874=ORIENTED_EDGE('',*,*,#5396,.T.);
#7875=ORIENTED_EDGE('',*,*,#5397,.F.);
#7876=ORIENTED_EDGE('',*,*,#5398,.F.);
#7877=ORIENTED_EDGE('',*,*,#5399,.F.);
#7878=ORIENTED_EDGE('',*,*,#5398,.T.);
#7879=ORIENTED_EDGE('',*,*,#5400,.T.);
#7880=ORIENTED_EDGE('',*,*,#5401,.F.);
#7881=ORIENTED_EDGE('',*,*,#5402,.F.);
#7882=ORIENTED_EDGE('',*,*,#5393,.F.);
#7883=ORIENTED_EDGE('',*,*,#5399,.T.);
#7884=ORIENTED_EDGE('',*,*,#5403,.T.);
#7885=ORIENTED_EDGE('',*,*,#5404,.F.);
#7886=ORIENTED_EDGE('',*,*,#5405,.T.);
#7887=ORIENTED_EDGE('',*,*,#5402,.T.);
#7888=ORIENTED_EDGE('',*,*,#5406,.F.);
#7889=ORIENTED_EDGE('',*,*,#5407,.T.);
#7890=ORIENTED_EDGE('',*,*,#5408,.T.);
#7891=ORIENTED_EDGE('',*,*,#5404,.T.);
#7892=ORIENTED_EDGE('',*,*,#5409,.T.);
#7893=ORIENTED_EDGE('',*,*,#5407,.F.);
#7894=ORIENTED_EDGE('',*,*,#5410,.T.);
#7895=ORIENTED_EDGE('',*,*,#5386,.T.);
#7896=ORIENTED_EDGE('',*,*,#5411,.F.);
#7897=ORIENTED_EDGE('',*,*,#5412,.F.);
#7898=ORIENTED_EDGE('',*,*,#5411,.T.);
#7899=ORIENTED_EDGE('',*,*,#5385,.T.);
#7900=ORIENTED_EDGE('',*,*,#5413,.F.);
#7901=ORIENTED_EDGE('',*,*,#5412,.T.);
#7902=ORIENTED_EDGE('',*,*,#5414,.T.);
#7903=ORIENTED_EDGE('',*,*,#5415,.T.);
#7904=ORIENTED_EDGE('',*,*,#5408,.F.);
#7905=ORIENTED_EDGE('',*,*,#5415,.F.);
#7906=ORIENTED_EDGE('',*,*,#5416,.F.);
#7907=ORIENTED_EDGE('',*,*,#5394,.F.);
#7908=ORIENTED_EDGE('',*,*,#5405,.F.);
#7909=ORIENTED_EDGE('',*,*,#5395,.F.);
#7910=ORIENTED_EDGE('',*,*,#5416,.T.);
#7911=ORIENTED_EDGE('',*,*,#5417,.T.);
#7912=ORIENTED_EDGE('',*,*,#5396,.F.);
#7913=ORIENTED_EDGE('',*,*,#5418,.T.);
#7914=ORIENTED_EDGE('',*,*,#5419,.T.);
#7915=ORIENTED_EDGE('',*,*,#5417,.F.);
#7916=ORIENTED_EDGE('',*,*,#5414,.F.);
#7917=ORIENTED_EDGE('',*,*,#5418,.F.);
#7918=ORIENTED_EDGE('',*,*,#5413,.T.);
#7919=ORIENTED_EDGE('',*,*,#5384,.T.);
#7920=ORIENTED_EDGE('',*,*,#5420,.F.);
#7921=ORIENTED_EDGE('',*,*,#5421,.F.);
#7922=ORIENTED_EDGE('',*,*,#5420,.T.);
#7923=ORIENTED_EDGE('',*,*,#5383,.T.);
#7924=ORIENTED_EDGE('',*,*,#5422,.F.);
#7925=ORIENTED_EDGE('',*,*,#5421,.T.);
#7926=ORIENTED_EDGE('',*,*,#5423,.F.);
#7927=ORIENTED_EDGE('',*,*,#5397,.T.);
#7928=ORIENTED_EDGE('',*,*,#5419,.F.);
#7929=ORIENTED_EDGE('',*,*,#5424,.T.);
#7930=ORIENTED_EDGE('',*,*,#5425,.T.);
#7931=ORIENTED_EDGE('',*,*,#5400,.F.);
#7932=ORIENTED_EDGE('',*,*,#5423,.T.);
#7933=ORIENTED_EDGE('',*,*,#5424,.F.);
#7934=ORIENTED_EDGE('',*,*,#5422,.T.);
#7935=ORIENTED_EDGE('',*,*,#5382,.T.);
#7936=ORIENTED_EDGE('',*,*,#5426,.F.);
#7937=ORIENTED_EDGE('',*,*,#5427,.F.);
#7938=ORIENTED_EDGE('',*,*,#5426,.T.);
#7939=ORIENTED_EDGE('',*,*,#5381,.T.);
#7940=ORIENTED_EDGE('',*,*,#5428,.F.);
#7941=ORIENTED_EDGE('',*,*,#5429,.T.);
#7942=ORIENTED_EDGE('',*,*,#5409,.F.);
#7943=ORIENTED_EDGE('',*,*,#5406,.T.);
#7944=ORIENTED_EDGE('',*,*,#5403,.F.);
#7945=ORIENTED_EDGE('',*,*,#5401,.T.);
#7946=ORIENTED_EDGE('',*,*,#5425,.F.);
#7947=ORIENTED_EDGE('',*,*,#5427,.T.);
#7948=ORIENTED_EDGE('',*,*,#5430,.F.);
#7949=ORIENTED_EDGE('',*,*,#5431,.T.);
#7950=ORIENTED_EDGE('',*,*,#5432,.T.);
#7951=ORIENTED_EDGE('',*,*,#5429,.F.);
#7952=ORIENTED_EDGE('',*,*,#5433,.T.);
#7953=ORIENTED_EDGE('',*,*,#5387,.T.);
#7954=ORIENTED_EDGE('',*,*,#5410,.F.);
#7955=ORIENTED_EDGE('',*,*,#5434,.F.);
#7956=ORIENTED_EDGE('',*,*,#5435,.T.);
#7957=ORIENTED_EDGE('',*,*,#5388,.T.);
#7958=ORIENTED_EDGE('',*,*,#5433,.F.);
#7959=ORIENTED_EDGE('',*,*,#5434,.T.);
#7960=ORIENTED_EDGE('',*,*,#5432,.F.);
#7961=ORIENTED_EDGE('',*,*,#5436,.T.);
#7962=ORIENTED_EDGE('',*,*,#5437,.T.);
#7963=ORIENTED_EDGE('',*,*,#5438,.T.);
#7964=ORIENTED_EDGE('',*,*,#5439,.T.);
#7965=ORIENTED_EDGE('',*,*,#5440,.T.);
#7966=ORIENTED_EDGE('',*,*,#5439,.F.);
#7967=ORIENTED_EDGE('',*,*,#5441,.F.);
#7968=ORIENTED_EDGE('',*,*,#5442,.T.);
#7969=ORIENTED_EDGE('',*,*,#5443,.F.);
#7970=ORIENTED_EDGE('',*,*,#5440,.F.);
#7971=ORIENTED_EDGE('',*,*,#5444,.F.);
#7972=ORIENTED_EDGE('',*,*,#5445,.T.);
#7973=ORIENTED_EDGE('',*,*,#5374,.T.);
#7974=ORIENTED_EDGE('',*,*,#5435,.F.);
#7975=ORIENTED_EDGE('',*,*,#5375,.T.);
#7976=ORIENTED_EDGE('',*,*,#5445,.F.);
#7977=ORIENTED_EDGE('',*,*,#5446,.T.);
#7978=ORIENTED_EDGE('',*,*,#5447,.T.);
#7979=ORIENTED_EDGE('',*,*,#5448,.F.);
#7980=ORIENTED_EDGE('',*,*,#5449,.T.);
#7981=ORIENTED_EDGE('',*,*,#5376,.T.);
#7982=ORIENTED_EDGE('',*,*,#5447,.F.);
#7983=ORIENTED_EDGE('',*,*,#5448,.T.);
#7984=ORIENTED_EDGE('',*,*,#5450,.T.);
#7985=ORIENTED_EDGE('',*,*,#5451,.F.);
#7986=ORIENTED_EDGE('',*,*,#5452,.F.);
#7987=ORIENTED_EDGE('',*,*,#5453,.T.);
#7988=ORIENTED_EDGE('',*,*,#5454,.F.);
#7989=ORIENTED_EDGE('',*,*,#5455,.F.);
#7990=ORIENTED_EDGE('',*,*,#5456,.F.);
#7991=ORIENTED_EDGE('',*,*,#5457,.T.);
#7992=ORIENTED_EDGE('',*,*,#5456,.T.);
#7993=ORIENTED_EDGE('',*,*,#5458,.T.);
#7994=ORIENTED_EDGE('',*,*,#5457,.F.);
#7995=ORIENTED_EDGE('',*,*,#5459,.T.);
#7996=ORIENTED_EDGE('',*,*,#5377,.T.);
#7997=ORIENTED_EDGE('',*,*,#5449,.F.);
#7998=ORIENTED_EDGE('',*,*,#5460,.F.);
#7999=ORIENTED_EDGE('',*,*,#5461,.T.);
#8000=ORIENTED_EDGE('',*,*,#5378,.T.);
#8001=ORIENTED_EDGE('',*,*,#5459,.F.);
#8002=ORIENTED_EDGE('',*,*,#5460,.T.);
#8003=ORIENTED_EDGE('',*,*,#5458,.F.);
#8004=ORIENTED_EDGE('',*,*,#5455,.T.);
#8005=ORIENTED_EDGE('',*,*,#5462,.T.);
#8006=ORIENTED_EDGE('',*,*,#5463,.T.);
#8007=ORIENTED_EDGE('',*,*,#5464,.T.);
#8008=ORIENTED_EDGE('',*,*,#5464,.F.);
#8009=ORIENTED_EDGE('',*,*,#5465,.T.);
#8010=ORIENTED_EDGE('',*,*,#5466,.T.);
#8011=ORIENTED_EDGE('',*,*,#5461,.F.);
#8012=ORIENTED_EDGE('',*,*,#5467,.F.);
#8013=ORIENTED_EDGE('',*,*,#5379,.T.);
#8014=ORIENTED_EDGE('',*,*,#5466,.F.);
#8015=ORIENTED_EDGE('',*,*,#5468,.F.);
#8016=ORIENTED_EDGE('',*,*,#5469,.F.);
#8017=ORIENTED_EDGE('',*,*,#5470,.T.);
#8018=ORIENTED_EDGE('',*,*,#5467,.T.);
#8019=ORIENTED_EDGE('',*,*,#5471,.F.);
#8020=ORIENTED_EDGE('',*,*,#5472,.T.);
#8021=ORIENTED_EDGE('',*,*,#5469,.T.);
#8022=ORIENTED_EDGE('',*,*,#5473,.T.);
#8023=ORIENTED_EDGE('',*,*,#5474,.T.);
#8024=ORIENTED_EDGE('',*,*,#5475,.T.);
#8025=ORIENTED_EDGE('',*,*,#5430,.T.);
#8026=ORIENTED_EDGE('',*,*,#5476,.F.);
#8027=ORIENTED_EDGE('',*,*,#5477,.F.);
#8028=ORIENTED_EDGE('',*,*,#5478,.T.);
#8029=ORIENTED_EDGE('',*,*,#5476,.T.);
#8030=ORIENTED_EDGE('',*,*,#5478,.F.);
#8031=ORIENTED_EDGE('',*,*,#5477,.T.);
#8032=ORIENTED_EDGE('',*,*,#5479,.F.);
#8033=ORIENTED_EDGE('',*,*,#5480,.F.);
#8034=ORIENTED_EDGE('',*,*,#5481,.T.);
#8035=ORIENTED_EDGE('',*,*,#5370,.F.);
#8036=ORIENTED_EDGE('',*,*,#5482,.T.);
#8037=ORIENTED_EDGE('',*,*,#5479,.T.);
#8038=ORIENTED_EDGE('',*,*,#5482,.F.);
#8039=ORIENTED_EDGE('',*,*,#5369,.F.);
#8040=ORIENTED_EDGE('',*,*,#5481,.F.);
#8041=ORIENTED_EDGE('',*,*,#5483,.F.);
#8042=ORIENTED_EDGE('',*,*,#5484,.T.);
#8043=ORIENTED_EDGE('',*,*,#5485,.T.);
#8044=ORIENTED_EDGE('',*,*,#5486,.F.);
#8045=ORIENTED_EDGE('',*,*,#5487,.F.);
#8046=ORIENTED_EDGE('',*,*,#5488,.F.);
#8047=ORIENTED_EDGE('',*,*,#5451,.T.);
#8048=ORIENTED_EDGE('',*,*,#5489,.T.);
#8049=ORIENTED_EDGE('',*,*,#5480,.T.);
#8050=ORIENTED_EDGE('',*,*,#5442,.F.);
#8051=ORIENTED_EDGE('',*,*,#5490,.F.);
#8052=ORIENTED_EDGE('',*,*,#5483,.T.);
#8053=ORIENTED_EDGE('',*,*,#5491,.T.);
#8054=ORIENTED_EDGE('',*,*,#5443,.T.);
#8055=ORIENTED_EDGE('',*,*,#5491,.F.);
#8056=ORIENTED_EDGE('',*,*,#5489,.F.);
#8057=ORIENTED_EDGE('',*,*,#5450,.F.);
#8058=ORIENTED_EDGE('',*,*,#5446,.F.);
#8059=ORIENTED_EDGE('',*,*,#5444,.T.);
#8060=ORIENTED_EDGE('',*,*,#5492,.F.);
#8061=ORIENTED_EDGE('',*,*,#5493,.T.);
#8062=ORIENTED_EDGE('',*,*,#5484,.F.);
#8063=ORIENTED_EDGE('',*,*,#5490,.T.);
#8064=ORIENTED_EDGE('',*,*,#5492,.T.);
#8065=ORIENTED_EDGE('',*,*,#5441,.T.);
#8066=ORIENTED_EDGE('',*,*,#5438,.F.);
#8067=ORIENTED_EDGE('',*,*,#5494,.F.);
#8068=ORIENTED_EDGE('',*,*,#5495,.T.);
#8069=ORIENTED_EDGE('',*,*,#5496,.F.);
#8070=ORIENTED_EDGE('',*,*,#5497,.T.);
#8071=ORIENTED_EDGE('',*,*,#5494,.T.);
#8072=ORIENTED_EDGE('',*,*,#5437,.F.);
#8073=ORIENTED_EDGE('',*,*,#5498,.F.);
#8074=ORIENTED_EDGE('',*,*,#5495,.F.);
#8075=ORIENTED_EDGE('',*,*,#5499,.T.);
#8076=ORIENTED_EDGE('',*,*,#5315,.T.);
#8077=ORIENTED_EDGE('',*,*,#5500,.F.);
#8078=ORIENTED_EDGE('',*,*,#5498,.T.);
#8079=ORIENTED_EDGE('',*,*,#5501,.T.);
#8080=ORIENTED_EDGE('',*,*,#5502,.F.);
#8081=ORIENTED_EDGE('',*,*,#5486,.T.);
#8082=ORIENTED_EDGE('',*,*,#5503,.F.);
#8083=ORIENTED_EDGE('',*,*,#5496,.T.);
#8084=ORIENTED_EDGE('',*,*,#5497,.F.);
#8085=ORIENTED_EDGE('',*,*,#5503,.T.);
#8086=ORIENTED_EDGE('',*,*,#5485,.F.);
#8087=ORIENTED_EDGE('',*,*,#5493,.F.);
#8088=ORIENTED_EDGE('',*,*,#5504,.T.);
#8089=ORIENTED_EDGE('',*,*,#5505,.F.);
#8090=ORIENTED_EDGE('',*,*,#5487,.T.);
#8091=ORIENTED_EDGE('',*,*,#5502,.T.);
#8092=ORIENTED_EDGE('',*,*,#5504,.F.);
#8093=ORIENTED_EDGE('',*,*,#5506,.T.);
#8094=ORIENTED_EDGE('',*,*,#5507,.T.);
#8095=ORIENTED_EDGE('',*,*,#5508,.F.);
#8096=ORIENTED_EDGE('',*,*,#5509,.F.);
#8097=ORIENTED_EDGE('',*,*,#5508,.T.);
#8098=ORIENTED_EDGE('',*,*,#5510,.T.);
#8099=ORIENTED_EDGE('',*,*,#5511,.F.);
#8100=ORIENTED_EDGE('',*,*,#5509,.T.);
#8101=ORIENTED_EDGE('',*,*,#5452,.T.);
#8102=ORIENTED_EDGE('',*,*,#5488,.T.);
#8103=ORIENTED_EDGE('',*,*,#5505,.T.);
#8104=ORIENTED_EDGE('',*,*,#5453,.F.);
#8105=ORIENTED_EDGE('',*,*,#5511,.T.);
#8106=ORIENTED_EDGE('',*,*,#5512,.T.);
#8107=ORIENTED_EDGE('',*,*,#5513,.F.);
#8108=ORIENTED_EDGE('',*,*,#5514,.F.);
#8109=ORIENTED_EDGE('',*,*,#5513,.T.);
#8110=ORIENTED_EDGE('',*,*,#5515,.T.);
#8111=ORIENTED_EDGE('',*,*,#5516,.F.);
#8112=ORIENTED_EDGE('',*,*,#5514,.T.);
#8113=ORIENTED_EDGE('',*,*,#5462,.F.);
#8114=ORIENTED_EDGE('',*,*,#5454,.T.);
#8115=ORIENTED_EDGE('',*,*,#5463,.F.);
#8116=ORIENTED_EDGE('',*,*,#5516,.T.);
#8117=ORIENTED_EDGE('',*,*,#5517,.T.);
#8118=ORIENTED_EDGE('',*,*,#5465,.F.);
#8119=ORIENTED_EDGE('',*,*,#5518,.F.);
#8120=ORIENTED_EDGE('',*,*,#5468,.T.);
#8121=ORIENTED_EDGE('',*,*,#5517,.F.);
#8122=ORIENTED_EDGE('',*,*,#5515,.F.);
#8123=ORIENTED_EDGE('',*,*,#5512,.F.);
#8124=ORIENTED_EDGE('',*,*,#5510,.F.);
#8125=ORIENTED_EDGE('',*,*,#5519,.F.);
#8126=ORIENTED_EDGE('',*,*,#5473,.F.);
#8127=ORIENTED_EDGE('',*,*,#5471,.T.);
#8128=ORIENTED_EDGE('',*,*,#5518,.T.);
#8129=ORIENTED_EDGE('',*,*,#5520,.F.);
#8130=ORIENTED_EDGE('',*,*,#5474,.F.);
#8131=ORIENTED_EDGE('',*,*,#5520,.T.);
#8132=ORIENTED_EDGE('',*,*,#5521,.T.);
#8133=ORIENTED_EDGE('',*,*,#5522,.F.);
#8134=ORIENTED_EDGE('',*,*,#5475,.F.);
#8135=ORIENTED_EDGE('',*,*,#5522,.T.);
#8136=ORIENTED_EDGE('',*,*,#5312,.T.);
#8137=ORIENTED_EDGE('',*,*,#5523,.F.);
#8138=ORIENTED_EDGE('',*,*,#5431,.F.);
#8139=ORIENTED_EDGE('',*,*,#5523,.T.);
#8140=ORIENTED_EDGE('',*,*,#5317,.T.);
#8141=ORIENTED_EDGE('',*,*,#5524,.F.);
#8142=ORIENTED_EDGE('',*,*,#5436,.F.);
#8143=ORIENTED_EDGE('',*,*,#5524,.T.);
#8144=ORIENTED_EDGE('',*,*,#5316,.T.);
#8145=ORIENTED_EDGE('',*,*,#5499,.F.);
#8146=ORIENTED_EDGE('',*,*,#5521,.F.);
#8147=ORIENTED_EDGE('',*,*,#5519,.T.);
#8148=ORIENTED_EDGE('',*,*,#5507,.F.);
#8149=ORIENTED_EDGE('',*,*,#5313,.F.);
#8150=ORIENTED_EDGE('',*,*,#5501,.F.);
#8151=ORIENTED_EDGE('',*,*,#5500,.T.);
#8152=ORIENTED_EDGE('',*,*,#5314,.T.);
#8153=ORIENTED_EDGE('',*,*,#5506,.F.);
#8154=ORIENTED_EDGE('',*,*,#5472,.F.);
#8155=ORIENTED_EDGE('',*,*,#5428,.T.);
#8156=ORIENTED_EDGE('',*,*,#5380,.T.);
#8157=ORIENTED_EDGE('',*,*,#5470,.F.);
#8537=CYLINDRICAL_SURFACE('',#9995,5.);
#8538=CYLINDRICAL_SURFACE('',#9999,4.);
#8539=CYLINDRICAL_SURFACE('',#10002,4.);
#8540=CYLINDRICAL_SURFACE('',#10008,6.);
#8541=CYLINDRICAL_SURFACE('',#10012,6.75);
#8542=CYLINDRICAL_SURFACE('',#10021,1.25);
#8543=CYLINDRICAL_SURFACE('',#10026,0.5);
#8544=CYLINDRICAL_SURFACE('',#10034,1.);
#8545=CYLINDRICAL_SURFACE('',#10039,0.5);
#8546=CYLINDRICAL_SURFACE('',#10042,0.5);
#8547=CYLINDRICAL_SURFACE('',#10046,3.);
#8548=CYLINDRICAL_SURFACE('',#10050,0.5);
#8549=CYLINDRICAL_SURFACE('',#10053,1.);
#8550=CYLINDRICAL_SURFACE('',#10060,8.);
#8551=CYLINDRICAL_SURFACE('',#10065,0.5);
#8552=CYLINDRICAL_SURFACE('',#10071,0.5);
#8553=CYLINDRICAL_SURFACE('',#10074,3.);
#8554=CYLINDRICAL_SURFACE('',#10081,1.);
#8555=CYLINDRICAL_SURFACE('',#10089,3.6);
#8556=CYLINDRICAL_SURFACE('',#10093,3.23);
#8557=CYLINDRICAL_SURFACE('',#10099,3.);
#8558=CYLINDRICAL_SURFACE('',#10102,1.);
#8559=CYLINDRICAL_SURFACE('',#10108,3.);
#8560=CYLINDRICAL_SURFACE('',#10109,3.);
#8561=CYLINDRICAL_SURFACE('',#10112,0.5);
#8562=CYLINDRICAL_SURFACE('',#10119,0.5);
#8563=CYLINDRICAL_SURFACE('',#10124,0.5);
#8564=CYLINDRICAL_SURFACE('',#10128,0.5);
#8565=CYLINDRICAL_SURFACE('',#10129,3.);
#8566=CYLINDRICAL_SURFACE('',#10130,0.5);
#8567=CYLINDRICAL_SURFACE('',#10131,0.5);
#8986=ADVANCED_FACE('',(#923,#304),#484,.F.);
#8987=ADVANCED_FACE('',(#924),#220,.F.);
#8988=ADVANCED_FACE('',(#925),#8537,.T.);
#8989=ADVANCED_FACE('',(#926,#305),#485,.T.);
#8990=ADVANCED_FACE('',(#927),#8538,.F.);
#8991=ADVANCED_FACE('',(#928),#8539,.F.);
#8992=ADVANCED_FACE('',(#929),#486,.T.);
#8993=ADVANCED_FACE('',(#930),#388,.T.);
#8994=ADVANCED_FACE('',(#931),#389,.T.);
#8995=ADVANCED_FACE('',(#932),#390,.T.);
#8996=ADVANCED_FACE('',(#933),#391,.T.);
#8997=ADVANCED_FACE('',(#934),#392,.T.);
#8998=ADVANCED_FACE('',(#935),#393,.T.);
#8999=ADVANCED_FACE('',(#936),#394,.T.);
#9000=ADVANCED_FACE('',(#937),#395,.T.);
#9001=ADVANCED_FACE('',(#938),#396,.T.);
#9002=ADVANCED_FACE('',(#939),#397,.T.);
#9003=ADVANCED_FACE('',(#940),#398,.T.);
#9004=ADVANCED_FACE('',(#941),#399,.T.);
#9005=ADVANCED_FACE('',(#942),#487,.T.);
#9006=ADVANCED_FACE('',(#943,#306),#488,.T.);
#9007=ADVANCED_FACE('',(#944,#307),#8540,.F.);
#9008=ADVANCED_FACE('',(#945,#308),#489,.T.);
#9009=ADVANCED_FACE('',(#946),#8541,.F.);
#9010=ADVANCED_FACE('',(#947,#309,#310),#490,.T.);
#9011=ADVANCED_FACE('',(#948),#8542,.F.);
#9012=ADVANCED_FACE('',(#949,#311),#491,.F.);
#9013=ADVANCED_FACE('',(#950),#8543,.T.);
#9014=ADVANCED_FACE('',(#951),#180,.F.);
#9015=ADVANCED_FACE('',(#952),#221,.F.);
#9016=ADVANCED_FACE('',(#953),#181,.F.);
#9017=ADVANCED_FACE('',(#954),#8544,.F.);
#9018=ADVANCED_FACE('',(#955),#222,.T.);
#9019=ADVANCED_FACE('',(#956),#8545,.T.);
#9020=ADVANCED_FACE('',(#957),#492,.T.);
#9021=ADVANCED_FACE('',(#958),#8546,.T.);
#9022=ADVANCED_FACE('',(#959),#223,.T.);
#9023=ADVANCED_FACE('',(#960),#8547,.T.);
#9024=ADVANCED_FACE('',(#961),#224,.T.);
#9025=ADVANCED_FACE('',(#962),#8548,.T.);
#9026=ADVANCED_FACE('',(#963),#493,.T.);
#9027=ADVANCED_FACE('',(#964),#8549,.F.);
#9028=ADVANCED_FACE('',(#965),#225,.T.);
#9029=ADVANCED_FACE('',(#966),#226,.T.);
#9030=ADVANCED_FACE('',(#967),#8550,.T.);
#9031=ADVANCED_FACE('',(#968),#227,.T.);
#9032=ADVANCED_FACE('',(#969),#8551,.T.);
#9033=ADVANCED_FACE('',(#970),#494,.T.);
#9034=ADVANCED_FACE('',(#971),#182,.F.);
#9035=ADVANCED_FACE('',(#972),#183,.T.);
#9036=ADVANCED_FACE('',(#973),#8552,.T.);
#9037=ADVANCED_FACE('',(#974),#184,.T.);
#9038=ADVANCED_FACE('',(#975),#8553,.T.);
#9039=ADVANCED_FACE('',(#976),#185,.F.);
#9040=ADVANCED_FACE('',(#977),#186,.T.);
#9041=ADVANCED_FACE('',(#978),#187,.T.);
#9042=ADVANCED_FACE('',(#979),#188,.F.);
#9043=ADVANCED_FACE('',(#980),#189,.T.);
#9044=ADVANCED_FACE('',(#981),#8554,.T.);
#9045=ADVANCED_FACE('',(#982),#190,.F.);
#9046=ADVANCED_FACE('',(#983,#312),#495,.T.);
#9047=ADVANCED_FACE('',(#984),#8555,.F.);
#9048=ADVANCED_FACE('',(#985,#313),#496,.T.);
#9049=ADVANCED_FACE('',(#986),#8556,.F.);
#9050=ADVANCED_FACE('',(#987,#314),#497,.T.);
#9051=ADVANCED_FACE('',(#988),#8557,.T.);
#9052=ADVANCED_FACE('',(#989),#498,.F.);
#9053=ADVANCED_FACE('',(#990),#499,.F.);
#9054=ADVANCED_FACE('',(#991),#8558,.F.);
#9055=ADVANCED_FACE('',(#992),#191,.F.);
#9056=ADVANCED_FACE('',(#993),#192,.T.);
#9057=ADVANCED_FACE('',(#994),#500,.F.);
#9058=ADVANCED_FACE('',(#995),#8559,.T.);
#9059=ADVANCED_FACE('',(#996),#8560,.T.);
#9060=ADVANCED_FACE('',(#997),#193,.T.);
#9061=ADVANCED_FACE('',(#998),#8561,.T.);
#9062=ADVANCED_FACE('',(#999),#501,.F.);
#9063=ADVANCED_FACE('',(#1000),#194,.T.);
#9064=ADVANCED_FACE('',(#1001),#195,.T.);
#9065=ADVANCED_FACE('',(#1002),#196,.F.);
#9066=ADVANCED_FACE('',(#1003),#197,.T.);
#9067=ADVANCED_FACE('',(#1004),#502,.T.);
#9068=ADVANCED_FACE('',(#1005),#8562,.T.);
#9069=ADVANCED_FACE('',(#1006),#228,.T.);
#9070=ADVANCED_FACE('',(#1007),#8563,.T.);
#9071=ADVANCED_FACE('',(#1008),#229,.T.);
#9072=ADVANCED_FACE('',(#1009),#8564,.T.);
#9073=ADVANCED_FACE('',(#1010),#8565,.T.);
#9074=ADVANCED_FACE('',(#1011),#8566,.T.);
#9075=ADVANCED_FACE('',(#1012),#8567,.T.);
#9125=CLOSED_SHELL('',(#8986,#8987,#8988,#8989,#8990,#8991,#8992,#8993,
#8994,#8995,#8996,#8997,#8998,#8999,#9000,#9001,#9002,#9003,#9004,#9005,
#9006,#9007,#9008,#9009,#9010,#9011,#9012,#9013,#9014,#9015,#9016,#9017,
#9018,#9019,#9020,#9021,#9022,#9023,#9024,#9025,#9026,#9027,#9028,#9029,
#9030,#9031,#9032,#9033,#9034,#9035,#9036,#9037,#9038,#9039,#9040,#9041,
#9042,#9043,#9044,#9045,#9046,#9047,#9048,#9049,#9050,#9051,#9052,#9053,
#9054,#9055,#9056,#9057,#9058,#9059,#9060,#9061,#9062,#9063,#9064,#9065,
#9066,#9067,#9068,#9069,#9070,#9071,#9072,#9073,#9074,#9075));
#9987=AXIS2_PLACEMENT_3D('',#39898,#11998,#11999);
#9988=AXIS2_PLACEMENT_3D('',#39899,#12000,#12001);
#9989=AXIS2_PLACEMENT_3D('',#39921,#12006,#12007);
#9990=AXIS2_PLACEMENT_3D('',#39923,#12008,#12009);
#9991=AXIS2_PLACEMENT_3D('',#39924,#12010,#12011);
#9992=AXIS2_PLACEMENT_3D('',#39927,#12012,#12013);
#9993=AXIS2_PLACEMENT_3D('',#39928,#12014,#12015);
#9994=AXIS2_PLACEMENT_3D('',#39929,#12016,#12017);
#9995=AXIS2_PLACEMENT_3D('',#39930,#12018,#12019);
#9996=AXIS2_PLACEMENT_3D('',#39932,#12020,#12021);
#9997=AXIS2_PLACEMENT_3D('',#39934,#12023,#12024);
#9998=AXIS2_PLACEMENT_3D('',#39936,#12025,#12026);
#9999=AXIS2_PLACEMENT_3D('',#39937,#12027,#12028);
#10000=AXIS2_PLACEMENT_3D('',#39940,#12029,#12030);
#10001=AXIS2_PLACEMENT_3D('',#39941,#12031,#12032);
#10002=AXIS2_PLACEMENT_3D('',#39943,#12034,#12035);
#10003=AXIS2_PLACEMENT_3D('',#39945,#12036,#12037);
#10004=AXIS2_PLACEMENT_3D('',#40065,#12040,#12041);
#10005=AXIS2_PLACEMENT_3D('',#43371,#12051,#12052);
#10006=AXIS2_PLACEMENT_3D('',#43372,#12053,#12054);
#10007=AXIS2_PLACEMENT_3D('',#43374,#12055,#12056);
#10008=AXIS2_PLACEMENT_3D('',#43375,#12057,#12058);
#10009=AXIS2_PLACEMENT_3D('',#43378,#12060,#12061);
#10010=AXIS2_PLACEMENT_3D('',#43426,#12062,#12063);
#10011=AXIS2_PLACEMENT_3D('',#43428,#12064,#12065);
#10012=AXIS2_PLACEMENT_3D('',#43429,#12066,#12067);
#10013=AXIS2_PLACEMENT_3D('',#43432,#12069,#12070);
#10014=AXIS2_PLACEMENT_3D('',#43433,#12071,#12072);
#10015=AXIS2_PLACEMENT_3D('',#43636,#12076,#12077);
#10016=AXIS2_PLACEMENT_3D('',#43638,#12078,#12079);
#10017=AXIS2_PLACEMENT_3D('',#43642,#12081,#12082);
#10018=AXIS2_PLACEMENT_3D('',#43646,#12084,#12085);
#10019=AXIS2_PLACEMENT_3D('',#43648,#12086,#12087);
#10020=AXIS2_PLACEMENT_3D('',#43651,#12089,#12090);
#10021=AXIS2_PLACEMENT_3D('',#43652,#12091,#12092);
#10022=AXIS2_PLACEMENT_3D('',#43654,#12093,#12094);
#10023=AXIS2_PLACEMENT_3D('',#43656,#12096,#12097);
#10024=AXIS2_PLACEMENT_3D('',#43661,#12099,#12100);
#10025=AXIS2_PLACEMENT_3D('',#43664,#12102,#12103);
#10026=AXIS2_PLACEMENT_3D('',#43665,#12104,#12105);
#10027=AXIS2_PLACEMENT_3D('',#43667,#12106,#12107);
#10028=AXIS2_PLACEMENT_3D('',#43822,#12109,#12110);
#10029=AXIS2_PLACEMENT_3D('',#43824,#12111,#12112);
#10030=AXIS2_PLACEMENT_3D('',#43839,#12113,#12114);
#10031=AXIS2_PLACEMENT_3D('',#43841,#12115,#12116);
#10032=AXIS2_PLACEMENT_3D('',#43842,#12117,#12118);
#10033=AXIS2_PLACEMENT_3D('',#43905,#12119,#12120);
#10034=AXIS2_PLACEMENT_3D('',#44049,#12121,#12122);
#10035=AXIS2_PLACEMENT_3D('',#44052,#12123,#12124);
#10036=AXIS2_PLACEMENT_3D('',#44055,#12127,#12128);
#10037=AXIS2_PLACEMENT_3D('',#44056,#12129,#12130);
#10038=AXIS2_PLACEMENT_3D('',#44057,#12131,#12132);
#10039=AXIS2_PLACEMENT_3D('',#44058,#12133,#12134);
#10040=AXIS2_PLACEMENT_3D('',#44061,#12136,#12137);
#10041=AXIS2_PLACEMENT_3D('',#44062,#12138,#12139);
#10042=AXIS2_PLACEMENT_3D('',#44066,#12142,#12143);
#10043=AXIS2_PLACEMENT_3D('',#44067,#12144,#12145);
#10044=AXIS2_PLACEMENT_3D('',#44068,#12146,#12147);
#10045=AXIS2_PLACEMENT_3D('',#44069,#12148,#12149);
#10046=AXIS2_PLACEMENT_3D('',#44070,#12150,#12151);
#10047=AXIS2_PLACEMENT_3D('',#44072,#12152,#12153);
#10048=AXIS2_PLACEMENT_3D('',#44074,#12155,#12156);
#10049=AXIS2_PLACEMENT_3D('',#44075,#12157,#12158);
#10050=AXIS2_PLACEMENT_3D('',#44076,#12159,#12160);
#10051=AXIS2_PLACEMENT_3D('',#44079,#12162,#12163);
#10052=AXIS2_PLACEMENT_3D('',#44080,#12164,#12165);
#10053=AXIS2_PLACEMENT_3D('',#44082,#12167,#12168);
#10054=AXIS2_PLACEMENT_3D('',#44084,#12169,#12170);
#10055=AXIS2_PLACEMENT_3D('',#44086,#12172,#12173);
#10056=AXIS2_PLACEMENT_3D('',#44087,#12174,#12175);
#10057=AXIS2_PLACEMENT_3D('',#44088,#12176,#12177);
#10058=AXIS2_PLACEMENT_3D('',#44090,#12178,#12179);
#10059=AXIS2_PLACEMENT_3D('',#44091,#12180,#12181);
#10060=AXIS2_PLACEMENT_3D('',#44092,#12182,#12183);
#10061=AXIS2_PLACEMENT_3D('',#44094,#12184,#12185);
#10062=AXIS2_PLACEMENT_3D('',#44098,#12187,#12188);
#10063=AXIS2_PLACEMENT_3D('',#44100,#12190,#12191);
#10064=AXIS2_PLACEMENT_3D('',#44101,#12192,#12193);
#10065=AXIS2_PLACEMENT_3D('',#44102,#12194,#12195);
#10066=AXIS2_PLACEMENT_3D('',#44105,#12197,#12198);
#10067=AXIS2_PLACEMENT_3D('',#44106,#12199,#12200);
#10068=AXIS2_PLACEMENT_3D('',#44369,#12203,#12204);
#10069=AXIS2_PLACEMENT_3D('',#44371,#12205,#12206);
#10070=AXIS2_PLACEMENT_3D('',#44496,#12207,#12208);
#10071=AXIS2_PLACEMENT_3D('',#44497,#12209,#12210);
#10072=AXIS2_PLACEMENT_3D('',#44500,#12212,#12213);
#10073=AXIS2_PLACEMENT_3D('',#44540,#12214,#12215);
#10074=AXIS2_PLACEMENT_3D('',#44541,#12216,#12217);
#10075=AXIS2_PLACEMENT_3D('',#44545,#12219,#12220);
#10076=AXIS2_PLACEMENT_3D('',#44797,#12222,#12223);
#10077=AXIS2_PLACEMENT_3D('',#44842,#12224,#12225);
#10078=AXIS2_PLACEMENT_3D('',#44915,#12226,#12227);
#10079=AXIS2_PLACEMENT_3D('',#44973,#12228,#12229);
#10080=AXIS2_PLACEMENT_3D('',#45113,#12230,#12231);
#10081=AXIS2_PLACEMENT_3D('',#45181,#12232,#12233);
#10082=AXIS2_PLACEMENT_3D('',#45183,#12234,#12235);
#10083=AXIS2_PLACEMENT_3D('',#45196,#12237,#12238);
#10084=AXIS2_PLACEMENT_3D('',#45197,#12239,#12240);
#10085=AXIS2_PLACEMENT_3D('',#45198,#12241,#12242);
#10086=AXIS2_PLACEMENT_3D('',#45199,#12243,#12244);
#10087=AXIS2_PLACEMENT_3D('',#45204,#12247,#12248);
#10088=AXIS2_PLACEMENT_3D('',#45207,#12250,#12251);
#10089=AXIS2_PLACEMENT_3D('',#45208,#12252,#12253);
#10090=AXIS2_PLACEMENT_3D('',#45210,#12254,#12255);
#10091=AXIS2_PLACEMENT_3D('',#45212,#12257,#12258);
#10092=AXIS2_PLACEMENT_3D('',#45214,#12259,#12260);
#10093=AXIS2_PLACEMENT_3D('',#45215,#12261,#12262);
#10094=AXIS2_PLACEMENT_3D('',#45217,#12263,#12264);
#10095=AXIS2_PLACEMENT_3D('',#45220,#12267,#12268);
#10096=AXIS2_PLACEMENT_3D('',#45223,#12269,#12270);
#10097=AXIS2_PLACEMENT_3D('',#45227,#12272,#12273);
#10098=AXIS2_PLACEMENT_3D('',#45231,#12275,#12276);
#10099=AXIS2_PLACEMENT_3D('',#45234,#12279,#12280);
#10100=AXIS2_PLACEMENT_3D('',#45237,#12283,#12284);
#10101=AXIS2_PLACEMENT_3D('',#45238,#12285,#12286);
#10102=AXIS2_PLACEMENT_3D('',#45242,#12289,#12290);
#10103=AXIS2_PLACEMENT_3D('',#45243,#12291,#12292);
#10104=AXIS2_PLACEMENT_3D('',#45440,#12293,#12294);
#10105=AXIS2_PLACEMENT_3D('',#45528,#12295,#12296);
#10106=AXIS2_PLACEMENT_3D('',#45529,#12297,#12298);
#10107=AXIS2_PLACEMENT_3D('',#45530,#12299,#12300);
#10108=AXIS2_PLACEMENT_3D('',#45535,#12304,#12305);
#10109=AXIS2_PLACEMENT_3D('',#45536,#12306,#12307);
#10110=AXIS2_PLACEMENT_3D('',#45646,#12309,#12310);
#10111=AXIS2_PLACEMENT_3D('',#45706,#12311,#12312);
#10112=AXIS2_PLACEMENT_3D('',#45707,#12313,#12314);
#10113=AXIS2_PLACEMENT_3D('',#45711,#12317,#12318);
#10114=AXIS2_PLACEMENT_3D('',#45712,#12319,#12320);
#10115=AXIS2_PLACEMENT_3D('',#45746,#12321,#12322);
#10116=AXIS2_PLACEMENT_3D('',#45747,#12323,#12324);
#10117=AXIS2_PLACEMENT_3D('',#45941,#12325,#12326);
#10118=AXIS2_PLACEMENT_3D('',#46030,#12327,#12328);
#10119=AXIS2_PLACEMENT_3D('',#46034,#12331,#12332);
#10120=AXIS2_PLACEMENT_3D('',#46035,#12333,#12334);
#10121=AXIS2_PLACEMENT_3D('',#46036,#12335,#12336);
#10122=AXIS2_PLACEMENT_3D('',#46037,#12337,#12338);
#10123=AXIS2_PLACEMENT_3D('',#46038,#12339,#12340);
#10124=AXIS2_PLACEMENT_3D('',#46039,#12341,#12342);
#10125=AXIS2_PLACEMENT_3D('',#46040,#12343,#12344);
#10126=AXIS2_PLACEMENT_3D('',#46041,#12345,#12346);
#10127=AXIS2_PLACEMENT_3D('',#46042,#12347,#12348);
#10128=AXIS2_PLACEMENT_3D('',#46043,#12349,#12350);
#10129=AXIS2_PLACEMENT_3D('',#46044,#12351,#12352);
#10130=AXIS2_PLACEMENT_3D('',#46045,#12353,#12354);
#10131=AXIS2_PLACEMENT_3D('',#46046,#12355,#12356);
#11998=DIRECTION('axis',(0.,0.,1.));
#11999=DIRECTION('refdir',(1.,0.,0.));
#12000=DIRECTION('center_axis',(1.,0.,0.));
#12001=DIRECTION('ref_axis',(0.,0.,1.));
#12002=DIRECTION('',(0.,-1.,0.));
#12003=DIRECTION('',(-1.134075269297E-9,-1.795971255033E-10,-1.));
#12004=DIRECTION('',(-4.42567343416081E-9,0.999999999992356,3.90988426483683E-6));
#12005=DIRECTION('',(-2.32692945446299E-8,0.999999999999997,-6.98070862355898E-8));
#12006=DIRECTION('center_axis',(1.,0.,0.));
#12007=DIRECTION('ref_axis',(0.,0.,1.));
#12008=DIRECTION('center_axis',(-1.,0.,0.));
#12009=DIRECTION('ref_axis',(0.,-1.,0.));
#12010=DIRECTION('center_axis',(-1.,0.,0.));
#12011=DIRECTION('ref_axis',(0.,-0.999934254603685,-0.0114667549975298));
#12012=DIRECTION('center_axis',(-1.,0.,0.));
#12013=DIRECTION('ref_axis',(0.,-1.,0.));
#12014=DIRECTION('center_axis',(-1.,0.,0.));
#12015=DIRECTION('ref_axis',(0.,-1.,0.));
#12016=DIRECTION('center_axis',(0.,-0.0114667549975297,0.999934254603685));
#12017=DIRECTION('ref_axis',(0.,0.999934254603685,0.0114667549975297));
#12018=DIRECTION('center_axis',(-1.,0.,0.));
#12019=DIRECTION('ref_axis',(0.,1.,0.));
#12020=DIRECTION('center_axis',(-1.,0.,0.));
#12021=DIRECTION('ref_axis',(0.,1.,0.));
#12022=DIRECTION('',(1.,0.,0.));
#12023=DIRECTION('center_axis',(-1.,0.,0.));
#12024=DIRECTION('ref_axis',(0.,1.,0.));
#12025=DIRECTION('center_axis',(1.,0.,0.));
#12026=DIRECTION('ref_axis',(0.,-1.,0.));
#12027=DIRECTION('center_axis',(-1.,0.,0.));
#12028=DIRECTION('ref_axis',(0.,0.,-1.));
#12029=DIRECTION('center_axis',(-1.,0.,0.));
#12030=DIRECTION('ref_axis',(0.,-0.866025403784429,0.500000000000017));
#12031=DIRECTION('center_axis',(-1.,0.,0.));
#12032=DIRECTION('ref_axis',(0.,-0.866025403784429,0.500000000000017));
#12033=DIRECTION('',(-1.,0.,0.));
#12034=DIRECTION('center_axis',(-1.,0.,0.));
#12035=DIRECTION('ref_axis',(0.,0.,-1.));
#12036=DIRECTION('center_axis',(-1.,0.,0.));
#12037=DIRECTION('ref_axis',(0.,-1.,0.));
#12038=DIRECTION('',(-1.,0.,0.));
#12039=DIRECTION('',(-1.,0.,0.));
#12040=DIRECTION('center_axis',(-1.,0.,0.));
#12041=DIRECTION('ref_axis',(0.,0.,-1.));
#12042=DIRECTION('',(0.500000000000004,-0.750000000000006,-0.433012701892204));
#12043=DIRECTION('',(0.500000000000004,0.750000000000006,0.433012701892204));
#12044=DIRECTION('',(1.,0.,0.));
#12045=DIRECTION('',(1.,0.,0.));
#12046=DIRECTION('',(0.500000000000004,0.750000000000006,-0.433012701892204));
#12047=DIRECTION('',(0.500000000000004,-0.750000000000006,0.433012701892204));
#12048=DIRECTION('',(0.500000000000017,0.,-0.866025403784429));
#12049=DIRECTION('',(0.500000000000017,1.24992574614904E-14,0.866025403784429));
#12050=DIRECTION('',(1.,0.,0.));
#12051=DIRECTION('center_axis',(0.,-0.500000000000017,0.866025403784429));
#12052=DIRECTION('ref_axis',(0.,-0.866025403784429,-0.500000000000017));
#12053=DIRECTION('center_axis',(1.,0.,0.));
#12054=DIRECTION('ref_axis',(0.,0.,1.));
#12055=DIRECTION('center_axis',(1.,0.,0.));
#12056=DIRECTION('ref_axis',(0.,0.,1.));
#12057=DIRECTION('center_axis',(1.,0.,0.));
#12058=DIRECTION('ref_axis',(0.,0.,1.));
#12059=DIRECTION('',(1.,0.,0.));
#12060=DIRECTION('center_axis',(1.,0.,0.));
#12061=DIRECTION('ref_axis',(0.,0.,1.));
#12062=DIRECTION('center_axis',(1.,0.,0.));
#12063=DIRECTION('ref_axis',(0.,0.,1.));
#12064=DIRECTION('center_axis',(1.,0.,0.));
#12065=DIRECTION('ref_axis',(0.,0.,1.));
#12066=DIRECTION('center_axis',(1.,0.,0.));
#12067=DIRECTION('ref_axis',(0.,0.,1.));
#12068=DIRECTION('',(1.,0.,0.));
#12069=DIRECTION('center_axis',(1.,0.,0.));
#12070=DIRECTION('ref_axis',(0.,0.,1.));
#12071=DIRECTION('center_axis',(1.,0.,0.));
#12072=DIRECTION('ref_axis',(0.,0.,1.));
#12073=DIRECTION('',(-1.419652628015E-8,-1.,0.));
#12074=DIRECTION('',(0.,-3.273726813475E-12,-1.));
#12075=DIRECTION('',(0.,1.,0.));
#12076=DIRECTION('center_axis',(-1.,0.,0.));
#12077=DIRECTION('ref_axis',(0.,-0.181670789891997,0.983359407388783));
#12078=DIRECTION('center_axis',(1.,0.,0.));
#12079=DIRECTION('ref_axis',(0.,-0.500000000000017,-0.866025403784429));
#12080=DIRECTION('',(0.,0.866025403790389,-0.499999999989694));
#12081=DIRECTION('center_axis',(-1.,0.,0.));
#12082=DIRECTION('ref_axis',(0.,-0.866025403784429,-0.500000000000017));
#12083=DIRECTION('',(0.,-0.499999999989307,0.866025403790612));
#12084=DIRECTION('center_axis',(1.,0.,0.));
#12085=DIRECTION('ref_axis',(0.,0.983359407388783,-0.181670789891997));
#12086=DIRECTION('center_axis',(-1.,0.,0.));
#12087=DIRECTION('ref_axis',(0.,0.,-1.));
#12088=DIRECTION('',(-2.63758496709599E-8,-0.999999999999996,7.91298651712797E-8));
#12089=DIRECTION('center_axis',(-1.,0.,0.));
#12090=DIRECTION('ref_axis',(0.,0.,-1.));
#12091=DIRECTION('center_axis',(1.,0.,0.));
#12092=DIRECTION('ref_axis',(0.,0.,-1.));
#12093=DIRECTION('center_axis',(-1.,0.,0.));
#12094=DIRECTION('ref_axis',(0.,0.,-1.));
#12095=DIRECTION('',(1.,0.,0.));
#12096=DIRECTION('center_axis',(1.,0.,0.));
#12097=DIRECTION('ref_axis',(0.,0.,-1.));
#12098=DIRECTION('',(5.13413878158674E-11,0.866025574454957,-0.499999704389875));
#12099=DIRECTION('center_axis',(1.,0.,0.));
#12100=DIRECTION('ref_axis',(0.,-0.399559341953183,0.91670733184476));
#12101=DIRECTION('',(6.42234657013179E-12,-0.499999694960384,0.866025579899072));
#12102=DIRECTION('center_axis',(-1.,0.,0.));
#12103=DIRECTION('ref_axis',(0.,-0.866025403784429,-0.500000000000017));
#12104=DIRECTION('center_axis',(0.,0.866025403784429,-0.500000000000017));
#12105=DIRECTION('ref_axis',(-1.,0.,0.));
#12106=DIRECTION('center_axis',(0.,0.866025403784429,-0.500000000000017));
#12107=DIRECTION('ref_axis',(-1.,0.,0.));
#12108=DIRECTION('',(0.,-0.866025403784429,0.500000000000017));
#12109=DIRECTION('center_axis',(0.,0.916707576755026,0.399558780056111));
#12110=DIRECTION('ref_axis',(1.,6.74402148298192E-13,-1.54728062548894E-12));
#12111=DIRECTION('center_axis',(1.,0.,0.));
#12112=DIRECTION('ref_axis',(0.,-0.500000000000017,-0.866025403784429));
#12113=DIRECTION('center_axis',(1.,0.,0.));
#12114=DIRECTION('ref_axis',(0.,0.999999564444476,0.000933333197827078));
#12115=DIRECTION('center_axis',(0.,0.399559341952196,0.91670733184519));
#12116=DIRECTION('ref_axis',(1.,0.,0.));
#12117=DIRECTION('center_axis',(1.,0.,0.));
#12118=DIRECTION('ref_axis',(0.,-0.399559341953183,0.91670733184476));
#12119=DIRECTION('center_axis',(-1.,0.,0.));
#12120=DIRECTION('ref_axis',(0.,0.866025403784429,0.500000000000017));
#12121=DIRECTION('center_axis',(1.,0.,0.));
#12122=DIRECTION('ref_axis',(0.,0.983359407388783,-0.181670789891997));
#12123=DIRECTION('center_axis',(1.,0.,0.));
#12124=DIRECTION('ref_axis',(0.,0.983359407388783,-0.181670789891997));
#12125=DIRECTION('',(-1.,9.103769590032E-11,-1.576833478604E-10));
#12126=DIRECTION('',(1.,-3.095953123496E-11,-1.675853530022E-10));
#12127=DIRECTION('center_axis',(1.,0.,0.));
#12128=DIRECTION('ref_axis',(0.,0.969024744073282,-0.246963651928195));
#12129=DIRECTION('center_axis',(0.,0.181670789891997,0.983359407388783));
#12130=DIRECTION('ref_axis',(0.,-0.983359407388783,0.181670789891997));
#12131=DIRECTION('center_axis',(0.,-0.500000000000017,0.866025403784429));
#12132=DIRECTION('ref_axis',(0.,-0.866025403784429,-0.500000000000017));
#12133=DIRECTION('center_axis',(0.,-0.500000000000017,0.866025403784429));
#12134=DIRECTION('ref_axis',(0.,-0.866025403784429,-0.500000000000017));
#12135=DIRECTION('',(0.,-0.500000000000017,0.866025403784429));
#12136=DIRECTION('center_axis',(0.,-0.500000000000017,0.866025403784429));
#12137=DIRECTION('ref_axis',(0.,-0.866025403784429,-0.500000000000017));
#12138=DIRECTION('center_axis',(0.,-0.866025403784429,-0.500000000000017));
#12139=DIRECTION('ref_axis',(0.,0.500000000000017,-0.866025403784429));
#12140=DIRECTION('',(-1.,2.030967986381E-12,-3.514818066227E-12));
#12141=DIRECTION('',(0.,0.500000000000017,-0.866025403784429));
#12142=DIRECTION('center_axis',(0.,-0.500000000000017,0.866025403784429));
#12143=DIRECTION('ref_axis',(-1.,0.,0.));
#12144=DIRECTION('center_axis',(0.,-0.500000000000017,0.866025403784429));
#12145=DIRECTION('ref_axis',(-1.,0.,0.));
#12146=DIRECTION('center_axis',(1.,0.,0.));
#12147=DIRECTION('ref_axis',(0.,-0.850531242834003,-0.525924524017702));
#12148=DIRECTION('center_axis',(-1.,0.,0.));
#12149=DIRECTION('ref_axis',(0.,-0.866025403784429,-0.500000000000017));
#12150=DIRECTION('center_axis',(1.,0.,0.));
#12151=DIRECTION('ref_axis',(0.,-0.707106781187104,0.707106781185991));
#12152=DIRECTION('center_axis',(-1.,0.,0.));
#12153=DIRECTION('ref_axis',(0.,-0.866025403784429,-0.500000000000017));
#12154=DIRECTION('',(-1.,-2.646771690706E-13,1.515824502955E-13));
#12155=DIRECTION('center_axis',(1.,0.,0.));
#12156=DIRECTION('ref_axis',(0.,-0.855623464285791,-0.517598770635694));
#12157=DIRECTION('center_axis',(0.,0.866025403784429,-0.500000000000017));
#12158=DIRECTION('ref_axis',(0.,0.500000000000017,0.866025403784429));
#12159=DIRECTION('center_axis',(0.,0.866025403784429,-0.500000000000017));
#12160=DIRECTION('ref_axis',(0.,0.500000000000017,0.866025403784429));
#12161=DIRECTION('',(0.,0.866025403784429,-0.500000000000017));
#12162=DIRECTION('center_axis',(0.,0.866025403784429,-0.500000000000017));
#12163=DIRECTION('ref_axis',(0.,0.500000000000017,0.866025403784429));
#12164=DIRECTION('center_axis',(0.,0.500000000000017,0.866025403784429));
#12165=DIRECTION('ref_axis',(0.,-0.866025403784429,0.500000000000017));
#12166=DIRECTION('',(1.,-1.516879954977E-10,8.757853701506E-11));
#12167=DIRECTION('center_axis',(-1.,0.,0.));
#12168=DIRECTION('ref_axis',(0.,0.181670789891997,-0.983359407388783));
#12169=DIRECTION('center_axis',(1.,0.,0.));
#12170=DIRECTION('ref_axis',(0.,-0.500000000000017,-0.866025403784429));
#12171=DIRECTION('',(-1.,-1.747034739097E-10,-3.227581165296E-11));
#12172=DIRECTION('center_axis',(-1.,0.,0.));
#12173=DIRECTION('ref_axis',(0.,-0.552140107391307,-0.833751342913411));
#12174=DIRECTION('center_axis',(0.,0.983359407388783,0.181670789891997));
#12175=DIRECTION('ref_axis',(0.,-0.181670789891997,0.983359407388783));
#12176=DIRECTION('center_axis',(1.,0.,0.));
#12177=DIRECTION('ref_axis',(0.,-0.0912156582260493,0.995831162243073));
#12178=DIRECTION('center_axis',(-1.,0.,0.));
#12179=DIRECTION('ref_axis',(0.,-0.181670789891997,0.983359407388783));
#12180=DIRECTION('center_axis',(0.,1.,0.));
#12181=DIRECTION('ref_axis',(0.,0.,1.));
#12182=DIRECTION('center_axis',(1.,0.,0.));
#12183=DIRECTION('ref_axis',(0.,0.,1.));
#12184=DIRECTION('center_axis',(-1.,0.,0.));
#12185=DIRECTION('ref_axis',(0.,0.,-1.));
#12186=DIRECTION('',(1.,0.,0.));
#12187=DIRECTION('center_axis',(1.,0.,0.));
#12188=DIRECTION('ref_axis',(0.,0.,1.));
#12189=DIRECTION('',(1.,0.,0.));
#12190=DIRECTION('center_axis',(1.,0.,0.));
#12191=DIRECTION('ref_axis',(0.,0.0076661909649299,-0.999970614326286));
#12192=DIRECTION('center_axis',(0.,-1.,0.));
#12193=DIRECTION('ref_axis',(0.,0.,-1.));
#12194=DIRECTION('center_axis',(0.,-1.,0.));
#12195=DIRECTION('ref_axis',(0.,0.,-1.));
#12196=DIRECTION('',(-8.96449889951894E-8,-0.999999999999993,7.91296186399094E-8));
#12197=DIRECTION('center_axis',(0.,-1.,0.));
#12198=DIRECTION('ref_axis',(2.7385805267949E-7,0.,-0.999999999999963));
#12199=DIRECTION('center_axis',(0.,0.,-1.));
#12200=DIRECTION('ref_axis',(0.,1.,0.));
#12201=DIRECTION('',(3.87257253216599E-8,0.999999999999997,-6.98071249166998E-8));
#12202=DIRECTION('',(1.,0.,0.));
#12203=DIRECTION('center_axis',(1.,1.57229173603E-10,0.));
#12204=DIRECTION('ref_axis',(-1.55747353131272E-10,0.990575410162307,0.136968451775501));
#12205=DIRECTION('center_axis',(-0.0400339593305145,0.0439586138816482,
0.998230896319046));
#12206=DIRECTION('ref_axis',(0.672168878015028,-0.73800672205553,0.0594565188088726));
#12207=DIRECTION('center_axis',(-0.00691483422088646,-0.977373823122084,
-0.211406232035434));
#12208=DIRECTION('ref_axis',(0.995574959726093,0.0130842956657209,-0.0930553640222855));
#12209=DIRECTION('center_axis',(0.,-1.,0.));
#12210=DIRECTION('ref_axis',(0.992164397268247,0.,-0.124939220396706));
#12211=DIRECTION('',(5.416713864812E-14,1.,4.290037380931E-13));
#12212=DIRECTION('center_axis',(0.,-1.,0.));
#12213=DIRECTION('ref_axis',(0.992164397268247,0.,-0.124939220396706));
#12214=DIRECTION('center_axis',(0.,-0.993031974610984,-0.117845226463398));
#12215=DIRECTION('ref_axis',(0.991993011196462,0.0148830010065676,-0.125412766568694));
#12216=DIRECTION('center_axis',(-0.124870949205596,-0.0330540747897288,
-0.991622243691764));
#12217=DIRECTION('ref_axis',(-4.15466272496426E-16,0.999444906979154,-0.0333148302326418));
#12218=DIRECTION('',(-0.124870949205706,-0.0330540747749215,-0.991622243692244));
#12219=DIRECTION('center_axis',(0.,0.,-1.));
#12220=DIRECTION('ref_axis',(0.96670522786149,0.255892560316366,0.));
#12221=DIRECTION('',(-0.124870949205497,-0.0330540747897292,-0.991622243691777));
#12222=DIRECTION('center_axis',(-0.519150775460989,0.833954178873382,-0.187090619427796));
#12223=DIRECTION('ref_axis',(-0.854630432587176,-0.504108685418202,0.1244236994378));
#12224=DIRECTION('center_axis',(0.,-0.979738498904873,-0.200280987024795));
#12225=DIRECTION('ref_axis',(0.559356823890107,0.166018314377717,-0.812131678275607));
#12226=DIRECTION('center_axis',(0.,-0.964005425963159,-0.265882565644289));
#12227=DIRECTION('ref_axis',(0.391203692848694,0.244692820224845,-0.887178163861102));
#12228=DIRECTION('center_axis',(-0.821166253638671,0.530754423774481,0.209727741438393));
#12229=DIRECTION('ref_axis',(-0.523347833413461,-0.846903765812651,0.0941331860386426));
#12230=DIRECTION('center_axis',(0.959966443903985,-7.32732351878489E-7,
0.280115023834496));
#12231=DIRECTION('ref_axis',(0.257680928625254,0.392129214826704,-0.883082792212723));
#12232=DIRECTION('center_axis',(0.,0.,1.));
#12233=DIRECTION('ref_axis',(0.707106785728413,0.707106776644682,0.));
#12234=DIRECTION('center_axis',(0.,0.,1.));
#12235=DIRECTION('ref_axis',(1.,0.,0.));
#12236=DIRECTION('',(-8.269906478952E-12,0.,-1.));
#12237=DIRECTION('center_axis',(0.,0.,1.));
#12238=DIRECTION('ref_axis',(1.,0.,0.));
#12239=DIRECTION('center_axis',(0.,1.,0.));
#12240=DIRECTION('ref_axis',(0.,0.,1.));
#12241=DIRECTION('center_axis',(-1.,0.,0.));
#12242=DIRECTION('ref_axis',(0.,0.,1.));
#12243=DIRECTION('center_axis',(0.,0.,1.));
#12244=DIRECTION('ref_axis',(0.,-1.,0.));
#12245=DIRECTION('',(0.,1.,0.));
#12246=DIRECTION('',(-1.,0.,0.));
#12247=DIRECTION('center_axis',(0.,0.,1.));
#12248=DIRECTION('ref_axis',(0.,1.,0.));
#12249=DIRECTION('',(0.,-1.,0.));
#12250=DIRECTION('center_axis',(0.,0.,1.));
#12251=DIRECTION('ref_axis',(0.,-1.,0.));
#12252=DIRECTION('center_axis',(0.,0.,1.));
#12253=DIRECTION('ref_axis',(0.,-1.,0.));
#12254=DIRECTION('center_axis',(0.,0.,1.));
#12255=DIRECTION('ref_axis',(0.,-1.,0.));
#12256=DIRECTION('',(0.,0.,1.));
#12257=DIRECTION('center_axis',(0.,0.,1.));
#12258=DIRECTION('ref_axis',(0.,-1.,0.));
#12259=DIRECTION('center_axis',(0.,0.,1.));
#12260=DIRECTION('ref_axis',(0.,1.,0.));
#12261=DIRECTION('center_axis',(0.,0.,1.));
#12262=DIRECTION('ref_axis',(0.,1.,0.));
#12263=DIRECTION('center_axis',(0.,0.,1.));
#12264=DIRECTION('ref_axis',(0.,-1.,0.));
#12265=DIRECTION('',(0.,0.,1.));
#12266=DIRECTION('',(0.,0.,1.));
#12267=DIRECTION('center_axis',(0.,0.,-1.));
#12268=DIRECTION('ref_axis',(0.,-1.,0.));
#12269=DIRECTION('center_axis',(0.,0.,1.));
#12270=DIRECTION('ref_axis',(0.673329668846713,-0.739342381478822,0.));
#12271=DIRECTION('',(-1.,0.,0.));
#12272=DIRECTION('center_axis',(0.,0.,-1.));
#12273=DIRECTION('ref_axis',(-0.313683251850025,-0.949527681275693,0.));
#12274=DIRECTION('',(0.,-1.,0.));
#12275=DIRECTION('center_axis',(0.,0.,1.));
#12276=DIRECTION('ref_axis',(-0.80779094785921,0.589469070059421,0.));
#12277=DIRECTION('',(-1.,0.,0.));
#12278=DIRECTION('',(0.,-1.,0.));
#12279=DIRECTION('center_axis',(0.123779845007298,-0.135915123929598,0.982957592705388));
#12280=DIRECTION('ref_axis',(9.61036805691157E-16,-0.990575410162308,-0.136968451775493));
#12281=DIRECTION('',(0.123779845007102,-0.135915123929602,0.982957592705412));
#12282=DIRECTION('',(0.123779534119897,-0.135915212762297,0.982957619571078));
#12283=DIRECTION('center_axis',(-0.992164397268247,0.,0.124939220396706));
#12284=DIRECTION('ref_axis',(0.124939220396706,0.,0.992164397268247));
#12285=DIRECTION('center_axis',(0.,0.990575410162307,0.136968451775501));
#12286=DIRECTION('ref_axis',(0.,0.136968451775501,-0.990575410162307));
#12287=DIRECTION('',(1.,0.,0.));
#12288=DIRECTION('',(0.0452022558840394,0.136828450245298,-0.989562899095587));
#12289=DIRECTION('center_axis',(1.,0.,0.));
#12290=DIRECTION('ref_axis',(0.,0.990575410162307,0.136968451775501));
#12291=DIRECTION('center_axis',(1.,0.,0.));
#12292=DIRECTION('ref_axis',(0.,0.990575410162307,0.136968451775501));
#12293=DIRECTION('center_axis',(0.0147910789458937,0.0447731623135355,0.998887675326942));
#12294=DIRECTION('ref_axis',(-0.313280857521534,-0.948489162952014,0.0471530706652296));
#12295=DIRECTION('center_axis',(0.,0.999999999999929,-3.77402948630611E-7));
#12296=DIRECTION('ref_axis',(1.16229440341503E-7,-3.77402948630608E-7,-0.999999999999922));
#12297=DIRECTION('center_axis',(0.0209905750013486,0.971496035276488,-0.236124647597782));
#12298=DIRECTION('ref_axis',(-0.0900783656611823,0.237053837004821,0.967311411284444));
#12299=DIRECTION('center_axis',(0.998958343750615,0.,0.0456314305170007));
#12300=DIRECTION('ref_axis',(0.0456314305170007,0.,-0.998958343750615));
#12301=DIRECTION('',(1.30063660726595E-7,0.999999999996163,-2.7670341656329E-6));
#12302=DIRECTION('',(-0.0456061512274497,0.0332801611178298,0.998404982883294));
#12303=DIRECTION('',(0.0452020303481621,0.136828427182506,-0.989562912586747));
#12304=DIRECTION('center_axis',(0.0452022558846083,0.136828450245295,-0.989562899095562));
#12305=DIRECTION('ref_axis',(4.63171168085811E-16,-0.990575410162305,-0.136968451775511));
#12306=DIRECTION('center_axis',(-0.045606153526751,0.0332801660870907,0.998404982612622));
#12307=DIRECTION('ref_axis',(1.51788304147964E-16,0.999444906979154,-0.0333148302326418));
#12308=DIRECTION('',(-0.0456061527666419,0.0332801651001014,0.998404982680243));
#12309=DIRECTION('center_axis',(-0.00599371100089924,0.993987697016237,
0.109327643388101));
#12310=DIRECTION('ref_axis',(-0.0158677933944027,-0.109410380526878,0.993870002447884));
#12311=DIRECTION('center_axis',(0.997994746578697,0.000832709485814794,
-0.0632913295502143));
#12312=DIRECTION('ref_axis',(0.059454730773529,-0.355397842285051,0.932822335006928));
#12313=DIRECTION('center_axis',(1.,0.,0.));
#12314=DIRECTION('ref_axis',(0.,0.999444906979154,-0.0333148302326385));
#12315=DIRECTION('',(0.999999999999499,3.543019115023E-8,1.000251741924E-6));
#12316=DIRECTION('',(0.999999999999606,-2.05591310759001E-9,-8.87615856965605E-7));
#12317=DIRECTION('center_axis',(0.999999999998528,0.,-1.71571223939805E-6));
#12318=DIRECTION('ref_axis',(-5.71586619530014E-8,0.999444906979749,-0.0333148302147516));
#12319=DIRECTION('center_axis',(0.,-0.999444906979154,0.0333148302326385));
#12320=DIRECTION('ref_axis',(0.,0.0333148302326385,0.999444906979154));
#12321=DIRECTION('center_axis',(-8.77617113914048E-11,-1.,1.28881744793477E-9));
#12322=DIRECTION('ref_axis',(0.994676936356327,4.5508643513665E-11,0.103042672135346));
#12323=DIRECTION('center_axis',(0.992288436659883,0.,0.123950225780698));
#12324=DIRECTION('ref_axis',(0.00423001996726221,0.999417512380893,-0.03386359221145));
#12325=DIRECTION('center_axis',(0.97803698136698,0.,0.208431434957796));
#12326=DIRECTION('ref_axis',(0.170039536409224,0.578326194595119,-0.797888067778222));
#12327=DIRECTION('center_axis',(0.,1.,0.));
#12328=DIRECTION('ref_axis',(0.,0.,1.));
#12329=DIRECTION('',(-1.,0.,0.));
#12330=DIRECTION('',(3.309808819951E-11,5.093238724031E-10,-1.));
#12331=DIRECTION('center_axis',(-1.,0.,0.));
#12332=DIRECTION('ref_axis',(0.,0.,1.));
#12333=DIRECTION('center_axis',(-1.,0.,0.));
#12334=DIRECTION('ref_axis',(0.,0.,1.));
#12335=DIRECTION('center_axis',(0.,0.,-1.));
#12336=DIRECTION('ref_axis',(0.0301983768555915,0.999543925015448,0.));
#12337=DIRECTION('center_axis',(0.,0.,1.));
#12338=DIRECTION('ref_axis',(0.,1.,0.));
#12339=DIRECTION('center_axis',(0.,-1.,0.));
#12340=DIRECTION('ref_axis',(0.,0.,1.));
#12341=DIRECTION('center_axis',(0.,-1.,0.));
#12342=DIRECTION('ref_axis',(0.,0.,1.));
#12343=DIRECTION('center_axis',(0.,-1.,0.));
#12344=DIRECTION('ref_axis',(0.,0.,1.));
#12345=DIRECTION('center_axis',(1.,0.,0.));
#12346=DIRECTION('ref_axis',(0.,-1.,1.24367530163205E-13));
#12347=DIRECTION('center_axis',(0.,1.,0.));
#12348=DIRECTION('ref_axis',(0.,0.,-1.));
#12349=DIRECTION('center_axis',(0.,1.,0.));
#12350=DIRECTION('ref_axis',(0.,0.,-1.));
#12351=DIRECTION('center_axis',(0.,0.,-1.));
#12352=DIRECTION('ref_axis',(-1.,0.,0.));
#12353=DIRECTION('center_axis',(0.,1.,0.));
#12354=DIRECTION('ref_axis',(-0.998958343750615,0.,-0.0456314305170007));
#12355=DIRECTION('center_axis',(0.,1.,0.));
#12356=DIRECTION('ref_axis',(0.,0.,1.));
#39898=CARTESIAN_POINT('',(0.,0.,0.));
#39899=CARTESIAN_POINT('Origin',(-4.6,0.,0.));
#39900=CARTESIAN_POINT('',(-4.6,10.41,7.5));
#39901=CARTESIAN_POINT('',(-4.6,1.41,7.5));
#39902=CARTESIAN_POINT('',(-4.6,10.40999999984,7.5));
#39903=CARTESIAN_POINT('',(-4.6000000442632,10.4099999970609,-7.98856626783461));
#39904=CARTESIAN_POINT('',(-4.6,10.40999999984,7.5));
#39905=CARTESIAN_POINT('',(-4.599999995006,5.31268601529799,-7.988586197742));
#39906=CARTESIAN_POINT('',(-4.599999995006,5.312686015298,-7.988586197742));
#39907=CARTESIAN_POINT('',(-4.60000008479568,3.59647899566988,-7.50000015263407));
#39908=CARTESIAN_POINT('Ctrl Pts',(-4.60000005087721,3.59647899566978,-7.50000015263649));
#39909=CARTESIAN_POINT('Ctrl Pts',(-4.59999986298528,3.70619272292874,-7.50000123432406));
#39910=CARTESIAN_POINT('Ctrl Pts',(-4.60000006358096,3.91406362288072,-7.51418484353807));
#39911=CARTESIAN_POINT('Ctrl Pts',(-4.599999982988,4.189476771086,-7.561416026773));
#39912=CARTESIAN_POINT('Ctrl Pts',(-4.600000004468,4.434127618739,-7.624029192647));
#39913=CARTESIAN_POINT('Ctrl Pts',(-4.599999999139,4.650710856925,-7.694659592193));
#39914=CARTESIAN_POINT('Ctrl Pts',(-4.599999998977,4.843005160611,-7.768527138287));
#39915=CARTESIAN_POINT('Ctrl Pts',(-4.600000004953,5.015100702816,-7.842916001697));
#39916=CARTESIAN_POINT('Ctrl Pts',(-4.599999981211,5.170593933842,-7.916289820707));
#39917=CARTESIAN_POINT('Ctrl Pts',(-4.60000004054,5.266673416514,-7.964776668264));
#39918=CARTESIAN_POINT('Ctrl Pts',(-4.599999995006,5.312686015298,-7.988586197742));
#39919=CARTESIAN_POINT('',(-4.6,1.41,-7.5));
#39920=CARTESIAN_POINT('',(-4.6,1.41,-7.5));
#39921=CARTESIAN_POINT('Origin',(-4.6,1.41,0.));
#39922=CARTESIAN_POINT('',(-4.6,7.40960552762211,0.0688005299851782));
#39923=CARTESIAN_POINT('Origin',(-4.6,1.41,0.));
#39924=CARTESIAN_POINT('Origin',(-5.6,1.41,0.));
#39925=CARTESIAN_POINT('',(-5.6,-3.59,0.));
#39926=CARTESIAN_POINT('',(-5.6,6.40967127301842,0.0573337749876485));
#39927=CARTESIAN_POINT('Origin',(-5.6,1.41,0.));
#39928=CARTESIAN_POINT('Origin',(-5.6,1.41,0.));
#39929=CARTESIAN_POINT('Origin',(-5.6,7.40960552762211,0.0688005299851782));
#39930=CARTESIAN_POINT('Origin',(-4.6,1.41,0.));
#39931=CARTESIAN_POINT('',(-14.6,-3.59,6.12323399573677E-16));
#39932=CARTESIAN_POINT('Origin',(-14.6,1.41,0.));
#39933=CARTESIAN_POINT('',(-4.6,-3.59,6.12323399573677E-16));
#39934=CARTESIAN_POINT('Origin',(-14.6,0.,0.));
#39935=CARTESIAN_POINT('',(-14.6,1.41,4.));
#39936=CARTESIAN_POINT('Origin',(-14.6,1.41,0.));
#39937=CARTESIAN_POINT('Origin',(-14.6,1.41,0.));
#39938=CARTESIAN_POINT('',(-12.599955217472,-2.05311064648514,2.00006051196135));
#39939=CARTESIAN_POINT('',(-12.6,1.41,4.));
#39940=CARTESIAN_POINT('Origin',(-12.6,1.41,0.));
#39941=CARTESIAN_POINT('Origin',(-12.6,1.41,0.));
#39942=CARTESIAN_POINT('',(-14.6,1.41,4.));
#39943=CARTESIAN_POINT('Origin',(-14.6,1.41,0.));
#39944=CARTESIAN_POINT('',(-3.1,1.41,4.));
#39945=CARTESIAN_POINT('Origin',(-3.1,1.41,0.));
#39946=CARTESIAN_POINT('',(-4.47396821277762,1.41,4.));
#39947=CARTESIAN_POINT('',(-14.6,1.41,4.));
#39948=CARTESIAN_POINT('',(-4.59999337538372,4.87352195157167,1.99964693648141));
#39949=CARTESIAN_POINT('Ctrl Pts',(-4.47396821277762,1.41,4.));
#39950=CARTESIAN_POINT('Ctrl Pts',(-4.47802321474399,1.55267489674965,4.));
#39951=CARTESIAN_POINT('Ctrl Pts',(-4.48213222009309,1.69531596101135,3.99236651952116));
#39952=CARTESIAN_POINT('Ctrl Pts',(-4.4906681550104,1.98294016555199,3.96146336088247));
#39953=CARTESIAN_POINT('Ctrl Pts',(-4.49509226438512,2.12759535602225,3.93783030862076));
#39954=CARTESIAN_POINT('Ctrl Pts',(-4.50494469986381,2.43962006156562,3.86908618594094));
#39955=CARTESIAN_POINT('Ctrl Pts',(-4.51040173745819,2.606018396681,3.82092707313125));
#39956=CARTESIAN_POINT('Ctrl Pts',(-4.52038860740983,2.90457634300073,3.71309713998014));
#39957=CARTESIAN_POINT('Ctrl Pts',(-4.5249123165038,3.03762834249849,3.65673024246835));
#39958=CARTESIAN_POINT('Ctrl Pts',(-4.53190546949731,3.24531722210745,3.55515752690714));
#39959=CARTESIAN_POINT('Ctrl Pts',(-4.53446142185042,3.32202920690643,3.51449549885797));
#39960=CARTESIAN_POINT('Ctrl Pts',(-4.54034315694366,3.49849701357434,3.41346772535774));
#39961=CARTESIAN_POINT('Ctrl Pts',(-4.54363691334612,3.59705824950081,3.35117270985553));
#39962=CARTESIAN_POINT('Ctrl Pts',(-4.55372497360401,3.89061373063259,3.1471588930267));
#39963=CARTESIAN_POINT('Ctrl Pts',(-4.56051176646417,4.07563514531634,2.99206294673198));
#39964=CARTESIAN_POINT('Ctrl Pts',(-4.57194713221524,4.34894837595383,2.71736344368141));
#39965=CARTESIAN_POINT('Ctrl Pts',(-4.57637475970776,4.44653251476823,2.60786314180913));
#39966=CARTESIAN_POINT('Ctrl Pts',(-4.58703999719547,4.66209483283886,2.33743206191275));
#39967=CARTESIAN_POINT('Ctrl Pts',(-4.59334861861747,4.77448463373213,2.1725445592894));
#39968=CARTESIAN_POINT('Ctrl Pts',(-4.59960196669704,4.87411610028898,1.99997491077231));
#39969=CARTESIAN_POINT('',(-3.84878783026703,4.87410161478956,1.99999999974644));
#39970=CARTESIAN_POINT('',(-3.85,4.874101615138,2.));
#39971=CARTESIAN_POINT('Ctrl Pts',(-3.84878782952482,4.87410161517191,1.99999999994084));
#39972=CARTESIAN_POINT('Ctrl Pts',(-3.85713541463281,5.00988343647519,1.76481898669005));
#39973=CARTESIAN_POINT('Ctrl Pts',(-3.86579655320577,5.12135499796743,1.516438340068));
#39974=CARTESIAN_POINT('Ctrl Pts',(-3.87700357702665,5.23571314511595,1.17147723100828));
#39975=CARTESIAN_POINT('Ctrl Pts',(-3.87979301326392,5.2616099576731,1.08330147408813));
#39976=CARTESIAN_POINT('Ctrl Pts',(-3.8875324253198,5.3267758384964,0.829374396988071));
#39977=CARTESIAN_POINT('Ctrl Pts',(-3.89232372159689,5.35852935393098,0.661901534699769));
#39978=CARTESIAN_POINT('Ctrl Pts',(-3.90164445511241,5.39933068569783,0.33332088901751));
#39979=CARTESIAN_POINT('Ctrl Pts',(-3.90616577556016,5.40950533665437,0.172680457019602));
#39980=CARTESIAN_POINT('Ctrl Pts',(-3.91485918785644,5.4103998948561,-0.128868547334375));
#39981=CARTESIAN_POINT('Ctrl Pts',(-3.91899728472511,5.403389775243,-0.269523734791878));
#39982=CARTESIAN_POINT('Ctrl Pts',(-3.92949010169241,5.36774660483486,-0.61584506126014));
#39983=CARTESIAN_POINT('Ctrl Pts',(-3.93596171182252,5.33049500919419,-0.820205843112968));
#39984=CARTESIAN_POINT('Ctrl Pts',(-3.94678581469179,5.2428813894696,-1.15216962797743));
#39985=CARTESIAN_POINT('Ctrl Pts',(-3.95108720632083,5.20151982219127,-1.28173804047728));
#39986=CARTESIAN_POINT('Ctrl Pts',(-3.95815429399473,5.12128476646775,-1.49492622583711));
#39987=CARTESIAN_POINT('Ctrl Pts',(-3.96096131409489,5.08597329433121,-1.57976605202262));
#39988=CARTESIAN_POINT('Ctrl Pts',(-3.96807606494566,4.98634724012396,-1.7976538191658));
#39989=CARTESIAN_POINT('Ctrl Pts',(-3.97227914857057,4.91752868463037,-1.92848733538));
#39990=CARTESIAN_POINT('Ctrl Pts',(-3.98146324970479,4.75069385577068,-2.20705429926935));
#39991=CARTESIAN_POINT('Ctrl Pts',(-3.98642774730493,4.6497812556587,-2.35268808037349));
#39992=CARTESIAN_POINT('Ctrl Pts',(-3.99578896820218,4.44727408042526,-2.60709077350989));
#39993=CARTESIAN_POINT('Ctrl Pts',(-4.00013752226369,4.34862331805883,-2.71780196259597));
#39994=CARTESIAN_POINT('Ctrl Pts',(-4.01175666237124,4.07623497223659,-2.99127849459317));
#39995=CARTESIAN_POINT('Ctrl Pts',(-4.01920284314558,3.8937221440456,-3.14446714373292));
#39996=CARTESIAN_POINT('Ctrl Pts',(-4.03039684119057,3.60194021417812,-3.34803162291242));
#39997=CARTESIAN_POINT('Ctrl Pts',(-4.03410508977674,3.50224692417008,-3.41121985721898));
#39998=CARTESIAN_POINT('Ctrl Pts',(-4.04043259544245,3.32413614929383,-3.51336192411137));
#39999=CARTESIAN_POINT('Ctrl Pts',(-4.04307908412172,3.24696082787826,-3.5543220716129));
#40000=CARTESIAN_POINT('Ctrl Pts',(-4.04985989702705,3.04053940671477,-3.65535752920676));
#40001=CARTESIAN_POINT('Ctrl Pts',(-4.05390375534371,2.90931869158175,-3.71111069265977));
#40002=CARTESIAN_POINT('Ctrl Pts',(-4.06284193540848,2.6119042658904,-3.81912070415939));
#40003=CARTESIAN_POINT('Ctrl Pts',(-4.06772160347664,2.44470973556781,-3.86776837074836));
#40004=CARTESIAN_POINT('Ctrl Pts',(-4.07694932757382,2.1317539852889,-3.937075200695));
#40005=CARTESIAN_POINT('Ctrl Pts',(-4.08125169467157,1.98699651538995,-3.9608791166392));
#40006=CARTESIAN_POINT('Ctrl Pts',(-4.09301151892351,1.59860160398172,-4.00299962462465));
#40007=CARTESIAN_POINT('Ctrl Pts',(-4.10066579918578,1.35404823912446,-4.00704862421727));
#40008=CARTESIAN_POINT('Ctrl Pts',(-4.11198140633078,0.995637385022808,
-3.98015192630208));
#40009=CARTESIAN_POINT('Ctrl Pts',(-4.11560712496378,0.881036526030751,
-3.96654810079726));
#40010=CARTESIAN_POINT('Ctrl Pts',(-4.12182572942684,0.681857405149143,
-3.93411767562979));
#40011=CARTESIAN_POINT('Ctrl Pts',(-4.12444412527263,0.597001844273346,
-3.9174620287807));
#40012=CARTESIAN_POINT('Ctrl Pts',(-4.13110257820161,0.377059353180721,
-3.86683599508181));
#40013=CARTESIAN_POINT('Ctrl Pts',(-4.13505818047302,0.243090662860835,
-3.82853903941916));
#40014=CARTESIAN_POINT('Ctrl Pts',(-4.14394891611014,-0.054486106748681,
-3.72639733363896));
#40015=CARTESIAN_POINT('Ctrl Pts',(-4.14886701052946,-0.21643691126297,
-3.65861438934144));
#40016=CARTESIAN_POINT('Ctrl Pts',(-4.15814707995622,-0.505052760626267,
-3.51485425923717));
#40017=CARTESIAN_POINT('Ctrl Pts',(-4.16246184930138,-0.632970335824287,
-3.44207759098763));
#40018=CARTESIAN_POINT('Ctrl Pts',(-4.17427317410496,-0.962885856764186,
-3.22949556864293));
#40019=CARTESIAN_POINT('Ctrl Pts',(-4.18196943446053,-1.15650713704172,
-3.07786656994227));
#40020=CARTESIAN_POINT('Ctrl Pts',(-4.19330963588578,-1.41854072582884,
-2.8306444192109));
#40021=CARTESIAN_POINT('Ctrl Pts',(-4.19691868971951,-1.49864594316486,
-2.74826667233921));
#40022=CARTESIAN_POINT('Ctrl Pts',(-4.2031172102864,-1.63257299550026,-2.59811580101652));
#40023=CARTESIAN_POINT('Ctrl Pts',(-4.20573170133228,-1.68795019061716,
-2.5318297690859));
#40024=CARTESIAN_POINT('Ctrl Pts',(-4.21379853036606,-1.85641204159948,
-2.31637107637409));
#40025=CARTESIAN_POINT('Ctrl Pts',(-4.21904724525982,-1.96119737707697,
-2.16103083840407));
#40026=CARTESIAN_POINT('Ctrl Pts',(-4.2304429640341,-2.16303601414209,-1.81118493732632));
#40027=CARTESIAN_POINT('Ctrl Pts',(-4.23659162406759,-2.25590822224409,
-1.61495872649002));
#40028=CARTESIAN_POINT('Ctrl Pts',(-4.24737437252633,-2.38473453489288,
-1.27355504778905));
#40029=CARTESIAN_POINT('Ctrl Pts',(-4.25185779501106,-2.4292993041449,-1.13213589537751));
#40030=CARTESIAN_POINT('Ctrl Pts',(-4.26197854844312,-2.5102892524769,-0.814597428677815));
#40031=CARTESIAN_POINT('Ctrl Pts',(-4.26765100744546,-2.54289827053674,
-0.637832512510027));
#40032=CARTESIAN_POINT('Ctrl Pts',(-4.27774887369803,-2.5798033346779,-0.318682236892733));
#40033=CARTESIAN_POINT('Ctrl Pts',(-4.28217494180975,-2.58858978675153,
-0.177116159811553));
#40034=CARTESIAN_POINT('Ctrl Pts',(-4.28926655321653,-2.59067481180548,
0.0585969388013058));
#40035=CARTESIAN_POINT('Ctrl Pts',(-4.29201068090646,-2.58819377611921,
0.152574799179403));
#40036=CARTESIAN_POINT('Ctrl Pts',(-4.29878578355939,-2.57367560802579,
0.387832894517081));
#40037=CARTESIAN_POINT('Ctrl Pts',(-4.30276284383635,-2.55743444386133,
0.52872530002292));
#40038=CARTESIAN_POINT('Ctrl Pts',(-4.31230255643117,-2.50096633200525,
0.861873716315035));
#40039=CARTESIAN_POINT('Ctrl Pts',(-4.31788348855111,-2.453999722358,1.05261009223179));
#40040=CARTESIAN_POINT('Ctrl Pts',(-4.327967578155,-2.34806572404957,1.37775114719943));
#40041=CARTESIAN_POINT('Ctrl Pts',(-4.33236795299842,-2.29535704235641,
1.51379776175824));
#40042=CARTESIAN_POINT('Ctrl Pts',(-4.34211297525343,-2.16517264423272,
1.80199710714394));
#40043=CARTESIAN_POINT('Ctrl Pts',(-4.34748378207211,-2.08514825905764,
1.95268789156043));
#40044=CARTESIAN_POINT('Ctrl Pts',(-4.35757777991757,-1.9169318958898,2.22578408856121));
#40045=CARTESIAN_POINT('Ctrl Pts',(-4.36229212032352,-1.83095405365336,
2.34921451452121));
#40046=CARTESIAN_POINT('Ctrl Pts',(-4.36947139588852,-1.68449076055774,
2.53608297090013));
#40047=CARTESIAN_POINT('Ctrl Pts',(-4.37203545870452,-1.62852322666058,
2.6028765715856));
#40048=CARTESIAN_POINT('Ctrl Pts',(-4.37795854739217,-1.49190155599502,
2.75550846278849));
#40049=CARTESIAN_POINT('Ctrl Pts',(-4.3812844372048,-1.40954893698499,2.83971899317701));
#40050=CARTESIAN_POINT('Ctrl Pts',(-4.39131853259455,-1.1499424513066,3.08273888832691));
#40051=CARTESIAN_POINT('Ctrl Pts',(-4.39802228460691,-0.962132639711373,
3.22948431899847));
#40052=CARTESIAN_POINT('Ctrl Pts',(-4.40935447792384,-0.639598163602044,
3.43810075559831));
#40053=CARTESIAN_POINT('Ctrl Pts',(-4.41377098264549,-0.512534997877063,
3.51073309565376));
#40054=CARTESIAN_POINT('Ctrl Pts',(-4.4235888209087,-0.22781721186987,3.65338347748354));
#40055=CARTESIAN_POINT('Ctrl Pts',(-4.4290180390454,-0.069032505004638,
3.72049959394663));
#40056=CARTESIAN_POINT('Ctrl Pts',(-4.43903876498291,0.231704694822792,
3.82531257514947));
#40057=CARTESIAN_POINT('Ctrl Pts',(-4.44362315896157,0.372369284968778,
3.86584013175734));
#40058=CARTESIAN_POINT('Ctrl Pts',(-4.45067549964498,0.599632867071186,
3.91801688464264));
#40059=CARTESIAN_POINT('Ctrl Pts',(-4.45323391251286,0.684937018050481,
3.93469628057976));
#40060=CARTESIAN_POINT('Ctrl Pts',(-4.45912820200206,0.886115422586876,
3.9672674116583));
#40061=CARTESIAN_POINT('Ctrl Pts',(-4.46243171505446,1.00227842112557,3.98088300670763));
#40062=CARTESIAN_POINT('Ctrl Pts',(-4.46847307119201,1.21580144485612,3.99646497806116));
#40063=CARTESIAN_POINT('Ctrl Pts',(-4.47120875000575,1.31290853880528,4.));
#40064=CARTESIAN_POINT('Ctrl Pts',(-4.47396821277762,1.41,4.));
#40065=CARTESIAN_POINT('Origin',(-12.6,0.,0.));
#40066=CARTESIAN_POINT('',(-12.5998293715479,4.2015986146261,2.27233586799447));
#40067=CARTESIAN_POINT('Ctrl Pts',(-12.6,-2.05373368417785,2.00041480624693));
#40068=CARTESIAN_POINT('Ctrl Pts',(-12.6,-1.86194821019491,2.29644101354744));
#40069=CARTESIAN_POINT('Ctrl Pts',(-12.6,-1.6337237691026,2.56258505139432));
#40070=CARTESIAN_POINT('Ctrl Pts',(-12.6,-1.11617616238642,3.02636049189356));
#40071=CARTESIAN_POINT('Ctrl Pts',(-12.6,-0.82928342253897,3.22307976599948));
#40072=CARTESIAN_POINT('Ctrl Pts',(-12.6,-0.123052762143918,3.5775029713655));
#40073=CARTESIAN_POINT('Ctrl Pts',(-12.6,0.359088891234675,3.7349719142707));
#40074=CARTESIAN_POINT('Ctrl Pts',(-12.6,1.34810068326337,3.8116791096069));
#40075=CARTESIAN_POINT('Ctrl Pts',(-12.6,1.84369675616155,3.77282245092087));
#40076=CARTESIAN_POINT('Ctrl Pts',(-12.6,2.72178118022736,3.49119653737293));
#40077=CARTESIAN_POINT('Ctrl Pts',(-12.5999999999996,3.07511507231026,3.31288578245549));
#40078=CARTESIAN_POINT('Ctrl Pts',(-12.5999999999996,3.75009162428244,2.82374222223055));
#40079=CARTESIAN_POINT('Ctrl Pts',(-12.6,4.01274809895788,2.53388433006154));
#40080=CARTESIAN_POINT('Ctrl Pts',(-12.6,4.20183229445798,2.27251622505692));
#40081=CARTESIAN_POINT('',(-12.6000166008662,0.83772686667478,-3.55358061870878));
#40082=CARTESIAN_POINT('Ctrl Pts',(-12.6,0.837723077840343,-3.55360908009661));
#40083=CARTESIAN_POINT('Ctrl Pts',(-12.6,0.496521059253182,-3.51949309243697));
#40084=CARTESIAN_POINT('Ctrl Pts',(-12.5999999999999,0.146329052235482,
-3.43525773297163));
#40085=CARTESIAN_POINT('Ctrl Pts',(-12.5999999999999,-0.553018328867865,
-3.134995004088));
#40086=CARTESIAN_POINT('Ctrl Pts',(-12.5999999999999,-0.871307034171167,
-2.93779118035574));
#40087=CARTESIAN_POINT('Ctrl Pts',(-12.5999999999999,-1.53424447284485,
-2.37755905857722));
#40088=CARTESIAN_POINT('Ctrl Pts',(-12.6,-1.83990405226507,-1.98879992581603));
#40089=CARTESIAN_POINT('Ctrl Pts',(-12.6,-2.29324808716915,-1.09713296481856));
#40090=CARTESIAN_POINT('Ctrl Pts',(-12.6000000000002,-2.43367803893011,
-0.602366737831792));
#40091=CARTESIAN_POINT('Ctrl Pts',(-12.6000000000002,-2.50222265717766,
0.237740648443177));
#40092=CARTESIAN_POINT('Ctrl Pts',(-12.6000000000001,-2.48645615185202,
0.59285266331533));
#40093=CARTESIAN_POINT('Ctrl Pts',(-12.6000000000001,-2.33846043510994,
1.32747957975342));
#40094=CARTESIAN_POINT('Ctrl Pts',(-12.6,-2.21733170155652,1.67484059027454));
#40095=CARTESIAN_POINT('Ctrl Pts',(-12.6,-2.05238345558469,1.99966421701685));
#40096=CARTESIAN_POINT('Ctrl Pts',(-12.6,4.20136030793409,2.27216120781755));
#40097=CARTESIAN_POINT('Ctrl Pts',(-12.6,4.24991321932181,2.21237988743208));
#40098=CARTESIAN_POINT('Ctrl Pts',(-12.6,4.29624720254232,2.15145486239861));
#40099=CARTESIAN_POINT('Ctrl Pts',(-12.6,4.34045738936432,2.08940595404779));
#40100=CARTESIAN_POINT('Ctrl Pts',(-12.6,4.3850853028298,2.02677076719239));
#40101=CARTESIAN_POINT('Ctrl Pts',(-12.6,4.42754941898348,1.96298989968627));
#40102=CARTESIAN_POINT('Ctrl Pts',(-12.6,4.4679095774266,1.89804670263138));
#40103=CARTESIAN_POINT('Ctrl Pts',(-12.6,4.50538330437375,1.83774803861745));
#40104=CARTESIAN_POINT('Ctrl Pts',(-12.6,4.54104318206744,1.77644645371704));
#40105=CARTESIAN_POINT('Ctrl Pts',(-12.6,4.57490409351515,1.71410627284305));
#40106=CARTESIAN_POINT('Ctrl Pts',(-12.6,4.63217999330126,1.60865754746247));
#40107=CARTESIAN_POINT('Ctrl Pts',(-12.6,4.68429586644297,1.50024999578326));
#40108=CARTESIAN_POINT('Ctrl Pts',(-12.6,4.73090070615598,1.38925781853925));
#40109=CARTESIAN_POINT('Ctrl Pts',(-12.6,4.76695274428081,1.3033977612963));
#40110=CARTESIAN_POINT('Ctrl Pts',(-12.6,4.79970608847906,1.21599067617616));
#40111=CARTESIAN_POINT('Ctrl Pts',(-12.6,4.82897683811643,1.12720778050039));
#40112=CARTESIAN_POINT('Ctrl Pts',(-12.6,4.85313221137757,1.05394064485055));
#40113=CARTESIAN_POINT('Ctrl Pts',(-12.6,4.87491474427738,0.979727992501767));
#40114=CARTESIAN_POINT('Ctrl Pts',(-12.6,4.8942662152241,0.904841310809496));
#40115=CARTESIAN_POINT('Ctrl Pts',(-12.6,4.91634804391075,0.819388640023172));
#40116=CARTESIAN_POINT('Ctrl Pts',(-12.6,4.93526322302942,0.733059052030427));
#40117=CARTESIAN_POINT('Ctrl Pts',(-12.6,4.95097297319694,0.646271284840811));
#40118=CARTESIAN_POINT('Ctrl Pts',(-12.6,4.96214115241793,0.584573210216633));
#40119=CARTESIAN_POINT('Ctrl Pts',(-12.6,4.97169041730954,0.522643909668857));
#40120=CARTESIAN_POINT('Ctrl Pts',(-12.6,4.97962272537674,0.460635682766227));
#40121=CARTESIAN_POINT('Ctrl Pts',(-12.6,4.99040979052231,0.376311325026525));
#40122=CARTESIAN_POINT('Ctrl Pts',(-12.6,4.99821257200861,0.291844226308379));
#40123=CARTESIAN_POINT('Ctrl Pts',(-12.6,5.00307142381211,0.207270573524764));
#40124=CARTESIAN_POINT('Ctrl Pts',(-12.6,5.00810941634383,0.11957877959151));
#40125=CARTESIAN_POINT('Ctrl Pts',(-12.6,5.00998274524699,0.0317718262261336));
#40126=CARTESIAN_POINT('Ctrl Pts',(-12.6,5.00867893574776,-0.0561151865291535));
#40127=CARTESIAN_POINT('Ctrl Pts',(-12.6,5.00792611094464,-0.106861498097263));
#40128=CARTESIAN_POINT('Ctrl Pts',(-12.6,5.00611296071654,-0.157634547885469));
#40129=CARTESIAN_POINT('Ctrl Pts',(-12.6,5.00322813990553,-0.208426976174122));
#40130=CARTESIAN_POINT('Ctrl Pts',(-12.6,4.99817808622467,-0.297342200461094));
#40131=CARTESIAN_POINT('Ctrl Pts',(-12.6,4.98983826675716,-0.386322571517995));
#40132=CARTESIAN_POINT('Ctrl Pts',(-12.6,4.97817114946835,-0.474964333428603));
#40133=CARTESIAN_POINT('Ctrl Pts',(-12.6,4.96609764893234,-0.566693621259453));
#40134=CARTESIAN_POINT('Ctrl Pts',(-12.6,4.95046069958265,-0.658059603697444));
#40135=CARTESIAN_POINT('Ctrl Pts',(-12.6,4.93126873595277,-0.748617385727737));
#40136=CARTESIAN_POINT('Ctrl Pts',(-12.6,4.92455646675259,-0.780289403395168));
#40137=CARTESIAN_POINT('Ctrl Pts',(-12.6,4.91740980403444,-0.811862632160295));
#40138=CARTESIAN_POINT('Ctrl Pts',(-12.6,4.9098305906043,-0.843318348590614));
#40139=CARTESIAN_POINT('Ctrl Pts',(-12.6,4.89642338914026,-0.898961738404567));
#40140=CARTESIAN_POINT('Ctrl Pts',(-12.6,4.8816647095724,-0.95423026124531));
#40141=CARTESIAN_POINT('Ctrl Pts',(-12.6,4.86559189236515,-1.00907338768238));
#40142=CARTESIAN_POINT('Ctrl Pts',(-12.6,4.83077712152216,-1.12786717812997));
#40143=CARTESIAN_POINT('Ctrl Pts',(-12.6,4.78979779688126,-1.24467503826931));
#40144=CARTESIAN_POINT('Ctrl Pts',(-12.6,4.74297831680097,-1.35904511124462));
#40145=CARTESIAN_POINT('Ctrl Pts',(-12.6,4.69520358782485,-1.47574865494059));
#40146=CARTESIAN_POINT('Ctrl Pts',(-12.6,4.64134719657638,-1.58991571958614));
#40147=CARTESIAN_POINT('Ctrl Pts',(-12.6,4.58170281408354,-1.70104801874762));
#40148=CARTESIAN_POINT('Ctrl Pts',(-12.6,4.53894557569914,-1.78071537397632));
#40149=CARTESIAN_POINT('Ctrl Pts',(-12.6,4.49321317213389,-1.85882199777155));
#40150=CARTESIAN_POINT('Ctrl Pts',(-12.6,4.44460131475763,-1.9351736094758));
#40151=CARTESIAN_POINT('Ctrl Pts',(-12.6,4.40703843688988,-1.99417127836253));
#40152=CARTESIAN_POINT('Ctrl Pts',(-12.6,4.36775615962475,-2.05212081170236));
#40153=CARTESIAN_POINT('Ctrl Pts',(-12.6,4.32679409915763,-2.10892946550827));
#40154=CARTESIAN_POINT('Ctrl Pts',(-12.6,4.26552386323019,-2.19390272080146));
#40155=CARTESIAN_POINT('Ctrl Pts',(-12.6,4.20049767569927,-2.27631129829982));
#40156=CARTESIAN_POINT('Ctrl Pts',(-12.6,4.13199412674128,-2.35567648544826));
#40157=CARTESIAN_POINT('Ctrl Pts',(-12.6,4.07080391109937,-2.42656876752625));
#40158=CARTESIAN_POINT('Ctrl Pts',(-12.6,4.00683995756574,-2.49503280234516));
#40159=CARTESIAN_POINT('Ctrl Pts',(-12.6,3.94032724264284,-2.5607506800043));
#40160=CARTESIAN_POINT('Ctrl Pts',(-12.6,3.90748575173575,-2.5931997099992));
#40161=CARTESIAN_POINT('Ctrl Pts',(-12.6,3.87402616911567,-2.62497698489842));
#40162=CARTESIAN_POINT('Ctrl Pts',(-12.6,3.83998007956055,-2.65606989143867));
#40163=CARTESIAN_POINT('Ctrl Pts',(-12.6,3.75997804822116,-2.72913248734819));
#40164=CARTESIAN_POINT('Ctrl Pts',(-12.6,3.67673002715616,-2.79842887040651));
#40165=CARTESIAN_POINT('Ctrl Pts',(-12.6,3.59053368325527,-2.86385313140299));
#40166=CARTESIAN_POINT('Ctrl Pts',(-12.6,3.53048820079388,-2.90942851358777));
#40167=CARTESIAN_POINT('Ctrl Pts',(-12.6,3.4690111015832,-2.95312415191365));
#40168=CARTESIAN_POINT('Ctrl Pts',(-12.6,3.40619362993573,-2.9948927862738));
#40169=CARTESIAN_POINT('Ctrl Pts',(-12.6,3.33281523122669,-3.04368359916757));
#40170=CARTESIAN_POINT('Ctrl Pts',(-12.6,3.25759896657405,-3.08984861095697));
#40171=CARTESIAN_POINT('Ctrl Pts',(-12.6,3.18077002699366,-3.13324970066485));
#40172=CARTESIAN_POINT('Ctrl Pts',(-12.6,3.07483187106991,-3.193094746475));
#40173=CARTESIAN_POINT('Ctrl Pts',(-12.6,2.96582853574357,-3.24768272390825));
#40174=CARTESIAN_POINT('Ctrl Pts',(-12.6,2.85437152516411,-3.29666597621036));
#40175=CARTESIAN_POINT('Ctrl Pts',(-12.6,2.76538543218785,-3.33577368438387));
#40176=CARTESIAN_POINT('Ctrl Pts',(-12.6,2.6748342422647,-3.37131051831734));
#40177=CARTESIAN_POINT('Ctrl Pts',(-12.6,2.58301134616202,-3.40311631283128));
#40178=CARTESIAN_POINT('Ctrl Pts',(-12.6,2.46115060033201,-3.44532667653894));
#40179=CARTESIAN_POINT('Ctrl Pts',(-12.6,2.33705407145644,-3.48096305732652));
#40180=CARTESIAN_POINT('Ctrl Pts',(-12.6,2.2114307992263,-3.50965933874659));
#40181=CARTESIAN_POINT('Ctrl Pts',(-12.6,2.11981415277956,-3.53058744404528));
#40182=CARTESIAN_POINT('Ctrl Pts',(-12.6,2.02738809550088,-3.5478233034159));
#40183=CARTESIAN_POINT('Ctrl Pts',(-12.6,1.93449359128411,-3.56138533330371));
#40184=CARTESIAN_POINT('Ctrl Pts',(-12.6,1.84382361703015,-3.57462259541225));
#40185=CARTESIAN_POINT('Ctrl Pts',(-12.6,1.75270509672104,-3.58436050971007));
#40186=CARTESIAN_POINT('Ctrl Pts',(-12.6,1.66144632445628,-3.59062972534713));
#40187=CARTESIAN_POINT('Ctrl Pts',(-12.6,1.61183505842739,-3.59403787688198));
#40188=CARTESIAN_POINT('Ctrl Pts',(-12.6,1.56218231482985,-3.59642109941458));
#40189=CARTESIAN_POINT('Ctrl Pts',(-12.6,1.51253728145747,-3.59778572530998));
#40190=CARTESIAN_POINT('Ctrl Pts',(-12.6,1.44328272851095,-3.59968937105066));
#40191=CARTESIAN_POINT('Ctrl Pts',(-12.6,1.37405002548623,-3.59961389113362));
#40192=CARTESIAN_POINT('Ctrl Pts',(-12.6,1.30479205521246,-3.59756529266946));
#40193=CARTESIAN_POINT('Ctrl Pts',(-12.6,1.22725669285759,-3.59527185519777));
#40194=CARTESIAN_POINT('Ctrl Pts',(-12.6,1.14968867032937,-3.59050647284628));
#40195=CARTESIAN_POINT('Ctrl Pts',(-12.6,1.07202485443785,-3.58322209629984));
#40196=CARTESIAN_POINT('Ctrl Pts',(-12.6,0.994361038546337,-3.57593771975341));
#40197=CARTESIAN_POINT('Ctrl Pts',(-12.6,0.916600758134591,-3.56613439828602));
#40198=CARTESIAN_POINT('Ctrl Pts',(-12.6,0.838694895738728,-3.55370611520755));
#40199=CARTESIAN_POINT('Ctrl Pts',(-12.87044835945,4.833816836034,2.150398813705));
#40200=CARTESIAN_POINT('Ctrl Pts',(-12.85461132379,4.548510437562,2.604657272318));
#40201=CARTESIAN_POINT('Ctrl Pts',(-12.82293725246,3.794830979319,3.397883596158));
#40202=CARTESIAN_POINT('Ctrl Pts',(-12.77542614546,2.291343487621,4.056653234419));
#40203=CARTESIAN_POINT('Ctrl Pts',(-12.72791503846,0.6500910845242,4.081135185525));
#40204=CARTESIAN_POINT('Ctrl Pts',(-12.68040393146,-0.8723606288515,3.467561272573));
#40205=CARTESIAN_POINT('Ctrl Pts',(-12.63289282446,-2.037972680177,2.31184527703));
#40206=CARTESIAN_POINT('Ctrl Pts',(-12.58538171746,-2.664509177573,0.7946828350227));
#40207=CARTESIAN_POINT('Ctrl Pts',(-12.53787061046,-2.654013040306,-0.8467251880981));
#40208=CARTESIAN_POINT('Ctrl Pts',(-12.49035950346,-2.008125483935,-2.355751205884));
#40209=CARTESIAN_POINT('Ctrl Pts',(-12.44284839646,-0.827828292971,-3.496465367642));
#40210=CARTESIAN_POINT('Ctrl Pts',(-12.39533728947,0.7023440434848,-4.090521836345));
#40211=CARTESIAN_POINT('Ctrl Pts',(-12.34782618247,2.343155260531,-4.045042082342));
#40212=CARTESIAN_POINT('Ctrl Pts',(-12.30031507547,3.838072193312,-3.367137752342));
#40213=CARTESIAN_POINT('Ctrl Pts',(-12.25280396847,4.953367790708,-2.162792329864));
#40214=CARTESIAN_POINT('Ctrl Pts',(-12.20529286147,5.51468157619,-0.6203152146922));
#40215=CARTESIAN_POINT('Ctrl Pts',(-12.15778175447,5.434212202017,1.019189818483));
#40216=CARTESIAN_POINT('Ctrl Pts',(-12.12610768314,4.961203081187,2.005852424555));
#40217=CARTESIAN_POINT('Ctrl Pts',(-12.11027064747,4.638247898493,2.434163571038));
#40218=CARTESIAN_POINT('Ctrl Pts',(-12.77687535715,4.696568786966,2.0641973444));
#40219=CARTESIAN_POINT('Ctrl Pts',(-12.76103832148,4.422699258062,2.5002462754));
#40220=CARTESIAN_POINT('Ctrl Pts',(-12.72936425015,3.699231998725,3.261675113968));
#40221=CARTESIAN_POINT('Ctrl Pts',(-12.68185314315,2.256013713854,3.894037134075));
#40222=CARTESIAN_POINT('Ctrl Pts',(-12.63434203615,0.6805529991396,3.917537695058));
#40223=CARTESIAN_POINT('Ctrl Pts',(-12.58683092915,-0.780869302481,3.328559672174));
#40224=CARTESIAN_POINT('Ctrl Pts',(-12.53931982215,-1.899756313399,2.219172021067));
#40225=CARTESIAN_POINT('Ctrl Pts',(-12.49180871515,-2.501177299056,0.7628269636494));
#40226=CARTESIAN_POINT('Ctrl Pts',(-12.44429760815,-2.49110191279,-0.8127831328632));
#40227=CARTESIAN_POINT('Ctrl Pts',(-12.39678650115,-1.871105579949,-2.261317924964));
#40228=CARTESIAN_POINT('Ctrl Pts',(-12.34927539416,-0.7381221018787,-3.356305109859));
#40229=CARTESIAN_POINT('Ctrl Pts',(-12.30176428716,0.730711331834,-3.926548070051));
#40230=CARTESIAN_POINT('Ctrl Pts',(-12.25425318016,2.305748546002,-3.882891429786));
#40231=CARTESIAN_POINT('Ctrl Pts',(-12.20674207316,3.740739833701,-3.232161756375));
#40232=CARTESIAN_POINT('Ctrl Pts',(-12.15923096616,4.81132738969,-2.076094050713));
#40233=CARTESIAN_POINT('Ctrl Pts',(-12.11171985916,5.350140198729,-0.5954490909769));
#40234=CARTESIAN_POINT('Ctrl Pts',(-12.06420875216,5.272896541685,0.9783342993609));
#40235=CARTESIAN_POINT('Ctrl Pts',(-12.03253468083,4.818848592592,1.925445280958));
#40236=CARTESIAN_POINT('Ctrl Pts',(-12.01669764516,4.508839478827,2.33658703081));
#40237=CARTESIAN_POINT('Ctrl Pts',(-12.68330235484,4.559320737899,1.977995875095));
#40238=CARTESIAN_POINT('Ctrl Pts',(-12.66746531917,4.296888078562,2.395835278482));
#40239=CARTESIAN_POINT('Ctrl Pts',(-12.63579124784,3.60363301813,3.125466631779));
#40240=CARTESIAN_POINT('Ctrl Pts',(-12.58828014084,2.220683940088,3.731421033731));
#40241=CARTESIAN_POINT('Ctrl Pts',(-12.54076903384,0.711014913755,3.753940204591));
#40242=CARTESIAN_POINT('Ctrl Pts',(-12.49325792684,-0.6893779761106,3.189558071774));
#40243=CARTESIAN_POINT('Ctrl Pts',(-12.44574681984,-1.76153994662,2.126498765103));
#40244=CARTESIAN_POINT('Ctrl Pts',(-12.39823571284,-2.337845420538,0.7309710922762));
#40245=CARTESIAN_POINT('Ctrl Pts',(-12.35072460584,-2.328190785274,-0.7788410776284));
#40246=CARTESIAN_POINT('Ctrl Pts',(-12.30321349885,-1.734085675964,-2.166884644044));
#40247=CARTESIAN_POINT('Ctrl Pts',(-12.25570239185,-0.6484159107864,-3.216144852076));
#40248=CARTESIAN_POINT('Ctrl Pts',(-12.20819128485,0.7590786201833,-3.762574303757));
#40249=CARTESIAN_POINT('Ctrl Pts',(-12.16068017785,2.268341831473,-3.720740777229));
#40250=CARTESIAN_POINT('Ctrl Pts',(-12.11316907085,3.64340747409,-3.097185760409));
#40251=CARTESIAN_POINT('Ctrl Pts',(-12.06565796385,4.669286988672,-1.989395771562));
#40252=CARTESIAN_POINT('Ctrl Pts',(-12.01814685685,5.185598821268,-0.5705829672616));
#40253=CARTESIAN_POINT('Ctrl Pts',(-11.97063574985,5.111580881353,0.9374787802385));
#40254=CARTESIAN_POINT('Ctrl Pts',(-11.93896167852,4.676494103997,1.84503813736));
#40255=CARTESIAN_POINT('Ctrl Pts',(-11.92312464285,4.379431059162,2.239010490582));
#40256=CARTESIAN_POINT('Ctrl Pts',(-12.58972935253,4.422072688831,1.89179440579));
#40257=CARTESIAN_POINT('Ctrl Pts',(-12.57389231686,4.171076899062,2.291424281564));
#40258=CARTESIAN_POINT('Ctrl Pts',(-12.54221824553,3.508034037536,2.98925814959));
#40259=CARTESIAN_POINT('Ctrl Pts',(-12.49470713853,2.185354166322,3.568804933387));
#40260=CARTESIAN_POINT('Ctrl Pts',(-12.44719603153,0.7414768283704,3.590342714124));
#40261=CARTESIAN_POINT('Ctrl Pts',(-12.39968492453,-0.5978866497401,3.050556471375));
#40262=CARTESIAN_POINT('Ctrl Pts',(-12.35217381753,-1.623323579841,2.03382550914));
#40263=CARTESIAN_POINT('Ctrl Pts',(-12.30466271053,-2.174513542021,0.699115220903));
#40264=CARTESIAN_POINT('Ctrl Pts',(-12.25715160354,-2.165279657758,-0.7448990223935));
#40265=CARTESIAN_POINT('Ctrl Pts',(-12.20964049654,-1.597065771978,-2.072451363124));
#40266=CARTESIAN_POINT('Ctrl Pts',(-12.16212938954,-0.5587097196941,-3.075984594292));
#40267=CARTESIAN_POINT('Ctrl Pts',(-12.11461828254,0.7874459085325,-3.598600537463));
#40268=CARTESIAN_POINT('Ctrl Pts',(-12.06710717554,2.230935116944,-3.558590124673));
#40269=CARTESIAN_POINT('Ctrl Pts',(-12.01959606854,3.546075114479,-2.962209764442));
#40270=CARTESIAN_POINT('Ctrl Pts',(-11.97208496154,4.527246587654,-1.902697492411));
#40271=CARTESIAN_POINT('Ctrl Pts',(-11.92457385454,5.021057443807,-0.5457168435463));
#40272=CARTESIAN_POINT('Ctrl Pts',(-11.87706274754,4.950265221021,0.8966232611161));
#40273=CARTESIAN_POINT('Ctrl Pts',(-11.84538867621,4.534139615403,1.764630993762));
#40274=CARTESIAN_POINT('Ctrl Pts',(-11.82955164055,4.250022639497,2.141433950353));
#40275=CARTESIAN_POINT('',(-11.868972894178,4.52769007505164,1.79999920916443));
#40276=CARTESIAN_POINT('Ctrl Pts',(-12.5996587430957,4.20136493479422,2.27215551093202));
#40277=CARTESIAN_POINT('Ctrl Pts',(-12.5943977786613,4.09860310341828,2.39868269823106));
#40278=CARTESIAN_POINT('Ctrl Pts',(-12.5891758755894,3.98732502091615,2.51830284549381));
#40279=CARTESIAN_POINT('Ctrl Pts',(-12.5785334644535,3.75015247715258,2.74049997081469));
#40280=CARTESIAN_POINT('Ctrl Pts',(-12.5730829185006,3.62515140958853,2.84237580960055));
#40281=CARTESIAN_POINT('Ctrl Pts',(-12.556572201564,3.22841147029478,3.12311372977992));
#40282=CARTESIAN_POINT('Ctrl Pts',(-12.5457361202519,2.93796003113066,3.27451147511612));
#40283=CARTESIAN_POINT('Ctrl Pts',(-12.5280760942906,2.43253160915354,3.45764998533339));
#40284=CARTESIAN_POINT('Ctrl Pts',(-12.5211823286344,2.22577086567203,3.51265613920689));
#40285=CARTESIAN_POINT('Ctrl Pts',(-12.4992511023973,1.56189787140324,3.62639865061708));
#40286=CARTESIAN_POINT('Ctrl Pts',(-12.484922380463,1.15006165872664,3.60587160724037));
#40287=CARTESIAN_POINT('Ctrl Pts',(-12.4639364419627,0.523509741436324,
3.50053912987217));
#40288=CARTESIAN_POINT('Ctrl Pts',(-12.4548990117254,0.241048622196361,
3.41743552208491));
#40289=CARTESIAN_POINT('Ctrl Pts',(-12.4375181030687,-0.238498909654585,
3.20870288645154));
#40290=CARTESIAN_POINT('Ctrl Pts',(-12.4294229188578,-0.440818259230192,
3.09578061643052));
#40291=CARTESIAN_POINT('Ctrl Pts',(-12.4071928908363,-0.984372392936457,
2.72079031597198));
#40292=CARTESIAN_POINT('Ctrl Pts',(-12.3928585057436,-1.31725659785877,
2.39882366289928));
#40293=CARTESIAN_POINT('Ctrl Pts',(-12.3611843204163,-1.84416734655621,
1.60897918648557));
#40294=CARTESIAN_POINT('Ctrl Pts',(-12.3450246572973,-2.02638844346352,
1.1670536115216));
#40295=CARTESIAN_POINT('Ctrl Pts',(-12.3261340790523,-2.14180721490078,
0.595506606229493));
#40296=CARTESIAN_POINT('Ctrl Pts',(-12.3224922447298,-2.15912086449384,
0.482401799479392));
#40297=CARTESIAN_POINT('Ctrl Pts',(-12.3029528758476,-2.2218564421081,-0.120504474255441));
#40298=CARTESIAN_POINT('Ctrl Pts',(-12.2886922857574,-2.1616248015831,-0.521999727125013));
#40299=CARTESIAN_POINT('Ctrl Pts',(-12.2682288883678,-2.02587956750989,
-1.12474793886592));
#40300=CARTESIAN_POINT('Ctrl Pts',(-12.2575770430017,-1.9034310571764,-1.44871120196594));
#40301=CARTESIAN_POINT('Ctrl Pts',(-12.2422350361894,-1.68078614497929,
-1.84942730753048));
#40302=CARTESIAN_POINT('Ctrl Pts',(-12.2382762535475,-1.61966717685923,
-1.94766303165829));
#40303=CARTESIAN_POINT('Ctrl Pts',(-12.218472214655,-1.28838939160236,-2.42686360279675));
#40304=CARTESIAN_POINT('Ctrl Pts',(-12.2031328728078,-0.947551774547012,
-2.75945540978527));
#40305=CARTESIAN_POINT('Ctrl Pts',(-12.180436080769,-0.363277372009374,
-3.14160848430859));
#40306=CARTESIAN_POINT('Ctrl Pts',(-12.1728536629882,-0.159300414696784,
-3.24797575371841));
#40307=CARTESIAN_POINT('Ctrl Pts',(-12.1571553863382,0.26932015198446,-3.42157278122556));
#40308=CARTESIAN_POINT('Ctrl Pts',(-12.14918351821,0.493308904608057,-3.48800886339262));
#40309=CARTESIAN_POINT('Ctrl Pts',(-12.1275974487476,1.13532477107718,-3.61349967260649));
#40310=CARTESIAN_POINT('Ctrl Pts',(-12.1148683059215,1.54872569242995,-3.62168563678726));
#40311=CARTESIAN_POINT('Ctrl Pts',(-12.0846045416093,2.42015504579482,-3.48538716709611));
#40312=CARTESIAN_POINT('Ctrl Pts',(-12.0696896115077,2.86579441032513,-3.32442554417545));
#40313=CARTESIAN_POINT('Ctrl Pts',(-12.0352911704397,3.76528393057223,-2.78522738984507));
#40314=CARTESIAN_POINT('Ctrl Pts',(-12.0189478704682,4.08895246372873,-2.42514526884088));
#40315=CARTESIAN_POINT('Ctrl Pts',(-12.0003638630839,4.42709248004169,-1.97674525807511));
#40316=CARTESIAN_POINT('Ctrl Pts',(-11.9928408103346,4.55088803313591,-1.77452838689738));
#40317=CARTESIAN_POINT('Ctrl Pts',(-11.9685369634296,4.87639280789863,-1.099887590332));
#40318=CARTESIAN_POINT('Ctrl Pts',(-11.9522024910297,4.97231142635138,-0.644603860682317));
#40319=CARTESIAN_POINT('Ctrl Pts',(-11.9337752540346,5.01281190989049,-0.0762115415695516));
#40320=CARTESIAN_POINT('Ctrl Pts',(-11.9281519807879,5.01253713121989,0.101078384455938));
#40321=CARTESIAN_POINT('Ctrl Pts',(-11.9136267266903,4.97870465316466,0.546027495964662));
#40322=CARTESIAN_POINT('Ctrl Pts',(-11.904380454833,4.92766437497361,0.809675408134278));
#40323=CARTESIAN_POINT('Ctrl Pts',(-11.8863722838056,4.76870972989004,1.32058258936207));
#40324=CARTESIAN_POINT('Ctrl Pts',(-11.8775396760734,4.66075207090338,1.5675594124826));
#40325=CARTESIAN_POINT('Ctrl Pts',(-11.8687770177641,4.52712046807184,1.79966253176968));
#40326=CARTESIAN_POINT('',(-12.099082574484,4.87271762261516,1.99920743468592));
#40327=CARTESIAN_POINT('',(-12.1,4.874101615138,2.));
#40328=CARTESIAN_POINT('',(-12.1620549971849,5.40898507946903,-1.21540908076623E-5));
#40329=CARTESIAN_POINT('Ctrl Pts',(-12.1620549971849,5.40898507946903,-1.21540908101445E-5));
#40330=CARTESIAN_POINT('Ctrl Pts',(-12.1569738930589,5.40917196074869,0.174930914237154));
#40331=CARTESIAN_POINT('Ctrl Pts',(-12.1519119116125,5.3979768036158,0.349893835687258));
#40332=CARTESIAN_POINT('Ctrl Pts',(-12.1416589980365,5.35271339118928,0.696450564633029));
#40333=CARTESIAN_POINT('Ctrl Pts',(-12.1364520209065,5.31874370082235,0.867680261306424));
#40334=CARTESIAN_POINT('Ctrl Pts',(-12.120579344798,5.18256318174135,1.37317087302075));
#40335=CARTESIAN_POINT('Ctrl Pts',(-12.1098370351016,5.04719145687279,1.69755110551158));
#40336=CARTESIAN_POINT('Ctrl Pts',(-12.0993394760039,4.87295253544702,1.99931610218236));
#40337=CARTESIAN_POINT('',(-12.5375049769753,-2.58973741874834,-1.59154708263292E-8));
#40338=CARTESIAN_POINT('Ctrl Pts',(-12.5375049769753,-2.58973741874834,
-1.59154705386966E-8));
#40339=CARTESIAN_POINT('Ctrl Pts',(-12.5229809386071,-2.58925208028242,
-0.477750600220128));
#40340=CARTESIAN_POINT('Ctrl Pts',(-12.5081812696076,-2.50269412720891,
-0.95241726371786));
#40341=CARTESIAN_POINT('Ctrl Pts',(-12.4828898262183,-2.20080335467406,
-1.76103220854594));
#40342=CARTESIAN_POINT('Ctrl Pts',(-12.4678568782273,-1.96397912807987,
-2.2454221394074));
#40343=CARTESIAN_POINT('Ctrl Pts',(-12.4378211477566,-1.29369923449151,
-2.96535211887595));
#40344=CARTESIAN_POINT('Ctrl Pts',(-12.4274807844472,-1.0352545554023,-3.18146576343454));
#40345=CARTESIAN_POINT('Ctrl Pts',(-12.4099857148573,-0.539434250315809,
-3.50087276770335));
#40346=CARTESIAN_POINT('Ctrl Pts',(-12.4026593404811,-0.311416064037279,
-3.61872249168621));
#40347=CARTESIAN_POINT('Ctrl Pts',(-12.378286903758,0.467325590917832,-3.93113010406675));
#40348=CARTESIAN_POINT('Ctrl Pts',(-12.3623752784994,0.981654375399767,
-4.00030241540116));
#40349=CARTESIAN_POINT('Ctrl Pts',(-12.3410980017126,1.68519871182383,-3.99775483161553));
#40350=CARTESIAN_POINT('Ctrl Pts',(-12.3332033087745,1.94933834976081,-3.9709602694738));
#40351=CARTESIAN_POINT('Ctrl Pts',(-12.3180516147445,2.45704356521002,-3.8682399238872));
#40352=CARTESIAN_POINT('Ctrl Pts',(-12.3108611512601,2.70001301347965,-3.79447138319196));
#40353=CARTESIAN_POINT('Ctrl Pts',(-12.2944726507626,3.21386326258636,-3.58290739661591));
#40354=CARTESIAN_POINT('Ctrl Pts',(-12.2850438758018,3.47926772047201,-3.43580922523939));
#40355=CARTESIAN_POINT('Ctrl Pts',(-12.2597967792659,4.15128057484633,-2.95764610397139));
#40356=CARTESIAN_POINT('Ctrl Pts',(-12.2445865801277,4.5179805244572,-2.57036434011953));
#40357=CARTESIAN_POINT('Ctrl Pts',(-12.2185641240652,4.99311961089714,-1.81620680963327));
#40358=CARTESIAN_POINT('Ctrl Pts',(-12.2075070265642,5.1435641225043,-1.47995601386522));
#40359=CARTESIAN_POINT('Ctrl Pts',(-12.1845278121184,5.35388368311229,-0.762341942254753));
#40360=CARTESIAN_POINT('Ctrl Pts',(-12.1731517423075,5.40857694496182,-0.382074515354316));
#40361=CARTESIAN_POINT('Ctrl Pts',(-12.1620549971849,5.40898507946903,-1.2154090805426E-5));
#40362=CARTESIAN_POINT('Ctrl Pts',(-12.5995521747198,-2.05308781517742,
1.9999870693724));
#40363=CARTESIAN_POINT('Ctrl Pts',(-12.5888604919629,-2.22886541883401,
1.69465508600805));
#40364=CARTESIAN_POINT('Ctrl Pts',(-12.5783563691698,-2.36455856972317,
1.36606660230804));
#40365=CARTESIAN_POINT('Ctrl Pts',(-12.5578742591034,-2.54469535699154,
0.691070574695697));
#40366=CARTESIAN_POINT('Ctrl Pts',(-12.5480600623093,-2.59009012980526,
0.347196683644455));
#40367=CARTESIAN_POINT('Ctrl Pts',(-12.5375049769753,-2.58973741874834,
-1.59154708263292E-8));
#40368=CARTESIAN_POINT('Ctrl Pts',(-12.8808295573,-1.233284553369,2.380024102084));
#40369=CARTESIAN_POINT('Ctrl Pts',(-12.85374622397,-1.773294892526,1.78028186128));
#40370=CARTESIAN_POINT('Ctrl Pts',(-12.7995795573,-2.426733796392,0.2014420016719));
#40371=CARTESIAN_POINT('Ctrl Pts',(-12.7183295573,-1.698583059424,-2.258550295837));
#40372=CARTESIAN_POINT('Ctrl Pts',(-12.6370795573,0.4155582784152,-3.711366470425));
#40373=CARTESIAN_POINT('Ctrl Pts',(-12.5558295573,2.972804381698,-3.510136505478));
#40374=CARTESIAN_POINT('Ctrl Pts',(-12.4745795573,4.833529694393,-1.744372868486));
#40375=CARTESIAN_POINT('Ctrl Pts',(-12.3933295573,5.168351131249,0.7988617992865));
#40376=CARTESIAN_POINT('Ctrl Pts',(-12.3120795573,3.828047522757,2.986040015375));
#40377=CARTESIAN_POINT('Ctrl Pts',(-12.2308295573,1.41,3.842315305328));
#40378=CARTESIAN_POINT('Ctrl Pts',(-12.1495795573,-1.008047522757,2.986040015375));
#40379=CARTESIAN_POINT('Ctrl Pts',(-12.0683295573,-2.348351131249,0.7988617992864));
#40380=CARTESIAN_POINT('Ctrl Pts',(-11.9870795573,-2.013529694393,-1.744372868486));
#40381=CARTESIAN_POINT('Ctrl Pts',(-11.9058295573,-0.1528043816976,-3.510136505478));
#40382=CARTESIAN_POINT('Ctrl Pts',(-11.8245795573,2.404441721585,-3.711366470425));
#40383=CARTESIAN_POINT('Ctrl Pts',(-11.7433295573,4.518583059424,-2.258550295837));
#40384=CARTESIAN_POINT('Ctrl Pts',(-11.6620795573,5.246733796392,0.2014420016719));
#40385=CARTESIAN_POINT('Ctrl Pts',(-11.60791289063,4.593294892526,1.78028186128));
#40386=CARTESIAN_POINT('Ctrl Pts',(-11.5808295573,4.053284553369,2.380024102084));
#40387=CARTESIAN_POINT('Ctrl Pts',(-12.78725655499,-1.353728408999,2.488472236804));
#40388=CARTESIAN_POINT('Ctrl Pts',(-12.76017322166,-1.918344849396,1.86140215202));
#40389=CARTESIAN_POINT('Ctrl Pts',(-12.70600655499,-2.601558338409,0.210620904237));
#40390=CARTESIAN_POINT('Ctrl Pts',(-12.62475655499,-1.840228698273,-2.361463357323));
#40391=CARTESIAN_POINT('Ctrl Pts',(-12.54350655499,0.3702455651116,-3.880478527159));
#40392=CARTESIAN_POINT('Ctrl Pts',(-12.46225655499,3.04401509758,-3.670079321308));
#40393=CARTESIAN_POINT('Ctrl Pts',(-12.38100655499,4.989526185852,-1.823856930718));
#40394=CARTESIAN_POINT('Ctrl Pts',(-12.29975655499,5.339604090179,0.8352627214266));
#40395=CARTESIAN_POINT('Ctrl Pts',(-12.21850655499,3.938228231968,3.12210186012));
#40396=CARTESIAN_POINT('Ctrl Pts',(-12.13725655499,1.41,4.017394174279));
#40397=CARTESIAN_POINT('Ctrl Pts',(-12.05600655499,-1.118228231968,3.12210186012));
#40398=CARTESIAN_POINT('Ctrl Pts',(-11.97475655499,-2.519604090179,0.8352627214266));
#40399=CARTESIAN_POINT('Ctrl Pts',(-11.89350655499,-2.169526185852,-1.823856930718));
#40400=CARTESIAN_POINT('Ctrl Pts',(-11.81225655499,-0.2240150975802,-3.670079321308));
#40401=CARTESIAN_POINT('Ctrl Pts',(-11.73100655499,2.449754434888,-3.880478527159));
#40402=CARTESIAN_POINT('Ctrl Pts',(-11.64975655499,4.660228698273,-2.361463357323));
#40403=CARTESIAN_POINT('Ctrl Pts',(-11.56850655499,5.421558338409,0.210620904237));
#40404=CARTESIAN_POINT('Ctrl Pts',(-11.51433988833,4.738344849396,1.86140215202));
#40405=CARTESIAN_POINT('Ctrl Pts',(-11.48725655499,4.173728408999,2.488472236804));
#40406=CARTESIAN_POINT('Ctrl Pts',(-12.69368355268,-1.474172264629,2.596920371524));
#40407=CARTESIAN_POINT('Ctrl Pts',(-12.66660021935,-2.063394806267,1.942522442761));
#40408=CARTESIAN_POINT('Ctrl Pts',(-12.61243355268,-2.776382880425,0.219799806802));
#40409=CARTESIAN_POINT('Ctrl Pts',(-12.53118355268,-1.981874337123,-2.464376418808));
#40410=CARTESIAN_POINT('Ctrl Pts',(-12.44993355268,0.3249328518079,-4.049590583892));
#40411=CARTESIAN_POINT('Ctrl Pts',(-12.36868355268,3.115225813463,-3.830022137138));
#40412=CARTESIAN_POINT('Ctrl Pts',(-12.28743355268,5.145522677312,-1.90334099295));
#40413=CARTESIAN_POINT('Ctrl Pts',(-12.20618355268,5.510857049109,0.8716636435667));
#40414=CARTESIAN_POINT('Ctrl Pts',(-12.12493355268,4.048408941179,3.258163704864));
#40415=CARTESIAN_POINT('Ctrl Pts',(-12.04368355268,1.41,4.192473043229));
#40416=CARTESIAN_POINT('Ctrl Pts',(-11.96243355268,-1.228408941179,3.258163704864));
#40417=CARTESIAN_POINT('Ctrl Pts',(-11.88118355268,-2.690857049109,0.8716636435667));
#40418=CARTESIAN_POINT('Ctrl Pts',(-11.79993355268,-2.325522677312,-1.90334099295));
#40419=CARTESIAN_POINT('Ctrl Pts',(-11.71868355268,-0.2952258134628,-3.830022137138));
#40420=CARTESIAN_POINT('Ctrl Pts',(-11.63743355268,2.495067148192,-4.049590583892));
#40421=CARTESIAN_POINT('Ctrl Pts',(-11.55618355268,4.801874337123,-2.464376418808));
#40422=CARTESIAN_POINT('Ctrl Pts',(-11.47493355268,5.596382880425,0.2197998068021));
#40423=CARTESIAN_POINT('Ctrl Pts',(-11.42076688602,4.883394806267,1.942522442761));
#40424=CARTESIAN_POINT('Ctrl Pts',(-11.39368355268,4.294172264629,2.596920371524));
#40425=CARTESIAN_POINT('Ctrl Pts',(-12.60011055037,-1.594616120259,2.705368506244));
#40426=CARTESIAN_POINT('Ctrl Pts',(-12.57302721704,-2.208444763137,2.023642733502));
#40427=CARTESIAN_POINT('Ctrl Pts',(-12.51886055037,-2.951207422442,0.2289787093671));
#40428=CARTESIAN_POINT('Ctrl Pts',(-12.43761055037,-2.123519975972,-2.567289480294));
#40429=CARTESIAN_POINT('Ctrl Pts',(-12.35636055037,0.2796201385043,-4.218702640626));
#40430=CARTESIAN_POINT('Ctrl Pts',(-12.27511055037,3.186436529345,-3.989964952968));
#40431=CARTESIAN_POINT('Ctrl Pts',(-12.19386055037,5.301519168772,-1.982825055182));
#40432=CARTESIAN_POINT('Ctrl Pts',(-12.11261055037,5.682110008039,0.9080645657069));
#40433=CARTESIAN_POINT('Ctrl Pts',(-12.03136055037,4.15858965039,3.394225549609));
#40434=CARTESIAN_POINT('Ctrl Pts',(-11.95011055037,1.41,4.36755191218));
#40435=CARTESIAN_POINT('Ctrl Pts',(-11.86886055037,-1.33858965039,3.394225549609));
#40436=CARTESIAN_POINT('Ctrl Pts',(-11.78761055037,-2.862110008039,0.9080645657069));
#40437=CARTESIAN_POINT('Ctrl Pts',(-11.70636055037,-2.481519168772,-1.982825055182));
#40438=CARTESIAN_POINT('Ctrl Pts',(-11.62511055037,-0.3664365293454,-3.989964952968));
#40439=CARTESIAN_POINT('Ctrl Pts',(-11.54386055037,2.540379861496,-4.218702640626));
#40440=CARTESIAN_POINT('Ctrl Pts',(-11.46261055037,4.943519975972,-2.567289480294));
#40441=CARTESIAN_POINT('Ctrl Pts',(-11.38136055037,5.771207422442,0.2289787093671));
#40442=CARTESIAN_POINT('Ctrl Pts',(-11.32719388371,5.028444763137,2.023642733502));
#40443=CARTESIAN_POINT('Ctrl Pts',(-11.30011055037,4.414616120259,2.705368506244));
#40444=CARTESIAN_POINT('',(-11.7876832506661,-2.5878486596569,-5.29887179826593E-6));
#40445=CARTESIAN_POINT('Ctrl Pts',(-12.0998894289566,4.87211890517844,1.99885431481197));
#40446=CARTESIAN_POINT('Ctrl Pts',(-12.0937922082008,4.77211154257748,2.17227988360039));
#40447=CARTESIAN_POINT('Ctrl Pts',(-12.0877133919531,4.65930703924313,2.33838315054028));
#40448=CARTESIAN_POINT('Ctrl Pts',(-12.0778119832033,4.45330143339801,2.59767923140541));
#40449=CARTESIAN_POINT('Ctrl Pts',(-12.0739356077645,4.366803567629,2.69623016690284));
#40450=CARTESIAN_POINT('Ctrl Pts',(-12.0646933833101,4.14612896190159,2.92357123365445));
#40451=CARTESIAN_POINT('Ctrl Pts',(-12.0594268420084,4.00772376869921,3.04716776291446));
#40452=CARTESIAN_POINT('Ctrl Pts',(-12.0453586268293,3.62722368060808,3.34101391083137));
#40453=CARTESIAN_POINT('Ctrl Pts',(-12.0364406835168,3.3736320493554,3.49487937456582));
#40454=CARTESIAN_POINT('Ctrl Pts',(-12.0188158713715,2.84936850747311,3.74003251133475));
#40455=CARTESIAN_POINT('Ctrl Pts',(-12.0101105720752,2.57938532281085,3.83352968685924));
#40456=CARTESIAN_POINT('Ctrl Pts',(-11.9900579652248,1.92897432069873,3.98426672819469));
#40457=CARTESIAN_POINT('Ctrl Pts',(-11.9793233272875,1.54723787739652,4.01629370329876));
#40458=CARTESIAN_POINT('Ctrl Pts',(-11.9600255472479,0.897272788894044,
3.97448380750347));
#40459=CARTESIAN_POINT('Ctrl Pts',(-11.9519430676385,0.633424037211266,
3.93066159074889));
#40460=CARTESIAN_POINT('Ctrl Pts',(-11.9323441145713,0.0119592206589963,
3.76396287315103));
#40461=CARTESIAN_POINT('Ctrl Pts',(-11.920802393218,-0.339284915436861,
3.61553825063958));
#40462=CARTESIAN_POINT('Ctrl Pts',(-11.9038095250028,-0.834646334145461,
3.31676895563602));
#40463=CARTESIAN_POINT('Ctrl Pts',(-11.8981176061492,-0.997843132716873,
3.20032165284924));
#40464=CARTESIAN_POINT('Ctrl Pts',(-11.8822880191012,-1.41301077947756,
2.85282643357032));
#40465=CARTESIAN_POINT('Ctrl Pts',(-11.8719415770262,-1.6455713910264,2.6002496039973));
#40466=CARTESIAN_POINT('Ctrl Pts',(-11.8496715525867,-2.07002341478387,
2.00537709549404));
#40467=CARTESIAN_POINT('Ctrl Pts',(-11.8377430377454,-2.25134971269181,
1.65483885383838));
#40468=CARTESIAN_POINT('Ctrl Pts',(-11.8210815019123,-2.43545043539192,
1.11533876887965));
#40469=CARTESIAN_POINT('Ctrl Pts',(-11.8159746586501,-2.48156811278056,
0.941863227818844));
#40470=CARTESIAN_POINT('Ctrl Pts',(-11.8032039756127,-2.564338138036,0.513344128743086));
#40471=CARTESIAN_POINT('Ctrl Pts',(-11.7954775775326,-2.58823907296245,
0.25661899120969));
#40472=CARTESIAN_POINT('Ctrl Pts',(-11.7876832506661,-2.5878486596569,-5.29887179842592E-6));
#40473=CARTESIAN_POINT('',(-11.3504675579642,4.87339933796339,1.9995945247564));
#40474=CARTESIAN_POINT('Ctrl Pts',(-11.7876832506661,-2.5878486596569,-5.29887179766264E-6));
#40475=CARTESIAN_POINT('Ctrl Pts',(-11.7846103880981,-2.58769474175568,
-0.101177752701668));
#40476=CARTESIAN_POINT('Ctrl Pts',(-11.7815269200527,-2.58376505817935,
-0.202352194944832));
#40477=CARTESIAN_POINT('Ctrl Pts',(-11.767159506054,-2.5479823868286,-0.67239604341351));
#40478=CARTESIAN_POINT('Ctrl Pts',(-11.7558727561899,-2.46962625916423,
-1.03803395302266));
#40479=CARTESIAN_POINT('Ctrl Pts',(-11.739409292753,-2.27534410088687,-1.5668017565316));
#40480=CARTESIAN_POINT('Ctrl Pts',(-11.7339326675503,-2.19566098586759,
-1.74228097956641));
#40481=CARTESIAN_POINT('Ctrl Pts',(-11.7180626751072,-1.93625154170422,
-2.21673614762035));
#40482=CARTESIAN_POINT('Ctrl Pts',(-11.7074698492726,-1.72910546764613,
-2.4994911803966));
#40483=CARTESIAN_POINT('Ctrl Pts',(-11.6858313890525,-1.24044482313432,
-3.0145296654611));
#40484=CARTESIAN_POINT('Ctrl Pts',(-11.674783142645,-0.95557542103658,-3.24457334198693));
#40485=CARTESIAN_POINT('Ctrl Pts',(-11.6591031158707,-0.496171389039835,
-3.52073443840331));
#40486=CARTESIAN_POINT('Ctrl Pts',(-11.6541761409979,-0.342265379603299,
-3.59982216006299));
#40487=CARTESIAN_POINT('Ctrl Pts',(-11.6342954682843,0.28277475538326,-3.87012213900222));
#40488=CARTESIAN_POINT('Ctrl Pts',(-11.6185640184131,0.78827110550862,-3.98091451149757));
#40489=CARTESIAN_POINT('Ctrl Pts',(-11.5968772493773,1.50366150222837,-4.00270758437244));
#40490=CARTESIAN_POINT('Ctrl Pts',(-11.5906341406035,1.71201481316968,-3.99305911453475));
#40491=CARTESIAN_POINT('Ctrl Pts',(-11.5793022612875,2.09485364618809,-3.94477507739172));
#40492=CARTESIAN_POINT('Ctrl Pts',(-11.5742512658516,2.26873754843006,-3.91066826854337));
#40493=CARTESIAN_POINT('Ctrl Pts',(-11.5609178711529,2.71142962776187,-3.79206837519196));
#40494=CARTESIAN_POINT('Ctrl Pts',(-11.5524721273212,2.97482797321889,-3.69004855288624));
#40495=CARTESIAN_POINT('Ctrl Pts',(-11.5294668643449,3.64940532079589,-3.34508319864017));
#40496=CARTESIAN_POINT('Ctrl Pts',(-11.5147555724654,4.0363775014314,-3.05299883030842));
#40497=CARTESIAN_POINT('Ctrl Pts',(-11.4954218216117,4.48438384752746,-2.56551816049437));
#40498=CARTESIAN_POINT('Ctrl Pts',(-11.4901560986607,4.59955745382197,-2.42076314139875));
#40499=CARTESIAN_POINT('Ctrl Pts',(-11.4788786389411,4.81671518935305,-2.10396141487377));
#40500=CARTESIAN_POINT('Ctrl Pts',(-11.4729223802691,4.91653276679171,-1.93170504376533));
#40501=CARTESIAN_POINT('Ctrl Pts',(-11.454290380336,5.18511036695413,-1.37827510867305));
#40502=CARTESIAN_POINT('Ctrl Pts',(-11.4414116708394,5.30941688375091,-0.974916313639125));
#40503=CARTESIAN_POINT('Ctrl Pts',(-11.4254481468296,5.38618076919228,-0.444564438851801));
#40504=CARTESIAN_POINT('Ctrl Pts',(-11.4219320593781,5.39797400151891,-0.325769559551178));
#40505=CARTESIAN_POINT('Ctrl Pts',(-11.4132876883655,5.41375293817565,-0.0287785142314743));
#40506=CARTESIAN_POINT('Ctrl Pts',(-11.4082243127921,5.41103538845619,0.1491799232229));
#40507=CARTESIAN_POINT('Ctrl Pts',(-11.3969631519055,5.37887832285405,0.532063032413717));
#40508=CARTESIAN_POINT('Ctrl Pts',(-11.3908068906373,5.34561745234865,0.735498453917561));
#40509=CARTESIAN_POINT('Ctrl Pts',(-11.3729998567251,5.206885987424,1.30744332532291));
#40510=CARTESIAN_POINT('Ctrl Pts',(-11.3611849998154,5.06375854791249,1.66721385919644));
#40511=CARTESIAN_POINT('Ctrl Pts',(-11.3497104489445,4.87307889585977,1.99938442467927));
#40512=CARTESIAN_POINT('',(-11.5809291742107,4.52769053405903,1.79999903547473));
#40513=CARTESIAN_POINT('',(-11.58094010768,4.527691453624,1.8));
#40514=CARTESIAN_POINT('Ctrl Pts',(-12.6,0.838694895738739,-3.55370611520755));
#40515=CARTESIAN_POINT('Ctrl Pts',(-12.5887641272916,1.16499951264074,-3.60576132676612));
#40516=CARTESIAN_POINT('Ctrl Pts',(-12.5770742688352,1.49857342709415,-3.61324189296731));
#40517=CARTESIAN_POINT('Ctrl Pts',(-12.5560586802186,2.12250050976799,-3.54138859102167));
#40518=CARTESIAN_POINT('Ctrl Pts',(-12.5471373056311,2.41003699969147,-3.47088661950422));
#40519=CARTESIAN_POINT('Ctrl Pts',(-12.5312999768489,2.8830601113705,-3.29055077504967));
#40520=CARTESIAN_POINT('Ctrl Pts',(-12.524252509136,3.07239137138561,-3.198855098942));
#40521=CARTESIAN_POINT('Ctrl Pts',(-12.5082823089597,3.46377174158328,-2.96588999220409));
#40522=CARTESIAN_POINT('Ctrl Pts',(-12.4993793701387,3.66244680102222,-2.81868848700558));
#40523=CARTESIAN_POINT('Ctrl Pts',(-12.4831637232564,4.01591068624947,-2.49492966001599));
#40524=CARTESIAN_POINT('Ctrl Pts',(-12.4760198719274,4.17110662319851,-2.32115475123233));
#40525=CARTESIAN_POINT('Ctrl Pts',(-12.4618210233891,4.44431682999554,-1.9491374193044));
#40526=CARTESIAN_POINT('Ctrl Pts',(-12.4546689448442,4.56280004195252,-1.75079245288425));
#40527=CARTESIAN_POINT('Ctrl Pts',(-12.439931361403,4.74718694464032,-1.36317401846108));
#40528=CARTESIAN_POINT('Ctrl Pts',(-12.4326747765561,4.81801285202238,-1.17619073207302));
#40529=CARTESIAN_POINT('Ctrl Pts',(-12.4063576468406,5.02342418869175,-0.456144231739891));
#40530=CARTESIAN_POINT('Ctrl Pts',(-12.3930138478682,5.02303169369089,0.00540451688270611));
#40531=CARTESIAN_POINT('Ctrl Pts',(-12.37109085781,4.96184573029325,0.688264102970618));
#40532=CARTESIAN_POINT('Ctrl Pts',(-12.3543545405096,4.86578260011855,1.15343937537345));
#40533=CARTESIAN_POINT('Ctrl Pts',(-12.3206718840845,4.40018540009682,2.05344488795971));
#40534=CARTESIAN_POINT('Ctrl Pts',(-12.3062079707334,4.11491495355461,2.41840678256053));
#40535=CARTESIAN_POINT('Ctrl Pts',(-12.283569485576,3.59309018571064,2.87243781592095));
#40536=CARTESIAN_POINT('Ctrl Pts',(-12.275620302287,3.39923678060795,3.00919228251818));
#40537=CARTESIAN_POINT('Ctrl Pts',(-12.2534491391618,2.83406207826439,3.33094760909004));
#40538=CARTESIAN_POINT('Ctrl Pts',(-12.2391421736313,2.43815303451555,3.47455698907783));
#40539=CARTESIAN_POINT('Ctrl Pts',(-12.2186112866935,1.80552823142804,3.58555148501812));
#40540=CARTESIAN_POINT('Ctrl Pts',(-12.2118094564931,1.57887832476874,3.60279712409267));
#40541=CARTESIAN_POINT('Ctrl Pts',(-12.1967053454351,1.11819157379905,3.59487576428567));
#40542=CARTESIAN_POINT('Ctrl Pts',(-12.1884339995617,0.883728304608525,
3.56799950559569));
#40543=CARTESIAN_POINT('Ctrl Pts',(-12.1722270298538,0.432344853464027,
3.47150505751602));
#40544=CARTESIAN_POINT('Ctrl Pts',(-12.1642973895436,0.214991410747773,
3.40335864083117));
#40545=CARTESIAN_POINT('Ctrl Pts',(-12.1413962581675,-0.432776918877695,
3.12926318578167));
#40546=CARTESIAN_POINT('Ctrl Pts',(-12.1276221440261,-0.83238108666093,
2.85440993772082));
#40547=CARTESIAN_POINT('Ctrl Pts',(-12.1035229055086,-1.30750875863012,
2.36934701595707));
#40548=CARTESIAN_POINT('Ctrl Pts',(-12.0961332943923,-1.43818770144354,
2.21124520291547));
#40549=CARTESIAN_POINT('Ctrl Pts',(-12.0822316782666,-1.67166744080994,
1.87248163943021));
#40550=CARTESIAN_POINT('Ctrl Pts',(-12.0757345443886,-1.77402337804945,
1.69164908071361));
#40551=CARTESIAN_POINT('Ctrl Pts',(-12.0620387872348,-1.95744861598317,
1.29133779792592));
#40552=CARTESIAN_POINT('Ctrl Pts',(-12.0548421196046,-2.03419661200844,
1.06982132872298));
#40553=CARTESIAN_POINT('Ctrl Pts',(-12.039453828938,-2.14304564689331,0.620278177587838));
#40554=CARTESIAN_POINT('Ctrl Pts',(-12.0311096529585,-2.17593528060915,
0.39226898784849));
#40555=CARTESIAN_POINT('Ctrl Pts',(-12.0116777247531,-2.20122601942365,
-0.166762796223493));
#40556=CARTESIAN_POINT('Ctrl Pts',(-12.0010460127369,-2.16959750059823,
-0.498536652134289));
#40557=CARTESIAN_POINT('Ctrl Pts',(-11.982907187648,-2.04047221966708,-1.05040640404938));
#40558=CARTESIAN_POINT('Ctrl Pts',(-11.9753521045416,-1.96414069249687,
-1.2756375235216));
#40559=CARTESIAN_POINT('Ctrl Pts',(-11.9479778753788,-1.62246649619555,
-2.02905179992013));
#40560=CARTESIAN_POINT('Ctrl Pts',(-11.9315011260785,-1.29930195159514,
-2.38930315827996));
#40561=CARTESIAN_POINT('Ctrl Pts',(-11.9132185835915,-0.902958965596291,
-2.76771196422866));
#40562=CARTESIAN_POINT('Ctrl Pts',(-11.905424226119,-0.715482172972858,
-2.9147589836845));
#40563=CARTESIAN_POINT('Ctrl Pts',(-11.8904653614941,-0.322663964575563,
-3.16399053807984));
#40564=CARTESIAN_POINT('Ctrl Pts',(-11.8834656399808,-0.119818097506157,
-3.26644888114137));
#40565=CARTESIAN_POINT('Ctrl Pts',(-11.8652109162172,0.391579322848854,
-3.46696903218546));
#40566=CARTESIAN_POINT('Ctrl Pts',(-11.8537230404663,0.707961006519751,
-3.54453244225553));
#40567=CARTESIAN_POINT('Ctrl Pts',(-11.8225903406543,1.61087350736643,-3.64197055765598));
#40568=CARTESIAN_POINT('Ctrl Pts',(-11.8090370118831,2.08903835372752,-3.5521639461965));
#40569=CARTESIAN_POINT('Ctrl Pts',(-11.7902657153263,2.62742750160701,-3.39322567344847));
#40570=CARTESIAN_POINT('Ctrl Pts',(-11.7827937637485,2.82255766322573,-3.31694616519985));
#40571=CARTESIAN_POINT('Ctrl Pts',(-11.7550408274743,3.52456462877589,-2.96994954477919));
#40572=CARTESIAN_POINT('Ctrl Pts',(-11.7410967124665,3.87591355900122,-2.64504773860041));
#40573=CARTESIAN_POINT('Ctrl Pts',(-11.7183255536125,4.35390464591097,-2.10338343352835));
#40574=CARTESIAN_POINT('Ctrl Pts',(-11.7045749484314,4.55763281573061,-1.78643682230267));
#40575=CARTESIAN_POINT('Ctrl Pts',(-11.6831068936867,4.80739207862655,-1.216534200417));
#40576=CARTESIAN_POINT('Ctrl Pts',(-11.675103963254,4.88319244853192,-0.977067848119014));
#40577=CARTESIAN_POINT('Ctrl Pts',(-11.6603829587993,4.97755178908749,-0.520997395951846));
#40578=CARTESIAN_POINT('Ctrl Pts',(-11.6536275474061,5.00250569713179,-0.305637573116578));
#40579=CARTESIAN_POINT('Ctrl Pts',(-11.6358967036407,5.01682165540191,0.238560233254273));
#40580=CARTESIAN_POINT('Ctrl Pts',(-11.6243174248663,4.98075713161062,0.565332704537782));
#40581=CARTESIAN_POINT('Ctrl Pts',(-11.6020225327239,4.81746533012486,1.20508148978053));
#40582=CARTESIAN_POINT('Ctrl Pts',(-11.5911778370602,4.69177805388506,1.51366930157276));
#40583=CARTESIAN_POINT('Ctrl Pts',(-11.5804418130255,4.52712444913299,1.79965561709499));
#40584=CARTESIAN_POINT('Ctrl Pts',(-12.95827988175,0.2420117051536,-3.405261127007));
#40585=CARTESIAN_POINT('Ctrl Pts',(-12.93620025074,0.871896082256,-3.62130845851));
#40586=CARTESIAN_POINT('Ctrl Pts',(-12.89204098874,2.25346886898,-3.694399003235));
#40587=CARTESIAN_POINT('Ctrl Pts',(-12.82580209574,4.073599630528,-2.695596833396));
#40588=CARTESIAN_POINT('Ctrl Pts',(-12.75956320274,5.094096064764,-0.8877177432058));
#40589=CARTESIAN_POINT('Ctrl Pts',(-12.69332430974,5.008999654046,1.18655771469));
#40590=CARTESIAN_POINT('Ctrl Pts',(-12.62708541674,3.843766347756,2.904733567434));
#40591=CARTESIAN_POINT('Ctrl Pts',(-12.56084652374,1.948124164015,3.751149176974));
#40592=CARTESIAN_POINT('Ctrl Pts',(-12.49460763074,-0.1090192521286,3.47178325432));
#40593=CARTESIAN_POINT('Ctrl Pts',(-12.42836873774,-1.710279489762,2.150477565921));
#40594=CARTESIAN_POINT('Ctrl Pts',(-12.36212984474,-2.375092347213,0.1837780628467));
#40595=CARTESIAN_POINT('Ctrl Pts',(-12.29589095173,-1.903936076344,-1.838076561439));
#40596=CARTESIAN_POINT('Ctrl Pts',(-12.22965205873,-0.4382135835323,-3.308292956026));
#40597=CARTESIAN_POINT('Ctrl Pts',(-12.16341316573,1.582191580049,-3.785639679087));
#40598=CARTESIAN_POINT('Ctrl Pts',(-12.09717427273,3.550907349452,-3.126839031206));
#40599=CARTESIAN_POINT('Ctrl Pts',(-12.03093537973,4.877145604737,-1.529675336636));
#40600=CARTESIAN_POINT('Ctrl Pts',(-11.96469648673,5.162671017333,0.5267674664513));
#40601=CARTESIAN_POINT('Ctrl Pts',(-11.92053722473,4.602606137466,1.79184174217));
#40602=CARTESIAN_POINT('Ctrl Pts',(-11.89845759373,4.176505297397,2.303572972466));
#40603=CARTESIAN_POINT('Ctrl Pts',(-12.8290540207,0.2420117051536,-3.405261127007));
#40604=CARTESIAN_POINT('Ctrl Pts',(-12.8069743897,0.871896082256,-3.62130845851));
#40605=CARTESIAN_POINT('Ctrl Pts',(-12.76281512769,2.25346886898,-3.694399003235));
#40606=CARTESIAN_POINT('Ctrl Pts',(-12.69657623469,4.073599630528,-2.695596833396));
#40607=CARTESIAN_POINT('Ctrl Pts',(-12.63033734169,5.094096064764,-0.8877177432058));
#40608=CARTESIAN_POINT('Ctrl Pts',(-12.56409844869,5.008999654046,1.18655771469));
#40609=CARTESIAN_POINT('Ctrl Pts',(-12.49785955569,3.843766347756,2.904733567434));
#40610=CARTESIAN_POINT('Ctrl Pts',(-12.43162066269,1.948124164015,3.751149176974));
#40611=CARTESIAN_POINT('Ctrl Pts',(-12.36538176969,-0.1090192521286,3.47178325432));
#40612=CARTESIAN_POINT('Ctrl Pts',(-12.29914287669,-1.710279489762,2.150477565921));
#40613=CARTESIAN_POINT('Ctrl Pts',(-12.23290398369,-2.375092347213,0.1837780628467));
#40614=CARTESIAN_POINT('Ctrl Pts',(-12.16666509068,-1.903936076344,-1.838076561439));
#40615=CARTESIAN_POINT('Ctrl Pts',(-12.10042619768,-0.4382135835323,-3.308292956026));
#40616=CARTESIAN_POINT('Ctrl Pts',(-12.03418730468,1.582191580049,-3.785639679087));
#40617=CARTESIAN_POINT('Ctrl Pts',(-11.96794841168,3.550907349452,-3.126839031206));
#40618=CARTESIAN_POINT('Ctrl Pts',(-11.90170951868,4.877145604737,-1.529675336636));
#40619=CARTESIAN_POINT('Ctrl Pts',(-11.83547062568,5.162671017333,0.5267674664513));
#40620=CARTESIAN_POINT('Ctrl Pts',(-11.79131136368,4.602606137466,1.79184174217));
#40621=CARTESIAN_POINT('Ctrl Pts',(-11.76923173268,4.176505297397,2.303572972466));
#40622=CARTESIAN_POINT('Ctrl Pts',(-12.69982815965,0.2420117051536,-3.405261127007));
#40623=CARTESIAN_POINT('Ctrl Pts',(-12.67774852865,0.871896082256,-3.62130845851));
#40624=CARTESIAN_POINT('Ctrl Pts',(-12.63358926664,2.25346886898,-3.694399003235));
#40625=CARTESIAN_POINT('Ctrl Pts',(-12.56735037364,4.073599630528,-2.695596833396));
#40626=CARTESIAN_POINT('Ctrl Pts',(-12.50111148064,5.094096064764,-0.8877177432058));
#40627=CARTESIAN_POINT('Ctrl Pts',(-12.43487258764,5.008999654046,1.18655771469));
#40628=CARTESIAN_POINT('Ctrl Pts',(-12.36863369464,3.843766347756,2.904733567434));
#40629=CARTESIAN_POINT('Ctrl Pts',(-12.30239480164,1.948124164015,3.751149176974));
#40630=CARTESIAN_POINT('Ctrl Pts',(-12.23615590864,-0.1090192521286,3.47178325432));
#40631=CARTESIAN_POINT('Ctrl Pts',(-12.16991701564,-1.710279489762,2.150477565921));
#40632=CARTESIAN_POINT('Ctrl Pts',(-12.10367812264,-2.375092347213,0.1837780628467));
#40633=CARTESIAN_POINT('Ctrl Pts',(-12.03743922964,-1.903936076344,-1.838076561439));
#40634=CARTESIAN_POINT('Ctrl Pts',(-11.97120033663,-0.4382135835323,-3.308292956026));
#40635=CARTESIAN_POINT('Ctrl Pts',(-11.90496144363,1.582191580049,-3.785639679087));
#40636=CARTESIAN_POINT('Ctrl Pts',(-11.83872255063,3.550907349452,-3.126839031206));
#40637=CARTESIAN_POINT('Ctrl Pts',(-11.77248365763,4.877145604737,-1.529675336636));
#40638=CARTESIAN_POINT('Ctrl Pts',(-11.70624476463,5.162671017333,0.5267674664513));
#40639=CARTESIAN_POINT('Ctrl Pts',(-11.66208550263,4.602606137466,1.79184174217));
#40640=CARTESIAN_POINT('Ctrl Pts',(-11.64000587163,4.176505297397,2.303572972466));
#40641=CARTESIAN_POINT('Ctrl Pts',(-12.5706022986,0.2420117051536,-3.405261127007));
#40642=CARTESIAN_POINT('Ctrl Pts',(-12.5485226676,0.871896082256,-3.62130845851));
#40643=CARTESIAN_POINT('Ctrl Pts',(-12.5043634056,2.25346886898,-3.694399003235));
#40644=CARTESIAN_POINT('Ctrl Pts',(-12.43812451259,4.073599630528,-2.695596833396));
#40645=CARTESIAN_POINT('Ctrl Pts',(-12.37188561959,5.094096064764,-0.8877177432058));
#40646=CARTESIAN_POINT('Ctrl Pts',(-12.30564672659,5.008999654046,1.18655771469));
#40647=CARTESIAN_POINT('Ctrl Pts',(-12.23940783359,3.843766347756,2.904733567434));
#40648=CARTESIAN_POINT('Ctrl Pts',(-12.17316894059,1.948124164015,3.751149176974));
#40649=CARTESIAN_POINT('Ctrl Pts',(-12.10693004759,-0.1090192521286,3.47178325432));
#40650=CARTESIAN_POINT('Ctrl Pts',(-12.04069115459,-1.710279489762,2.150477565921));
#40651=CARTESIAN_POINT('Ctrl Pts',(-11.97445226159,-2.375092347213,0.1837780628467));
#40652=CARTESIAN_POINT('Ctrl Pts',(-11.90821336859,-1.903936076344,-1.838076561439));
#40653=CARTESIAN_POINT('Ctrl Pts',(-11.84197447558,-0.4382135835323,-3.308292956026));
#40654=CARTESIAN_POINT('Ctrl Pts',(-11.77573558258,1.582191580049,-3.785639679087));
#40655=CARTESIAN_POINT('Ctrl Pts',(-11.70949668958,3.550907349452,-3.126839031206));
#40656=CARTESIAN_POINT('Ctrl Pts',(-11.64325779658,4.877145604737,-1.529675336636));
#40657=CARTESIAN_POINT('Ctrl Pts',(-11.57701890358,5.162671017333,0.5267674664513));
#40658=CARTESIAN_POINT('Ctrl Pts',(-11.53285964158,4.602606137466,1.79184174217));
#40659=CARTESIAN_POINT('Ctrl Pts',(-11.51078001058,4.176505297397,2.303572972466));
#40660=CARTESIAN_POINT('',(-11.86905989232,4.527691453624,1.8));
#40661=CARTESIAN_POINT('Ctrl Pts',(-11.96883879157,4.990278823326,0.3763024677636));
#40662=CARTESIAN_POINT('Ctrl Pts',(-11.94175545824,4.90489850173,1.188641964648));
#40663=CARTESIAN_POINT('Ctrl Pts',(-11.88758879157,4.159906564498,2.74938154341));
#40664=CARTESIAN_POINT('Ctrl Pts',(-11.80633879157,1.816485745292,3.867708124722));
#40665=CARTESIAN_POINT('Ctrl Pts',(-11.72508879157,-0.7080347390856,3.261458897656));
#40666=CARTESIAN_POINT('Ctrl Pts',(-11.64383879157,-2.288549945275,1.201740552274));
#40667=CARTESIAN_POINT('Ctrl Pts',(-11.56258879157,-2.220586231791,-1.393654028254));
#40668=CARTESIAN_POINT('Ctrl Pts',(-11.48133879157,-0.5344423398995,-3.367872149436));
#40669=CARTESIAN_POINT('Ctrl Pts',(-11.40008879157,2.018355591389,-3.841006095744));
#40670=CARTESIAN_POINT('Ctrl Pts',(-11.31883879157,4.300004419211,-2.602171624442));
#40671=CARTESIAN_POINT('Ctrl Pts',(-11.23758879157,5.293554962079,-0.2035285038406));
#40672=CARTESIAN_POINT('Ctrl Pts',(-11.15633879157,4.556173683172,2.285828984956));
#40673=CARTESIAN_POINT('Ctrl Pts',(-11.07508879157,2.416517383734,3.756374013533));
#40674=CARTESIAN_POINT('Ctrl Pts',(-10.99383879157,-0.1717518438912,3.552672808756));
#40675=CARTESIAN_POINT('Ctrl Pts',(-10.91258879157,-2.055021498606,1.765516636523));
#40676=CARTESIAN_POINT('Ctrl Pts',(-10.83133879157,-2.393903084153,-0.8085445604757));
#40677=CARTESIAN_POINT('Ctrl Pts',(-10.75008879157,-1.037354340631,-3.022230916284));
#40678=CARTESIAN_POINT('Ctrl Pts',(-10.66883879157,1.41,-3.888884541858));
#40679=CARTESIAN_POINT('Ctrl Pts',(-10.58758879157,3.857354340631,-3.022230916284));
#40680=CARTESIAN_POINT('Ctrl Pts',(-10.50633879157,5.213903084153,-0.8085445604757));
#40681=CARTESIAN_POINT('Ctrl Pts',(-10.42508879157,4.875021498606,1.765516636523));
#40682=CARTESIAN_POINT('Ctrl Pts',(-10.34383879157,2.991751843891,3.552672808756));
#40683=CARTESIAN_POINT('Ctrl Pts',(-10.26258879157,0.4034826162665,3.756374013533));
#40684=CARTESIAN_POINT('Ctrl Pts',(-10.18133879157,-1.736173683172,2.285828984956));
#40685=CARTESIAN_POINT('Ctrl Pts',(-10.10008879157,-2.473554962079,-0.2035285038406));
#40686=CARTESIAN_POINT('Ctrl Pts',(-10.01883879157,-1.480004419211,-2.602171624442));
#40687=CARTESIAN_POINT('Ctrl Pts',(-9.937588791574,0.8016444086106,-3.841006095744));
#40688=CARTESIAN_POINT('Ctrl Pts',(-9.856338791574,3.3544423399,-3.367872149436));
#40689=CARTESIAN_POINT('Ctrl Pts',(-9.775088791574,5.040586231791,-1.393654028254));
#40690=CARTESIAN_POINT('Ctrl Pts',(-9.693838791574,5.108549945275,1.201740552274));
#40691=CARTESIAN_POINT('Ctrl Pts',(-9.612588791574,3.528034739086,3.261458897656));
#40692=CARTESIAN_POINT('Ctrl Pts',(-9.531338791574,1.003514254708,3.867708124722));
#40693=CARTESIAN_POINT('Ctrl Pts',(-9.450088791574,-1.339906564498,2.74938154341));
#40694=CARTESIAN_POINT('Ctrl Pts',(-9.395922124908,-2.08489850173,1.188641964648));
#40695=CARTESIAN_POINT('Ctrl Pts',(-9.368838791574,-2.170278823326,0.3763024677635));
#40696=CARTESIAN_POINT('Ctrl Pts',(-11.83961293052,4.990278823326,0.3763024677636));
#40697=CARTESIAN_POINT('Ctrl Pts',(-11.81252959719,4.90489850173,1.188641964648));
#40698=CARTESIAN_POINT('Ctrl Pts',(-11.75836293052,4.159906564498,2.74938154341));
#40699=CARTESIAN_POINT('Ctrl Pts',(-11.67711293052,1.816485745292,3.867708124722));
#40700=CARTESIAN_POINT('Ctrl Pts',(-11.59586293052,-0.7080347390856,3.261458897656));
#40701=CARTESIAN_POINT('Ctrl Pts',(-11.51461293052,-2.288549945275,1.201740552274));
#40702=CARTESIAN_POINT('Ctrl Pts',(-11.43336293052,-2.220586231791,-1.393654028254));
#40703=CARTESIAN_POINT('Ctrl Pts',(-11.35211293052,-0.5344423398995,-3.367872149436));
#40704=CARTESIAN_POINT('Ctrl Pts',(-11.27086293052,2.018355591389,-3.841006095744));
#40705=CARTESIAN_POINT('Ctrl Pts',(-11.18961293052,4.300004419211,-2.602171624442));
#40706=CARTESIAN_POINT('Ctrl Pts',(-11.10836293052,5.293554962079,-0.2035285038406));
#40707=CARTESIAN_POINT('Ctrl Pts',(-11.02711293052,4.556173683172,2.285828984956));
#40708=CARTESIAN_POINT('Ctrl Pts',(-10.94586293052,2.416517383734,3.756374013533));
#40709=CARTESIAN_POINT('Ctrl Pts',(-10.86461293052,-0.1717518438912,3.552672808756));
#40710=CARTESIAN_POINT('Ctrl Pts',(-10.78336293052,-2.055021498606,1.765516636523));
#40711=CARTESIAN_POINT('Ctrl Pts',(-10.70211293052,-2.393903084153,-0.8085445604757));
#40712=CARTESIAN_POINT('Ctrl Pts',(-10.62086293052,-1.037354340631,-3.022230916284));
#40713=CARTESIAN_POINT('Ctrl Pts',(-10.53961293052,1.41,-3.888884541858));
#40714=CARTESIAN_POINT('Ctrl Pts',(-10.45836293052,3.857354340631,-3.022230916284));
#40715=CARTESIAN_POINT('Ctrl Pts',(-10.37711293052,5.213903084153,-0.8085445604757));
#40716=CARTESIAN_POINT('Ctrl Pts',(-10.29586293052,4.875021498606,1.765516636523));
#40717=CARTESIAN_POINT('Ctrl Pts',(-10.21461293052,2.991751843891,3.552672808756));
#40718=CARTESIAN_POINT('Ctrl Pts',(-10.13336293052,0.4034826162665,3.756374013533));
#40719=CARTESIAN_POINT('Ctrl Pts',(-10.05211293052,-1.736173683172,2.285828984956));
#40720=CARTESIAN_POINT('Ctrl Pts',(-9.970862930525,-2.473554962079,-0.2035285038406));
#40721=CARTESIAN_POINT('Ctrl Pts',(-9.889612930525,-1.480004419211,-2.602171624442));
#40722=CARTESIAN_POINT('Ctrl Pts',(-9.808362930525,0.8016444086106,-3.841006095744));
#40723=CARTESIAN_POINT('Ctrl Pts',(-9.727112930525,3.3544423399,-3.367872149436));
#40724=CARTESIAN_POINT('Ctrl Pts',(-9.645862930525,5.040586231791,-1.393654028254));
#40725=CARTESIAN_POINT('Ctrl Pts',(-9.564612930525,5.108549945275,1.201740552274));
#40726=CARTESIAN_POINT('Ctrl Pts',(-9.483362930525,3.528034739086,3.261458897656));
#40727=CARTESIAN_POINT('Ctrl Pts',(-9.402112930525,1.003514254708,3.867708124722));
#40728=CARTESIAN_POINT('Ctrl Pts',(-9.320862930525,-1.339906564498,2.74938154341));
#40729=CARTESIAN_POINT('Ctrl Pts',(-9.266696263858,-2.08489850173,1.188641964648));
#40730=CARTESIAN_POINT('Ctrl Pts',(-9.239612930525,-2.170278823326,0.3763024677635));
#40731=CARTESIAN_POINT('Ctrl Pts',(-11.71038706948,4.990278823326,0.3763024677636));
#40732=CARTESIAN_POINT('Ctrl Pts',(-11.68330373614,4.90489850173,1.188641964648));
#40733=CARTESIAN_POINT('Ctrl Pts',(-11.62913706948,4.159906564498,2.74938154341));
#40734=CARTESIAN_POINT('Ctrl Pts',(-11.54788706948,1.816485745292,3.867708124722));
#40735=CARTESIAN_POINT('Ctrl Pts',(-11.46663706948,-0.7080347390856,3.261458897656));
#40736=CARTESIAN_POINT('Ctrl Pts',(-11.38538706948,-2.288549945275,1.201740552274));
#40737=CARTESIAN_POINT('Ctrl Pts',(-11.30413706948,-2.220586231791,-1.393654028254));
#40738=CARTESIAN_POINT('Ctrl Pts',(-11.22288706948,-0.5344423398995,-3.367872149436));
#40739=CARTESIAN_POINT('Ctrl Pts',(-11.14163706948,2.018355591389,-3.841006095744));
#40740=CARTESIAN_POINT('Ctrl Pts',(-11.06038706948,4.300004419211,-2.602171624442));
#40741=CARTESIAN_POINT('Ctrl Pts',(-10.97913706948,5.293554962079,-0.2035285038406));
#40742=CARTESIAN_POINT('Ctrl Pts',(-10.89788706948,4.556173683172,2.285828984956));
#40743=CARTESIAN_POINT('Ctrl Pts',(-10.81663706948,2.416517383734,3.756374013533));
#40744=CARTESIAN_POINT('Ctrl Pts',(-10.73538706948,-0.1717518438912,3.552672808756));
#40745=CARTESIAN_POINT('Ctrl Pts',(-10.65413706948,-2.055021498606,1.765516636523));
#40746=CARTESIAN_POINT('Ctrl Pts',(-10.57288706948,-2.393903084153,-0.8085445604757));
#40747=CARTESIAN_POINT('Ctrl Pts',(-10.49163706948,-1.037354340631,-3.022230916284));
#40748=CARTESIAN_POINT('Ctrl Pts',(-10.41038706948,1.41,-3.888884541858));
#40749=CARTESIAN_POINT('Ctrl Pts',(-10.32913706948,3.857354340631,-3.022230916284));
#40750=CARTESIAN_POINT('Ctrl Pts',(-10.24788706948,5.213903084153,-0.8085445604757));
#40751=CARTESIAN_POINT('Ctrl Pts',(-10.16663706948,4.875021498606,1.765516636523));
#40752=CARTESIAN_POINT('Ctrl Pts',(-10.08538706948,2.991751843891,3.552672808756));
#40753=CARTESIAN_POINT('Ctrl Pts',(-10.00413706948,0.4034826162665,3.756374013533));
#40754=CARTESIAN_POINT('Ctrl Pts',(-9.922887069475,-1.736173683172,2.285828984956));
#40755=CARTESIAN_POINT('Ctrl Pts',(-9.841637069475,-2.473554962079,-0.2035285038406));
#40756=CARTESIAN_POINT('Ctrl Pts',(-9.760387069475,-1.480004419211,-2.602171624442));
#40757=CARTESIAN_POINT('Ctrl Pts',(-9.679137069475,0.8016444086106,-3.841006095744));
#40758=CARTESIAN_POINT('Ctrl Pts',(-9.597887069475,3.3544423399,-3.367872149436));
#40759=CARTESIAN_POINT('Ctrl Pts',(-9.516637069475,5.040586231791,-1.393654028254));
#40760=CARTESIAN_POINT('Ctrl Pts',(-9.435387069475,5.108549945275,1.201740552274));
#40761=CARTESIAN_POINT('Ctrl Pts',(-9.354137069475,3.528034739086,3.261458897656));
#40762=CARTESIAN_POINT('Ctrl Pts',(-9.272887069475,1.003514254708,3.867708124722));
#40763=CARTESIAN_POINT('Ctrl Pts',(-9.191637069475,-1.339906564498,2.74938154341));
#40764=CARTESIAN_POINT('Ctrl Pts',(-9.137470402809,-2.08489850173,1.188641964648));
#40765=CARTESIAN_POINT('Ctrl Pts',(-9.110387069475,-2.170278823326,0.3763024677635));
#40766=CARTESIAN_POINT('Ctrl Pts',(-11.58116120843,4.990278823326,0.3763024677636));
#40767=CARTESIAN_POINT('Ctrl Pts',(-11.55407787509,4.90489850173,1.188641964648));
#40768=CARTESIAN_POINT('Ctrl Pts',(-11.49991120843,4.159906564498,2.74938154341));
#40769=CARTESIAN_POINT('Ctrl Pts',(-11.41866120843,1.816485745292,3.867708124722));
#40770=CARTESIAN_POINT('Ctrl Pts',(-11.33741120843,-0.7080347390856,3.261458897656));
#40771=CARTESIAN_POINT('Ctrl Pts',(-11.25616120843,-2.288549945275,1.201740552274));
#40772=CARTESIAN_POINT('Ctrl Pts',(-11.17491120843,-2.220586231791,-1.393654028254));
#40773=CARTESIAN_POINT('Ctrl Pts',(-11.09366120843,-0.5344423398995,-3.367872149436));
#40774=CARTESIAN_POINT('Ctrl Pts',(-11.01241120843,2.018355591389,-3.841006095744));
#40775=CARTESIAN_POINT('Ctrl Pts',(-10.93116120843,4.300004419211,-2.602171624442));
#40776=CARTESIAN_POINT('Ctrl Pts',(-10.84991120843,5.293554962079,-0.2035285038406));
#40777=CARTESIAN_POINT('Ctrl Pts',(-10.76866120843,4.556173683172,2.285828984956));
#40778=CARTESIAN_POINT('Ctrl Pts',(-10.68741120843,2.416517383734,3.756374013533));
#40779=CARTESIAN_POINT('Ctrl Pts',(-10.60616120843,-0.1717518438912,3.552672808756));
#40780=CARTESIAN_POINT('Ctrl Pts',(-10.52491120843,-2.055021498606,1.765516636523));
#40781=CARTESIAN_POINT('Ctrl Pts',(-10.44366120843,-2.393903084153,-0.8085445604757));
#40782=CARTESIAN_POINT('Ctrl Pts',(-10.36241120843,-1.037354340631,-3.022230916284));
#40783=CARTESIAN_POINT('Ctrl Pts',(-10.28116120843,1.41,-3.888884541858));
#40784=CARTESIAN_POINT('Ctrl Pts',(-10.19991120843,3.857354340631,-3.022230916284));
#40785=CARTESIAN_POINT('Ctrl Pts',(-10.11866120843,5.213903084153,-0.8085445604757));
#40786=CARTESIAN_POINT('Ctrl Pts',(-10.03741120843,4.875021498606,1.765516636523));
#40787=CARTESIAN_POINT('Ctrl Pts',(-9.956161208426,2.991751843891,3.552672808756));
#40788=CARTESIAN_POINT('Ctrl Pts',(-9.874911208426,0.4034826162665,3.756374013533));
#40789=CARTESIAN_POINT('Ctrl Pts',(-9.793661208426,-1.736173683172,2.285828984956));
#40790=CARTESIAN_POINT('Ctrl Pts',(-9.712411208426,-2.473554962079,-0.2035285038406));
#40791=CARTESIAN_POINT('Ctrl Pts',(-9.631161208426,-1.480004419211,-2.602171624442));
#40792=CARTESIAN_POINT('Ctrl Pts',(-9.549911208426,0.8016444086106,-3.841006095744));
#40793=CARTESIAN_POINT('Ctrl Pts',(-9.468661208426,3.3544423399,-3.367872149436));
#40794=CARTESIAN_POINT('Ctrl Pts',(-9.387411208426,5.040586231791,-1.393654028254));
#40795=CARTESIAN_POINT('Ctrl Pts',(-9.306161208426,5.108549945275,1.201740552274));
#40796=CARTESIAN_POINT('Ctrl Pts',(-9.224911208426,3.528034739086,3.261458897656));
#40797=CARTESIAN_POINT('Ctrl Pts',(-9.143661208426,1.003514254708,3.867708124722));
#40798=CARTESIAN_POINT('Ctrl Pts',(-9.062411208426,-1.339906564498,2.74938154341));
#40799=CARTESIAN_POINT('Ctrl Pts',(-9.008244541759,-2.08489850173,1.188641964648));
#40800=CARTESIAN_POINT('Ctrl Pts',(-8.981161208426,-2.170278823326,0.3763024677635));
#40801=CARTESIAN_POINT('',(-9.08094010928004,-1.70769139852697,1.7999999682789));
#40802=CARTESIAN_POINT('Ctrl Pts',(-11.5809617506456,4.5260831847495,1.79907626034106));
#40803=CARTESIAN_POINT('Ctrl Pts',(-11.5684450873295,4.3378600575804,2.1262786819466));
#40804=CARTESIAN_POINT('Ctrl Pts',(-11.5538980982549,4.06794174588371,2.48158171780862));
#40805=CARTESIAN_POINT('Ctrl Pts',(-11.5214314833192,3.30533424391916,3.09434306772659));
#40806=CARTESIAN_POINT('Ctrl Pts',(-11.5058149680683,2.87955875891145,3.31694181014995));
#40807=CARTESIAN_POINT('Ctrl Pts',(-11.4743697636094,1.97084917822777,3.58784773144761));
#40808=CARTESIAN_POINT('Ctrl Pts',(-11.458927499448,1.49858395212458,3.62974369515122));
#40809=CARTESIAN_POINT('Ctrl Pts',(-11.4278797681144,0.567783349223922,
3.52751529061047));
#40810=CARTESIAN_POINT('Ctrl Pts',(-11.4125981009723,0.118590523682951,
3.39023797385841));
#40811=CARTESIAN_POINT('Ctrl Pts',(-11.3789404175473,-0.776750715579688,
2.91391088646765));
#40812=CARTESIAN_POINT('Ctrl Pts',(-11.363281015408,-1.12631120018392,2.58165267968671));
#40813=CARTESIAN_POINT('Ctrl Pts',(-11.3354748649634,-1.65756052459529,
1.93228316468842));
#40814=CARTESIAN_POINT('Ctrl Pts',(-11.3205629146619,-1.87884143765697,
1.53172977266817));
#40815=CARTESIAN_POINT('Ctrl Pts',(-11.2898146617579,-2.16265954300596,
0.650116766645046));
#40816=CARTESIAN_POINT('Ctrl Pts',(-11.2740125696461,-2.21484896790171,
0.166880112239114));
#40817=CARTESIAN_POINT('Ctrl Pts',(-11.2452857971753,-2.14178934307187,
-0.696743368548383));
#40818=CARTESIAN_POINT('Ctrl Pts',(-11.2299872318515,-2.04216345247547,
-1.15659791290261));
#40819=CARTESIAN_POINT('Ctrl Pts',(-11.1965187948146,-1.58161797675723,
-2.05390441834313));
#40820=CARTESIAN_POINT('Ctrl Pts',(-11.1809028018103,-1.28346141477642,
-2.43059522198911));
#40821=CARTESIAN_POINT('Ctrl Pts',(-11.1494553479051,-0.563858309517445,
-3.04814548837911));
#40822=CARTESIAN_POINT('Ctrl Pts',(-11.1340098599798,-0.149535385823463,
-3.27882544829088));
#40823=CARTESIAN_POINT('Ctrl Pts',(-11.1029565216824,0.742348833731377,
-3.56464372425645));
#40824=CARTESIAN_POINT('Ctrl Pts',(-11.0876732494035,1.20855364600226,-3.62224850779717));
#40825=CARTESIAN_POINT('Ctrl Pts',(-11.0540224073665,2.22006102775741,-3.55194694257004));
#40826=CARTESIAN_POINT('Ctrl Pts',(-11.0383675007242,2.67453375101345,-3.39102207324724));
#40827=CARTESIAN_POINT('Ctrl Pts',(-11.0105554436935,3.42438260732585,-3.01428152575009));
#40828=CARTESIAN_POINT('Ctrl Pts',(-10.995646825868,3.78954524063164,-2.73864661536387));
#40829=CARTESIAN_POINT('Ctrl Pts',(-10.9649039633072,4.40784438986543,-2.04929227481183));
#40830=CARTESIAN_POINT('Ctrl Pts',(-10.949101116759,4.65238613785367,-1.62921992321605));
#40831=CARTESIAN_POINT('Ctrl Pts',(-10.920381728934,4.93742752730497,-0.810959839651295));
#40832=CARTESIAN_POINT('Ctrl Pts',(-10.9050839876911,5.0338584634379,-0.350448986549228));
#40833=CARTESIAN_POINT('Ctrl Pts',(-10.8716136041178,4.97891930544053,0.656699056108514));
#40834=CARTESIAN_POINT('Ctrl Pts',(-10.8559955478887,4.86008836875808,1.12224707164084));
#40835=CARTESIAN_POINT('Ctrl Pts',(-10.8245490450561,4.45453566345954,1.97938216415778));
#40836=CARTESIAN_POINT('Ctrl Pts',(-10.8091065245231,4.17024380133705,2.35881196450516));
#40837=CARTESIAN_POINT('Ctrl Pts',(-10.7780497954225,3.47214510051836,2.98330370028508));
#40838=CARTESIAN_POINT('Ctrl Pts',(-10.7627635570628,3.06977273055838,3.22589817344446));
#40839=CARTESIAN_POINT('Ctrl Pts',(-10.7291162063469,2.11747273302227,3.57376459988511));
#40840=CARTESIAN_POINT('Ctrl Pts',(-10.7134646975643,1.63698623022721,3.61203190002298));
#40841=CARTESIAN_POINT('Ctrl Pts',(-10.6856469276413,0.798531261064757,
3.57346703035343));
#40842=CARTESIAN_POINT('Ctrl Pts',(-10.6707424649389,0.352879643376062,
3.47053387849982));
#40843=CARTESIAN_POINT('Ctrl Pts',(-10.6400060097322,-0.492512987916646,
3.09309930974023));
#40844=CARTESIAN_POINT('Ctrl Pts',(-10.6242022843195,-0.887025969969569,
2.8091196588916));
#40845=CARTESIAN_POINT('Ctrl Pts',(-10.5954908481819,-1.48059838918454,
2.17820084892424));
#40846=CARTESIAN_POINT('Ctrl Pts',(-10.5801941864632,-1.75636379133539,
1.7970258246446));
#40847=CARTESIAN_POINT('Ctrl Pts',(-10.546722144091,-2.11671818989919,0.854902102534742));
#40848=CARTESIAN_POINT('Ctrl Pts',(-10.5311017518598,-2.19793715412459,
0.381267556022045));
#40849=CARTESIAN_POINT('Ctrl Pts',(-10.4996563495939,-2.17689468407349,
-0.566708949154503));
#40850=CARTESIAN_POINT('Ctrl Pts',(-10.484217199875,-2.07199190034994,-1.02896894673998));
#40851=CARTESIAN_POINT('Ctrl Pts',(-10.4531565975826,-1.6889857158799,-1.88386424768358));
#40852=CARTESIAN_POINT('Ctrl Pts',(-10.4378669742447,-1.42033608863859,
-2.26946266636307));
#40853=CARTESIAN_POINT('Ctrl Pts',(-10.4042232279263,-0.692530601496339,
-2.97513752621574));
#40854=CARTESIAN_POINT('Ctrl Pts',(-10.388575550876,-0.269500817280129,
-3.20590346729835));
#40855=CARTESIAN_POINT('Ctrl Pts',(-10.3607516492302,0.512062543121538,
-3.51243382004678));
#40856=CARTESIAN_POINT('Ctrl Pts',(-10.3458519718052,0.960835502840228,
-3.6));
#40857=CARTESIAN_POINT('Ctrl Pts',(-10.3160282435544,1.85916449715974,-3.6));
#40858=CARTESIAN_POINT('Ctrl Pts',(-10.3011285661188,2.30793745687843,-3.51243382004679));
#40859=CARTESIAN_POINT('Ctrl Pts',(-10.2733046644732,3.0895008172801,-3.20590346729836));
#40860=CARTESIAN_POINT('Ctrl Pts',(-10.2576569874231,3.51253060149631,-2.97513752621576));
#40861=CARTESIAN_POINT('Ctrl Pts',(-10.2240132411048,4.24033608863857,-2.2694626663631));
#40862=CARTESIAN_POINT('Ctrl Pts',(-10.2087236177669,4.50898571587988,-1.88386424768361));
#40863=CARTESIAN_POINT('Ctrl Pts',(-10.1776630154745,4.89199190034992,-1.02896894674003));
#40864=CARTESIAN_POINT('Ctrl Pts',(-10.1622238657555,4.99689468407348,-0.566708949154548));
#40865=CARTESIAN_POINT('Ctrl Pts',(-10.1307784634897,5.0179371541246,0.38126755602198));
#40866=CARTESIAN_POINT('Ctrl Pts',(-10.1151580712585,4.9367181898992,0.854902102534665));
#40867=CARTESIAN_POINT('Ctrl Pts',(-10.0816860288865,4.57636379133542,1.79702582464447));
#40868=CARTESIAN_POINT('Ctrl Pts',(-10.066389367168,4.30059838918458,2.17820084892409));
#40869=CARTESIAN_POINT('Ctrl Pts',(-10.0376779310305,3.70702596996962,2.80911965889149));
#40870=CARTESIAN_POINT('Ctrl Pts',(-10.021874205618,3.31251298791666,3.09309930974017));
#40871=CARTESIAN_POINT('Ctrl Pts',(-9.99113775041132,2.46712035662394,3.47053387849983));
#40872=CARTESIAN_POINT('Ctrl Pts',(-9.97623328770884,2.02146873893528,3.57346703035345));
#40873=CARTESIAN_POINT('Ctrl Pts',(-9.94841551778588,1.18301376977285,3.61203190002298));
#40874=CARTESIAN_POINT('Ctrl Pts',(-9.93276400900317,0.702527266977886,
3.57376459988507));
#40875=CARTESIAN_POINT('Ctrl Pts',(-9.8991166582872,-0.249772730558297,
3.22589817344437));
#40876=CARTESIAN_POINT('Ctrl Pts',(-9.88383041992763,-0.652145100518404,
2.9833037002849));
#40877=CARTESIAN_POINT('Ctrl Pts',(-9.85277369082696,-1.35024380133725,
2.35881196450481));
#40878=CARTESIAN_POINT('Ctrl Pts',(-9.8373311702941,-1.63453566345976,1.97938216415737));
#40879=CARTESIAN_POINT('Ctrl Pts',(-9.80588466746157,-2.04008836875821,
1.12224707164038));
#40880=CARTESIAN_POINT('Ctrl Pts',(-9.79026661123261,-2.15891930544059,
0.656699056108114));
#40881=CARTESIAN_POINT('Ctrl Pts',(-9.75679622765946,-2.21385846343786,
-0.350448986549525));
#40882=CARTESIAN_POINT('Ctrl Pts',(-9.74149848641643,-2.1174275273049,-0.810959839651566));
#40883=CARTESIAN_POINT('Ctrl Pts',(-9.71277909859132,-1.83238613785356,
-1.6292199232163));
#40884=CARTESIAN_POINT('Ctrl Pts',(-9.69697625204285,-1.58784438986529,
-2.0492922748121));
#40885=CARTESIAN_POINT('Ctrl Pts',(-9.66623338948216,-0.969545240631444,
-2.73864661536413));
#40886=CARTESIAN_POINT('Ctrl Pts',(-9.65132477165689,-0.604382607325644,
-3.01428152575034));
#40887=CARTESIAN_POINT('Ctrl Pts',(-9.62351271462641,0.145466248986811,
-3.39102207324742));
#40888=CARTESIAN_POINT('Ctrl Pts',(-9.60785780798448,0.599938972242795,
-3.55194694257012));
#40889=CARTESIAN_POINT('Ctrl Pts',(-9.57420696594746,1.61144635399806,-3.62224850779716));
#40890=CARTESIAN_POINT('Ctrl Pts',(-9.55892369366837,2.07765116626913,-3.56464372425638));
#40891=CARTESIAN_POINT('Ctrl Pts',(-9.52787035537066,2.96953538582417,-3.27882544829067));
#40892=CARTESIAN_POINT('Ctrl Pts',(-9.51242486744516,3.38385830951819,-3.04814548837884));
#40893=CARTESIAN_POINT('Ctrl Pts',(-9.48097741353986,4.10346141477696,-2.43059522198876));
#40894=CARTESIAN_POINT('Ctrl Pts',(-9.46536142053563,4.40161797675756,-2.05390441834288));
#40895=CARTESIAN_POINT('Ctrl Pts',(-9.43189298349869,4.86216345247558,-1.15659791290247));
#40896=CARTESIAN_POINT('Ctrl Pts',(-9.41659441817477,4.96178934307193,-0.696743368548196));
#40897=CARTESIAN_POINT('Ctrl Pts',(-9.38786764570381,5.03484896790173,0.166880112239431));
#40898=CARTESIAN_POINT('Ctrl Pts',(-9.37206555359201,4.98265954300592,0.650116766645498));
#40899=CARTESIAN_POINT('Ctrl Pts',(-9.34131730068819,4.69884143765681,1.53172977266874));
#40900=CARTESIAN_POINT('Ctrl Pts',(-9.32640535038695,4.47756052459509,1.93228316468901));
#40901=CARTESIAN_POINT('Ctrl Pts',(-9.29859919994251,3.94631120018363,2.58165267968722));
#40902=CARTESIAN_POINT('Ctrl Pts',(-9.28293979780336,3.59675071557947,2.91391088646799));
#40903=CARTESIAN_POINT('Ctrl Pts',(-9.2492821143784,2.70140947631694,3.39023797385853));
#40904=CARTESIAN_POINT('Ctrl Pts',(-9.23400044723609,2.25221665077595,3.52751529061053));
#40905=CARTESIAN_POINT('Ctrl Pts',(-9.20295271590245,1.32141604787522,3.62974369515122));
#40906=CARTESIAN_POINT('Ctrl Pts',(-9.18751045174112,0.849150821771942,
3.58784773144756));
#40907=CARTESIAN_POINT('Ctrl Pts',(-9.15606524728236,-0.0595587589118044,
3.31694181014979));
#40908=CARTESIAN_POINT('Ctrl Pts',(-9.14044873203119,-0.485334243919505,
3.09434306772639));
#40909=CARTESIAN_POINT('Ctrl Pts',(-9.10798160501358,-1.24795377417342,
2.48157205297963));
#40910=CARTESIAN_POINT('Ctrl Pts',(-9.09343435231503,-1.51787189169958,
2.12625850253129));
#40911=CARTESIAN_POINT('Ctrl Pts',(-9.08091840173459,-1.70608413170262,
1.79907461418022));
#40912=CARTESIAN_POINT('',(-9.36905988923136,-1.70769139850482,1.79999996826055));
#40913=CARTESIAN_POINT('',(-9.369059892324,-1.707691453624,1.8));
#40914=CARTESIAN_POINT('Ctrl Pts',(-11.8690815026286,4.52608269350975,1.79907711429981));
#40915=CARTESIAN_POINT('Ctrl Pts',(-11.856564880409,4.3378600965681,2.12627841043079));
#40916=CARTESIAN_POINT('Ctrl Pts',(-11.8420179011084,4.06794217344854,2.48158137425679));
#40917=CARTESIAN_POINT('Ctrl Pts',(-11.8095512679702,3.30533424391916,3.09434306772659));
#40918=CARTESIAN_POINT('Ctrl Pts',(-11.7939347527189,2.87955875891145,3.31694181014995));
#40919=CARTESIAN_POINT('Ctrl Pts',(-11.7624895482601,1.97084917822778,3.58784773144761));
#40920=CARTESIAN_POINT('Ctrl Pts',(-11.7470472840988,1.49858395212459,3.62974369515122));
#40921=CARTESIAN_POINT('Ctrl Pts',(-11.7159995527651,0.567783349223929,
3.52751529061047));
#40922=CARTESIAN_POINT('Ctrl Pts',(-11.7007178856228,0.118590523682957,
3.39023797385841));
#40923=CARTESIAN_POINT('Ctrl Pts',(-11.6670602021978,-0.776750715579682,
2.91391088646765));
#40924=CARTESIAN_POINT('Ctrl Pts',(-11.6514008000586,-1.12631120018392,
2.58165267968671));
#40925=CARTESIAN_POINT('Ctrl Pts',(-11.6235946496142,-1.65756052459529,
1.93228316468843));
#40926=CARTESIAN_POINT('Ctrl Pts',(-11.608682699313,-1.87884143765697,1.53172977266818));
#40927=CARTESIAN_POINT('Ctrl Pts',(-11.5779344464092,-2.16265954300595,
0.65011676664506));
#40928=CARTESIAN_POINT('Ctrl Pts',(-11.5621323542974,-2.21484896790171,
0.166880112239127));
#40929=CARTESIAN_POINT('Ctrl Pts',(-11.5334055818265,-2.14178934307187,
-0.696743368548371));
#40930=CARTESIAN_POINT('Ctrl Pts',(-11.5181070165025,-2.04216345247547,
-1.1565979129026));
#40931=CARTESIAN_POINT('Ctrl Pts',(-11.4846385794655,-1.58161797675724,
-2.05390441834312));
#40932=CARTESIAN_POINT('Ctrl Pts',(-11.4690225864612,-1.28346141477642,
-2.43059522198911));
#40933=CARTESIAN_POINT('Ctrl Pts',(-11.4375751325559,-0.563858309517446,
-3.04814548837911));
#40934=CARTESIAN_POINT('Ctrl Pts',(-11.4221296446305,-0.149535385823461,
-3.27882544829088));
#40935=CARTESIAN_POINT('Ctrl Pts',(-11.3910763063328,0.742348833731382,
-3.56464372425646));
#40936=CARTESIAN_POINT('Ctrl Pts',(-11.3757930340538,1.20855364600227,-3.62224850779717));
#40937=CARTESIAN_POINT('Ctrl Pts',(-11.3421421920168,2.22006102775741,-3.55194694257004));
#40938=CARTESIAN_POINT('Ctrl Pts',(-11.3264872853748,2.67453375101345,-3.39102207324724));
#40939=CARTESIAN_POINT('Ctrl Pts',(-11.2986752283443,3.42438260732584,-3.0142815257501));
#40940=CARTESIAN_POINT('Ctrl Pts',(-11.2837666105191,3.78954524063164,-2.73864661536387));
#40941=CARTESIAN_POINT('Ctrl Pts',(-11.2530237479584,4.40784438986543,-2.04929227481183));
#40942=CARTESIAN_POINT('Ctrl Pts',(-11.2372209014099,4.65238613785367,-1.62921992321605));
#40943=CARTESIAN_POINT('Ctrl Pts',(-11.2085015135848,4.93742752730497,-0.810959839651302));
#40944=CARTESIAN_POINT('Ctrl Pts',(-11.1932037723418,5.0338584634379,-0.350448986549234));
#40945=CARTESIAN_POINT('Ctrl Pts',(-11.1597333887686,4.97891930544053,0.65669905610851));
#40946=CARTESIAN_POINT('Ctrl Pts',(-11.1441153325397,4.86008836875808,1.12224707164084));
#40947=CARTESIAN_POINT('Ctrl Pts',(-11.1126688297072,4.45453566345955,1.97938216415777));
#40948=CARTESIAN_POINT('Ctrl Pts',(-11.0972263091744,4.17024380133706,2.35881196450515));
#40949=CARTESIAN_POINT('Ctrl Pts',(-11.0661695800737,3.47214510051836,2.98330370028508));
#40950=CARTESIAN_POINT('Ctrl Pts',(-11.0508833417141,3.06977273055838,3.22589817344446));
#40951=CARTESIAN_POINT('Ctrl Pts',(-11.0172359909979,2.11747273302226,3.57376459988511));
#40952=CARTESIAN_POINT('Ctrl Pts',(-11.0015844822151,1.6369862302272,3.61203190002299));
#40953=CARTESIAN_POINT('Ctrl Pts',(-10.973766712292,0.798531261064747,3.57346703035343));
#40954=CARTESIAN_POINT('Ctrl Pts',(-10.9588622495894,0.352879643376049,
3.47053387849982));
#40955=CARTESIAN_POINT('Ctrl Pts',(-10.9281257943826,-0.492512987916658,
3.09309930974022));
#40956=CARTESIAN_POINT('Ctrl Pts',(-10.9123220689698,-0.88702596996958,
2.80911965889159));
#40957=CARTESIAN_POINT('Ctrl Pts',(-10.8836106328322,-1.48059838918455,
2.17820084892423));
#40958=CARTESIAN_POINT('Ctrl Pts',(-10.8683139711136,-1.7563637913354,1.79702582464458));
#40959=CARTESIAN_POINT('Ctrl Pts',(-10.8348419287415,-2.11671818989919,
0.854902102534729));
#40960=CARTESIAN_POINT('Ctrl Pts',(-10.8192215365103,-2.1979371541246,0.381267556022032));
#40961=CARTESIAN_POINT('Ctrl Pts',(-10.7877761342445,-2.17689468407348,
-0.566708949154515));
#40962=CARTESIAN_POINT('Ctrl Pts',(-10.7723369845255,-2.07199190034993,
-1.02896894674));
#40963=CARTESIAN_POINT('Ctrl Pts',(-10.7412763822331,-1.68898571587989,
-1.88386424768359));
#40964=CARTESIAN_POINT('Ctrl Pts',(-10.7259867588952,-1.42033608863858,
-2.26946266636308));
#40965=CARTESIAN_POINT('Ctrl Pts',(-10.6923430125769,-0.692530601496336,
-2.97513752621574));
#40966=CARTESIAN_POINT('Ctrl Pts',(-10.6766953355268,-0.269500817280127,
-3.20590346729835));
#40967=CARTESIAN_POINT('Ctrl Pts',(-10.6488714338812,0.512062543121538,
-3.51243382004678));
#40968=CARTESIAN_POINT('Ctrl Pts',(-10.6339717564456,0.960835502840229,
-3.6));
#40969=CARTESIAN_POINT('Ctrl Pts',(-10.6041480281948,1.85916449715974,-3.6));
#40970=CARTESIAN_POINT('Ctrl Pts',(-10.5892483507698,2.30793745687843,-3.51243382004679));
#40971=CARTESIAN_POINT('Ctrl Pts',(-10.561424449124,3.0895008172801,-3.20590346729836));
#40972=CARTESIAN_POINT('Ctrl Pts',(-10.5457767720737,3.51253060149632,-2.97513752621576));
#40973=CARTESIAN_POINT('Ctrl Pts',(-10.5121330257553,4.24033608863857,-2.26946266636309));
#40974=CARTESIAN_POINT('Ctrl Pts',(-10.4968434024174,4.50898571587988,-1.8838642476836));
#40975=CARTESIAN_POINT('Ctrl Pts',(-10.465782800125,4.89199190034993,-1.02896894674001));
#40976=CARTESIAN_POINT('Ctrl Pts',(-10.4503436504061,4.99689468407348,-0.566708949154526));
#40977=CARTESIAN_POINT('Ctrl Pts',(-10.4188982481402,5.01793715412459,0.381267556022008));
#40978=CARTESIAN_POINT('Ctrl Pts',(-10.403277855909,4.93671818989919,0.854902102534692));
#40979=CARTESIAN_POINT('Ctrl Pts',(-10.3698058135368,4.57636379133541,1.7970258246445));
#40980=CARTESIAN_POINT('Ctrl Pts',(-10.3545091518181,4.30059838918456,2.17820084892412));
#40981=CARTESIAN_POINT('Ctrl Pts',(-10.3257977156805,3.70702596996959,2.80911965889151));
#40982=CARTESIAN_POINT('Ctrl Pts',(-10.3099939902678,3.31251298791663,3.09309930974019));
#40983=CARTESIAN_POINT('Ctrl Pts',(-10.2792575350611,2.4671203566239,3.47053387849984));
#40984=CARTESIAN_POINT('Ctrl Pts',(-10.2643530723587,2.02146873893524,3.57346703035346));
#40985=CARTESIAN_POINT('Ctrl Pts',(-10.2365353024357,1.18301376977281,3.61203190002298));
#40986=CARTESIAN_POINT('Ctrl Pts',(-10.2208837936531,0.702527266977845,
3.57376459988506));
#40987=CARTESIAN_POINT('Ctrl Pts',(-10.1872364429371,-0.249772730558337,
3.22589817344435));
#40988=CARTESIAN_POINT('Ctrl Pts',(-10.1719502045775,-0.652145100518445,
2.98330370028487));
#40989=CARTESIAN_POINT('Ctrl Pts',(-10.1408934754768,-1.35024380133728,
2.35881196450477));
#40990=CARTESIAN_POINT('Ctrl Pts',(-10.125450954944,-1.63453566345979,1.97938216415733));
#40991=CARTESIAN_POINT('Ctrl Pts',(-10.0940044521113,-2.04008836875823,
1.12224707164033));
#40992=CARTESIAN_POINT('Ctrl Pts',(-10.0783863958821,-2.1589193054406,0.656699056108066));
#40993=CARTESIAN_POINT('Ctrl Pts',(-10.0449160123088,-2.21385846343786,
-0.350448986549575));
#40994=CARTESIAN_POINT('Ctrl Pts',(-10.0296182710657,-2.11742752730489,
-0.810959839651615));
#40995=CARTESIAN_POINT('Ctrl Pts',(-10.0008988832406,-1.83238613785353,
-1.62921992321635));
#40996=CARTESIAN_POINT('Ctrl Pts',(-9.9850960366923,-1.58784438986525,-2.04929227481215));
#40997=CARTESIAN_POINT('Ctrl Pts',(-9.95435317413131,-0.969545240631397,
-2.73864661536417));
#40998=CARTESIAN_POINT('Ctrl Pts',(-9.93944455630554,-0.604382607325591,
-3.01428152575038));
#40999=CARTESIAN_POINT('Ctrl Pts',(-9.91163249927465,0.14546624898688,-3.39102207324745));
#41000=CARTESIAN_POINT('Ctrl Pts',(-9.89597759263216,0.599938972242873,
-3.55194694257014));
#41001=CARTESIAN_POINT('Ctrl Pts',(-9.86232675059507,1.61144635399815,-3.62224850779715));
#41002=CARTESIAN_POINT('Ctrl Pts',(-9.84704347831627,2.07765116626922,-3.56464372425636));
#41003=CARTESIAN_POINT('Ctrl Pts',(-9.81599014001884,2.96953538582425,-3.27882544829063));
#41004=CARTESIAN_POINT('Ctrl Pts',(-9.80054465209373,3.38385830951826,-3.04814548837879));
#41005=CARTESIAN_POINT('Ctrl Pts',(-9.76909719818853,4.10346141477701,-2.4305952219887));
#41006=CARTESIAN_POINT('Ctrl Pts',(-9.75348120518421,4.40161797675761,-2.05390441834282));
#41007=CARTESIAN_POINT('Ctrl Pts',(-9.72001276814728,4.86216345247561,-1.1565979129024));
#41008=CARTESIAN_POINT('Ctrl Pts',(-9.70471420282341,4.96178934307195,-0.696743368548125));
#41009=CARTESIAN_POINT('Ctrl Pts',(-9.67598743035251,5.03484896790172,0.1668801122395));
#41010=CARTESIAN_POINT('Ctrl Pts',(-9.66018533824078,4.98265954300591,0.650116766645566));
#41011=CARTESIAN_POINT('Ctrl Pts',(-9.6294370853368,4.69884143765678,1.5317297726688));
#41012=CARTESIAN_POINT('Ctrl Pts',(-9.6145251350353,4.47756052459505,1.93228316468907));
#41013=CARTESIAN_POINT('Ctrl Pts',(-9.58671898459069,3.94631120018358,2.58165267968727));
#41014=CARTESIAN_POINT('Ctrl Pts',(-9.5710595824514,3.59675071557941,2.91391088646803));
#41015=CARTESIAN_POINT('Ctrl Pts',(-9.53740189902645,2.70140947631686,3.39023797385856));
#41016=CARTESIAN_POINT('Ctrl Pts',(-9.52212023188427,2.25221665077588,3.52751529061055));
#41017=CARTESIAN_POINT('Ctrl Pts',(-9.49107250055062,1.32141604787514,3.62974369515122));
#41018=CARTESIAN_POINT('Ctrl Pts',(-9.47563023638925,0.849150821771872,
3.58784773144755));
#41019=CARTESIAN_POINT('Ctrl Pts',(-9.44418503193039,-0.0595587589118644,
3.31694181014976));
#41020=CARTESIAN_POINT('Ctrl Pts',(-9.42856851667912,-0.485334243919561,
3.09434306772636));
#41021=CARTESIAN_POINT('Ctrl Pts',(-9.39610138755524,-1.24795382365235,
2.48157201322289));
#41022=CARTESIAN_POINT('Ctrl Pts',(-9.38155413329044,-1.51787195955029,
2.12625841386456));
#41023=CARTESIAN_POINT('Ctrl Pts',(-9.36903818168777,-1.70608420231175,
1.79907449143491));
#41024=CARTESIAN_POINT('Ctrl Pts',(-12.17488944963,5.430961212849,0.4226200533094));
#41025=CARTESIAN_POINT('Ctrl Pts',(-12.14780611629,5.335071764451,1.334947212679));
#41026=CARTESIAN_POINT('Ctrl Pts',(-12.09363944963,4.49838171004,3.087792066179));
#41027=CARTESIAN_POINT('Ctrl Pts',(-12.01238944963,1.86651847134,4.343769052512));
#41028=CARTESIAN_POINT('Ctrl Pts',(-11.93113944963,-0.9687352755443,3.662899000864));
#41029=CARTESIAN_POINT('Ctrl Pts',(-11.84988944963,-2.743789860399,1.349658053758));
#41030=CARTESIAN_POINT('Ctrl Pts',(-11.76863944963,-2.667460761666,-1.565193402042));
#41031=CARTESIAN_POINT('Ctrl Pts',(-11.68738944963,-0.7737760730864,-3.782410239809));
#41032=CARTESIAN_POINT('Ctrl Pts',(-11.60613944963,2.093235680042,-4.313780376177));
#41033=CARTESIAN_POINT('Ctrl Pts',(-11.52488944963,4.655723656744,-2.922462659301));
#41034=CARTESIAN_POINT('Ctrl Pts',(-11.44363944963,5.771566414534,-0.2285800240809));
#41035=CARTESIAN_POINT('Ctrl Pts',(-11.36238944963,4.943423784343,2.56718265288));
#41036=CARTESIAN_POINT('Ctrl Pts',(-11.28113944963,2.540405635919,4.218731264996));
#41037=CARTESIAN_POINT('Ctrl Pts',(-11.19988944963,-0.3664434354111,3.989957282902));
#41038=CARTESIAN_POINT('Ctrl Pts',(-11.11863944963,-2.481517318933,1.982827111076));
#41039=CARTESIAN_POINT('Ctrl Pts',(-11.03738944963,-2.862110501329,-0.9080651192168));
#41040=CARTESIAN_POINT('Ctrl Pts',(-10.95613944963,-1.338589527067,-3.394225391463));
#41041=CARTESIAN_POINT('Ctrl Pts',(-10.87488944963,1.41,-4.367551991253));
#41042=CARTESIAN_POINT('Ctrl Pts',(-10.79363944963,4.158589527067,-3.394225391463));
#41043=CARTESIAN_POINT('Ctrl Pts',(-10.71238944963,5.682110501329,-0.9080651192168));
#41044=CARTESIAN_POINT('Ctrl Pts',(-10.63113944963,5.301517318933,1.982827111076));
#41045=CARTESIAN_POINT('Ctrl Pts',(-10.54988944963,3.186443435411,3.989957282902));
#41046=CARTESIAN_POINT('Ctrl Pts',(-10.46863944963,0.2795943640806,4.218731264996));
#41047=CARTESIAN_POINT('Ctrl Pts',(-10.38738944963,-2.123423784343,2.56718265288));
#41048=CARTESIAN_POINT('Ctrl Pts',(-10.30613944963,-2.951566414534,-0.2285800240809));
#41049=CARTESIAN_POINT('Ctrl Pts',(-10.22488944963,-1.835723656744,-2.922462659301));
#41050=CARTESIAN_POINT('Ctrl Pts',(-10.14363944963,0.7267643199575,-4.313780376177));
#41051=CARTESIAN_POINT('Ctrl Pts',(-10.06238944963,3.593776073086,-3.782410239809));
#41052=CARTESIAN_POINT('Ctrl Pts',(-9.981139449625,5.487460761666,-1.565193402042));
#41053=CARTESIAN_POINT('Ctrl Pts',(-9.899889449625,5.563789860399,1.349658053758));
#41054=CARTESIAN_POINT('Ctrl Pts',(-9.818639449625,3.788735275544,3.662899000864));
#41055=CARTESIAN_POINT('Ctrl Pts',(-9.737389449625,0.9534815286599,4.343769052512));
#41056=CARTESIAN_POINT('Ctrl Pts',(-9.656139449625,-1.67838171004,3.087792066179));
#41057=CARTESIAN_POINT('Ctrl Pts',(-9.601972782958,-2.515071764451,1.334947212679));
#41058=CARTESIAN_POINT('Ctrl Pts',(-9.574889449625,-2.610961212849,0.4226200533094));
#41059=CARTESIAN_POINT('Ctrl Pts',(-12.08131644732,5.269775872549,0.4056787913812));
#41060=CARTESIAN_POINT('Ctrl Pts',(-12.05423311398,5.177730274553,1.281434157126));
#41061=CARTESIAN_POINT('Ctrl Pts',(-12.00006644732,4.37458000429,2.964013997052));
#41062=CARTESIAN_POINT('Ctrl Pts',(-11.91881644732,1.848218348245,4.169643549716));
#41063=CARTESIAN_POINT('Ctrl Pts',(-11.83756644732,-0.8733806489824,3.51606703938));
#41064=CARTESIAN_POINT('Ctrl Pts',(-11.75631644732,-2.577279914956,1.295555295446));
#41065=CARTESIAN_POINT('Ctrl Pts',(-11.67506644732,-2.504010565149,-1.502450635378));
#41066=CARTESIAN_POINT('Ctrl Pts',(-11.59381644732,-0.686236633921,-3.630787518428));
#41067=CARTESIAN_POINT('Ctrl Pts',(-11.51256644732,2.06584730951,-4.140857007583));
#41068=CARTESIAN_POINT('Ctrl Pts',(-11.43131644732,4.5256146991,-2.805312029559));
#41069=CARTESIAN_POINT('Ctrl Pts',(-11.35006644732,5.596727481863,-0.2194171033222));
#41070=CARTESIAN_POINT('Ctrl Pts',(-11.26881644732,4.801782001457,2.464273873707));
#41071=CARTESIAN_POINT('Ctrl Pts',(-11.18756644732,2.495091889415,4.049618060818));
#41072=CARTESIAN_POINT('Ctrl Pts',(-11.10631644732,-0.2952324426901,3.830014774536));
#41073=CARTESIAN_POINT('Ctrl Pts',(-11.02506644732,-2.325520901626,1.903342966431));
#41074=CARTESIAN_POINT('Ctrl Pts',(-10.94381644732,-2.690857522625,-0.8716641748885));
#41075=CARTESIAN_POINT('Ctrl Pts',(-10.86256644732,-1.2284088228,-3.258163553058));
#41076=CARTESIAN_POINT('Ctrl Pts',(-10.78131644732,1.41,-4.192473119132));
#41077=CARTESIAN_POINT('Ctrl Pts',(-10.70006644732,4.0484088228,-3.258163553058));
#41078=CARTESIAN_POINT('Ctrl Pts',(-10.61881644732,5.510857522625,-0.8716641748885));
#41079=CARTESIAN_POINT('Ctrl Pts',(-10.53756644732,5.145520901626,1.903342966431));
#41080=CARTESIAN_POINT('Ctrl Pts',(-10.45631644732,3.11523244269,3.830014774536));
#41081=CARTESIAN_POINT('Ctrl Pts',(-10.37506644732,0.3249081105847,4.049618060818));
#41082=CARTESIAN_POINT('Ctrl Pts',(-10.29381644732,-1.981782001457,2.464273873707));
#41083=CARTESIAN_POINT('Ctrl Pts',(-10.21256644732,-2.776727481863,-0.2194171033222));
#41084=CARTESIAN_POINT('Ctrl Pts',(-10.13131644732,-1.7056146991,-2.805312029559));
#41085=CARTESIAN_POINT('Ctrl Pts',(-10.05006644732,0.7541526904896,-4.140857007583));
#41086=CARTESIAN_POINT('Ctrl Pts',(-9.968816447316,3.506236633921,-3.630787518428));
#41087=CARTESIAN_POINT('Ctrl Pts',(-9.887566447316,5.324010565149,-1.502450635378));
#41088=CARTESIAN_POINT('Ctrl Pts',(-9.806316447316,5.397279914956,1.295555295446));
#41089=CARTESIAN_POINT('Ctrl Pts',(-9.725066447316,3.693380648982,3.51606703938));
#41090=CARTESIAN_POINT('Ctrl Pts',(-9.643816447316,0.9717816517551,4.169643549716));
#41091=CARTESIAN_POINT('Ctrl Pts',(-9.562566447316,-1.55458000429,2.964013997052));
#41092=CARTESIAN_POINT('Ctrl Pts',(-9.50839978065,-2.357730274553,1.281434157126));
#41093=CARTESIAN_POINT('Ctrl Pts',(-9.481316447316,-2.449775872549,0.4056787913812));
#41094=CARTESIAN_POINT('Ctrl Pts',(-11.98774344501,5.10859053225,0.388737529453));
#41095=CARTESIAN_POINT('Ctrl Pts',(-11.96066011167,5.020388784654,1.227921101574));
#41096=CARTESIAN_POINT('Ctrl Pts',(-11.90649344501,4.250778298539,2.840235927925));
#41097=CARTESIAN_POINT('Ctrl Pts',(-11.82524344501,1.82991822515,3.99551804692));
#41098=CARTESIAN_POINT('Ctrl Pts',(-11.74399344501,-0.7780260224205,3.369235077895));
#41099=CARTESIAN_POINT('Ctrl Pts',(-11.66274344501,-2.410769969513,1.241452537133));
#41100=CARTESIAN_POINT('Ctrl Pts',(-11.58149344501,-2.340560368632,-1.439707868714));
#41101=CARTESIAN_POINT('Ctrl Pts',(-11.50024344501,-0.5986971947557,-3.479164797048));
#41102=CARTESIAN_POINT('Ctrl Pts',(-11.41899344501,2.038458938978,-3.967933638989));
#41103=CARTESIAN_POINT('Ctrl Pts',(-11.33774344501,4.395505741456,-2.688161399818));
#41104=CARTESIAN_POINT('Ctrl Pts',(-11.25649344501,5.421888549192,-0.2102541825635));
#41105=CARTESIAN_POINT('Ctrl Pts',(-11.17524344501,4.660140218572,2.361365094534));
#41106=CARTESIAN_POINT('Ctrl Pts',(-11.09399344501,2.449778142911,3.88050485664));
#41107=CARTESIAN_POINT('Ctrl Pts',(-11.01274344501,-0.2240214499691,3.670072266171));
#41108=CARTESIAN_POINT('Ctrl Pts',(-10.93149344501,-2.16952448432,1.823858821786));
#41109=CARTESIAN_POINT('Ctrl Pts',(-10.85024344501,-2.519604543921,-0.8352632305602));
#41110=CARTESIAN_POINT('Ctrl Pts',(-10.76899344501,-1.118228118532,-3.122101714653));
#41111=CARTESIAN_POINT('Ctrl Pts',(-10.68774344501,1.41,-4.017394247012));
#41112=CARTESIAN_POINT('Ctrl Pts',(-10.60649344501,3.938228118532,-3.122101714653));
#41113=CARTESIAN_POINT('Ctrl Pts',(-10.52524344501,5.339604543921,-0.8352632305602));
#41114=CARTESIAN_POINT('Ctrl Pts',(-10.44399344501,4.98952448432,1.823858821786));
#41115=CARTESIAN_POINT('Ctrl Pts',(-10.36274344501,3.044021449969,3.670072266171));
#41116=CARTESIAN_POINT('Ctrl Pts',(-10.28149344501,0.3702218570889,3.88050485664));
#41117=CARTESIAN_POINT('Ctrl Pts',(-10.20024344501,-1.840140218572,2.361365094534));
#41118=CARTESIAN_POINT('Ctrl Pts',(-10.11899344501,-2.601888549192,-0.2102541825635));
#41119=CARTESIAN_POINT('Ctrl Pts',(-10.03774344501,-1.575505741456,-2.688161399818));
#41120=CARTESIAN_POINT('Ctrl Pts',(-9.956493445008,0.7815410610216,-3.967933638989));
#41121=CARTESIAN_POINT('Ctrl Pts',(-9.875243445008,3.418697194756,-3.479164797048));
#41122=CARTESIAN_POINT('Ctrl Pts',(-9.793993445008,5.160560368632,-1.439707868714));
#41123=CARTESIAN_POINT('Ctrl Pts',(-9.712743445008,5.230769969513,1.241452537133));
#41124=CARTESIAN_POINT('Ctrl Pts',(-9.631493445008,3.59802602242,3.369235077895));
#41125=CARTESIAN_POINT('Ctrl Pts',(-9.550243445008,0.9900817748502,3.99551804692));
#41126=CARTESIAN_POINT('Ctrl Pts',(-9.468993445008,-1.430778298539,2.840235927925));
#41127=CARTESIAN_POINT('Ctrl Pts',(-9.414826778341,-2.200388784654,1.227921101574));
#41128=CARTESIAN_POINT('Ctrl Pts',(-9.387743445008,-2.28859053225,0.388737529453));
#41129=CARTESIAN_POINT('Ctrl Pts',(-11.8941704427,4.94740519195,0.3717962675248));
#41130=CARTESIAN_POINT('Ctrl Pts',(-11.86708710937,4.863047294756,1.174408046021));
#41131=CARTESIAN_POINT('Ctrl Pts',(-11.8129204427,4.126976592789,2.716457858798));
#41132=CARTESIAN_POINT('Ctrl Pts',(-11.7316704427,1.811618102055,3.821392544123));
#41133=CARTESIAN_POINT('Ctrl Pts',(-11.6504204427,-0.6826713958586,3.22240311641));
#41134=CARTESIAN_POINT('Ctrl Pts',(-11.5691704427,-2.244260024069,1.187349778821));
#41135=CARTESIAN_POINT('Ctrl Pts',(-11.4879204427,-2.177110172115,-1.37696510205));
#41136=CARTESIAN_POINT('Ctrl Pts',(-11.4066704427,-0.5111577555903,-3.327542075668));
#41137=CARTESIAN_POINT('Ctrl Pts',(-11.3254204427,2.011070568446,-3.795010270395));
#41138=CARTESIAN_POINT('Ctrl Pts',(-11.2441704427,4.265396783812,-2.571010770076));
#41139=CARTESIAN_POINT('Ctrl Pts',(-11.1629204427,5.247049616522,-0.2010912618048));
#41140=CARTESIAN_POINT('Ctrl Pts',(-11.0816704427,4.518498435686,2.258456315361));
#41141=CARTESIAN_POINT('Ctrl Pts',(-11.0004204427,2.404464396407,3.711391652462));
#41142=CARTESIAN_POINT('Ctrl Pts',(-10.9191704427,-0.1528104572481,3.510129757805));
#41143=CARTESIAN_POINT('Ctrl Pts',(-10.8379204427,-2.013528067013,1.744374677141));
#41144=CARTESIAN_POINT('Ctrl Pts',(-10.7566704427,-2.348351565217,-0.7988622862319));
#41145=CARTESIAN_POINT('Ctrl Pts',(-10.6754204427,-1.008047414265,-2.986039876248));
#41146=CARTESIAN_POINT('Ctrl Pts',(-10.5941704427,1.41,-3.842315374891));
#41147=CARTESIAN_POINT('Ctrl Pts',(-10.5129204427,3.828047414265,-2.986039876248));
#41148=CARTESIAN_POINT('Ctrl Pts',(-10.4316704427,5.168351565217,-0.7988622862319));
#41149=CARTESIAN_POINT('Ctrl Pts',(-10.3504204427,4.833528067013,1.744374677141));
#41150=CARTESIAN_POINT('Ctrl Pts',(-10.2691704427,2.972810457248,3.510129757805));
#41151=CARTESIAN_POINT('Ctrl Pts',(-10.1879204427,0.4155356035931,3.711391652462));
#41152=CARTESIAN_POINT('Ctrl Pts',(-10.1066704427,-1.698498435686,2.258456315361));
#41153=CARTESIAN_POINT('Ctrl Pts',(-10.0254204427,-2.427049616522,-0.2010912618048));
#41154=CARTESIAN_POINT('Ctrl Pts',(-9.944170442699,-1.445396783812,-2.571010770076));
#41155=CARTESIAN_POINT('Ctrl Pts',(-9.862920442699,0.8089294315536,-3.795010270395));
#41156=CARTESIAN_POINT('Ctrl Pts',(-9.781670442699,3.33115775559,-3.327542075668));
#41157=CARTESIAN_POINT('Ctrl Pts',(-9.700420442699,4.997110172115,-1.37696510205));
#41158=CARTESIAN_POINT('Ctrl Pts',(-9.619170442699,5.064260024069,1.187349778821));
#41159=CARTESIAN_POINT('Ctrl Pts',(-9.537920442699,3.502671395859,3.22240311641));
#41160=CARTESIAN_POINT('Ctrl Pts',(-9.456670442699,1.008381897945,3.821392544123));
#41161=CARTESIAN_POINT('Ctrl Pts',(-9.375420442699,-1.306976592789,2.716457858798));
#41162=CARTESIAN_POINT('Ctrl Pts',(-9.321253776032,-2.043047294756,1.174408046021));
#41163=CARTESIAN_POINT('Ctrl Pts',(-9.294170442699,-2.12740519195,0.3717962675247));
#41164=CARTESIAN_POINT('',(-9.59950292206818,-2.05335595141186,1.99956949001459));
#41165=CARTESIAN_POINT('',(-9.6,-2.054101615138,2.));
#41166=CARTESIAN_POINT('Ctrl Pts',(-9.60038389030658,-2.0529396754269,1.99929827157929));
#41167=CARTESIAN_POINT('Ctrl Pts',(-9.60356530287706,-2.00039204375156,
2.09076525956697));
#41168=CARTESIAN_POINT('Ctrl Pts',(-9.60671484827216,-1.94423773209052,
2.18016104618138));
#41169=CARTESIAN_POINT('Ctrl Pts',(-9.61408724163892,-1.80249740006208,
2.38692131089865));
#41170=CARTESIAN_POINT('Ctrl Pts',(-9.61822215610905,-1.71422667129878,
2.50151091015392));
#41171=CARTESIAN_POINT('Ctrl Pts',(-9.62752557198061,-1.50197970552175,
2.74767411679855));
#41172=CARTESIAN_POINT('Ctrl Pts',(-9.63270765290204,-1.3754430723976,2.87546943152105));
#41173=CARTESIAN_POINT('Ctrl Pts',(-9.64887550363486,-0.968293782115969,
3.23412919115236));
#41174=CARTESIAN_POINT('Ctrl Pts',(-9.66016975238785,-0.663659725799785,
3.43661940584889));
#41175=CARTESIAN_POINT('Ctrl Pts',(-9.67632979613604,-0.189542768342011,
3.66788018375336));
#41176=CARTESIAN_POINT('Ctrl Pts',(-9.68135338289722,-0.036546137152591,
3.73128585713501));
#41177=CARTESIAN_POINT('Ctrl Pts',(-9.69224736938775,0.309509670573514,
3.85011655992189));
#41178=CARTESIAN_POINT('Ctrl Pts',(-9.69797243888469,0.503018926468948,
3.90055566772882));
#41179=CARTESIAN_POINT('Ctrl Pts',(-9.70781276540716,0.84255087277572,3.96177018746316));
#41180=CARTESIAN_POINT('Ctrl Pts',(-9.71194276219778,0.985825172191182,
3.97951488629265));
#41181=CARTESIAN_POINT('Ctrl Pts',(-9.72745568668193,1.5114670143326,4.01533129444717));
#41182=CARTESIAN_POINT('Ctrl Pts',(-9.73934444916767,1.89643369774521,3.98611924326558));
#41183=CARTESIAN_POINT('Ctrl Pts',(-9.75634099757543,2.43748806067625,3.86761301664057));
#41184=CARTESIAN_POINT('Ctrl Pts',(-9.76158382277774,2.60314950883664,3.82015904654046));
#41185=CARTESIAN_POINT('Ctrl Pts',(-9.77264780072068,2.95189040385358,3.69541703711582));
#41186=CARTESIAN_POINT('Ctrl Pts',(-9.77834886504983,3.13279319787768,3.61499425675465));
#41187=CARTESIAN_POINT('Ctrl Pts',(-9.78809948113757,3.43332706222437,3.4530480553865));
#41188=CARTESIAN_POINT('Ctrl Pts',(-9.79217582267793,3.55518422433439,3.37855139482717));
#41189=CARTESIAN_POINT('Ctrl Pts',(-9.80867298776108,4.01774454336137,3.05977039466347));
#41190=CARTESIAN_POINT('Ctrl Pts',(-9.82175163310386,4.32467416430134,2.76746153256514));
#41191=CARTESIAN_POINT('Ctrl Pts',(-9.83955881259253,4.67970399945409,2.30675385449881));
#41192=CARTESIAN_POINT('Ctrl Pts',(-9.84451574946329,4.77155439973838,2.17143332655518));
#41193=CARTESIAN_POINT('Ctrl Pts',(-9.85484351938631,4.94853306828867,1.87275013717391));
#41194=CARTESIAN_POINT('Ctrl Pts',(-9.86011041467817,5.03082291373801,1.70886404923415));
#41195=CARTESIAN_POINT('Ctrl Pts',(-9.86943108170336,5.15647050662968,1.40756122410476));
#41196=CARTESIAN_POINT('Ctrl Pts',(-9.87349827715893,5.2040919766527,1.27325096319659));
#41197=CARTESIAN_POINT('Ctrl Pts',(-9.88997934009062,5.36250385534211,0.734865045393361));
#41198=CARTESIAN_POINT('Ctrl Pts',(-9.90305133392686,5.41686001613788,0.31476452742291));
#41199=CARTESIAN_POINT('Ctrl Pts',(-9.92084546501746,5.40263864746328,-0.266266922728023));
#41200=CARTESIAN_POINT('Ctrl Pts',(-9.92579666794673,5.38882790792707,-0.429042738008711));
#41201=CARTESIAN_POINT('Ctrl Pts',(-9.93610600141257,5.33841054894495,-0.771919576338839));
#41202=CARTESIAN_POINT('Ctrl Pts',(-9.94136091884868,5.29930430288804,-0.950648946963678));
#41203=CARTESIAN_POINT('Ctrl Pts',(-9.95067177282764,5.20746617111596,-1.26354440945371));
#41204=CARTESIAN_POINT('Ctrl Pts',(-9.9547410020691,5.159936242499,-1.39796426332582));
#41205=CARTESIAN_POINT('Ctrl Pts',(-9.97122325667245,4.94423427933181,-1.91611054506857));
#41206=CARTESIAN_POINT('Ctrl Pts',(-9.98429397417252,4.72213490688853,-2.27678351108641));
#41207=CARTESIAN_POINT('Ctrl Pts',(-10.0020887433787,4.34544430186493,-2.71941947935478));
#41208=CARTESIAN_POINT('Ctrl Pts',(-10.0070414655184,4.2322450932266,-2.83726924033038));
#41209=CARTESIAN_POINT('Ctrl Pts',(-10.0173533129096,3.97723159744509,-3.07206834503773));
#41210=CARTESIAN_POINT('Ctrl Pts',(-10.0226092318958,3.83433887046246,-3.18637976934664));
#41211=CARTESIAN_POINT('Ctrl Pts',(-10.031921004753,3.5660324141649,-3.37176777016096));
#41212=CARTESIAN_POINT('Ctrl Pts',(-10.0359901742059,3.44450475238576,-3.44631916963979));
#41213=CARTESIAN_POINT('Ctrl Pts',(-10.0524713276702,2.95083066874372,-3.71323316974167));
#41214=CARTESIAN_POINT('Ctrl Pts',(-10.0655408566307,2.55128780158735,-3.85375264974307));
#41215=CARTESIAN_POINT('Ctrl Pts',(-10.0833348409095,1.9800155071088,-3.9607014925102));
#41216=CARTESIAN_POINT('Ctrl Pts',(-10.0882878803586,1.8178689752247,-3.98105582710122));
#41217=CARTESIAN_POINT('Ctrl Pts',(-10.0986028994856,1.47181841038385,-4.00306053216985));
#41218=CARTESIAN_POINT('Ctrl Pts',(-10.1038614457517,1.28873662241507,-4.00197013253393));
#41219=CARTESIAN_POINT('Ctrl Pts',(-10.1131761742988,0.963450536031142,
-3.97717099590949));
#41220=CARTESIAN_POINT('Ctrl Pts',(-10.1172456861664,0.822079760251391,
-3.95862047716695));
#41221=CARTESIAN_POINT('Ctrl Pts',(-10.1337210833123,0.270654828968657,
-3.85538213337134));
#41222=CARTESIAN_POINT('Ctrl Pts',(-10.1467835422855,-0.12807379225162,
-3.71323318192157));
#41223=CARTESIAN_POINT('Ctrl Pts',(-10.1645727398934,-0.639225617322842,
-3.43696945479779));
#41224=CARTESIAN_POINT('Ctrl Pts',(-10.1695274186164,-0.778097028999871,
-3.35073195043681));
#41225=CARTESIAN_POINT('Ctrl Pts',(-10.1798510443381,-1.06112010795561,
-3.14991508542845));
#41226=CARTESIAN_POINT('Ctrl Pts',(-10.1851160499579,-1.20289109057113,
-3.03370354506004));
#41227=CARTESIAN_POINT('Ctrl Pts',(-10.1944386818381,-1.44025798266449,
-2.80950825991934));
#41228=CARTESIAN_POINT('Ctrl Pts',(-10.1985096791852,-1.53846870358844,
-2.70607957564346));
#41229=CARTESIAN_POINT('Ctrl Pts',(-10.2149660765781,-1.901540294255,-2.27929208182364));
#41230=CARTESIAN_POINT('Ctrl Pts',(-10.2280047461702,-2.12161193747308,
-1.91856587848559));
#41231=CARTESIAN_POINT('Ctrl Pts',(-10.2457782540083,-2.34500085639878,
-1.38278262607149));
#41232=CARTESIAN_POINT('Ctrl Pts',(-10.2507388319314,-2.39876523335634,
-1.22821628666278));
#41233=CARTESIAN_POINT('Ctrl Pts',(-10.2610940638057,-2.49270795668494,
-0.893073927079879));
#41234=CARTESIAN_POINT('Ctrl Pts',(-10.2663828896523,-2.52991411400295,
-0.712710153376773));
#41235=CARTESIAN_POINT('Ctrl Pts',(-10.2757342916575,-2.57330753149533,
-0.388081751887753));
#41236=CARTESIAN_POINT('Ctrl Pts',(-10.2798103901135,-2.58449302881199,
-0.245736061020243));
#41237=CARTESIAN_POINT('Ctrl Pts',(-10.2961990259462,-2.59773794386555,
0.31202360398641));
#41238=CARTESIAN_POINT('Ctrl Pts',(-10.3091532014495,-2.5423095309823,0.728235535351825));
#41239=CARTESIAN_POINT('Ctrl Pts',(-10.3268709512183,-2.3800745075292,1.28358089222998));
#41240=CARTESIAN_POINT('Ctrl Pts',(-10.331852549475,-2.32455286622402,1.43821007369828));
#41241=CARTESIAN_POINT('Ctrl Pts',(-10.3423194746549,-2.18552130886872,
1.76126220786652));
#41242=CARTESIAN_POINT('Ctrl Pts',(-10.3476922445167,-2.09953324990513,
1.92748599744783));
#41243=CARTESIAN_POINT('Ctrl Pts',(-10.3571458922523,-1.92672997818416,
2.20991504740668));
#41244=CARTESIAN_POINT('Ctrl Pts',(-10.3612408013389,-1.84533486327226,
2.32792924036541));
#41245=CARTESIAN_POINT('Ctrl Pts',(-10.3773779107013,-1.50932128266654,
2.76207457284958));
#41246=CARTESIAN_POINT('Ctrl Pts',(-10.3900198521859,-1.21201226449631,
3.04441768316098));
#41247=CARTESIAN_POINT('Ctrl Pts',(-10.4075335128801,-0.743988086270147,
3.37240036674797));
#41248=CARTESIAN_POINT('Ctrl Pts',(-10.4125957843033,-0.601796957317238,
3.4595532256687));
#41249=CARTESIAN_POINT('Ctrl Pts',(-10.4234767888686,-0.279127871830285,
3.63054871401733));
#41250=CARTESIAN_POINT('Ctrl Pts',(-10.429157275838,-0.0976044409438953,
3.70992203602593));
#41251=CARTESIAN_POINT('Ctrl Pts',(-10.4389963500317,0.227674526330999,
3.82363980065691));
#41252=CARTESIAN_POINT('Ctrl Pts',(-10.4431705301241,0.367777254335285,
3.86402210570016));
#41253=CARTESIAN_POINT('Ctrl Pts',(-10.4582004139136,0.864978434099937,
3.97776706276133));
#41254=CARTESIAN_POINT('Ctrl Pts',(-10.4694924955657,1.23080414723719,4.01002125222356));
#41255=CARTESIAN_POINT('Ctrl Pts',(-10.4871409462028,1.80472053537462,3.98404612758533));
#41256=CARTESIAN_POINT('Ctrl Pts',(-10.493577465914,2.01464812178365,3.95814054182262));
#41257=CARTESIAN_POINT('Ctrl Pts',(-10.5045000912726,2.37481293781915,3.88433901412407));
#41258=CARTESIAN_POINT('Ctrl Pts',(-10.5090183740214,2.52595482119583,3.84390308541401));
#41259=CARTESIAN_POINT('Ctrl Pts',(-10.5166111392828,2.77801443806076,3.75997974605779));
#41260=CARTESIAN_POINT('Ctrl Pts',(-10.5197090386381,2.87987189669372,3.72129811497914));
#41261=CARTESIAN_POINT('Ctrl Pts',(-10.5277070283744,3.13450631164313,3.61227739170519));
#41262=CARTESIAN_POINT('Ctrl Pts',(-10.5326867226591,3.28450323417034,3.5362650427459));
#41263=CARTESIAN_POINT('Ctrl Pts',(-10.5440435692485,3.6088581575327,3.34557807293149));
#41264=CARTESIAN_POINT('Ctrl Pts',(-10.5504678209985,3.7804766845146,3.22585319720809));
#41265=CARTESIAN_POINT('Ctrl Pts',(-10.5655939875803,4.16088617150598,2.91459262974356));
#41266=CARTESIAN_POINT('Ctrl Pts',(-10.5742932160297,4.36131384990957,2.71250670110083));
#41267=CARTESIAN_POINT('Ctrl Pts',(-10.5870541477555,4.63087356683859,2.37551237534754));
#41268=CARTESIAN_POINT('Ctrl Pts',(-10.5913105589387,4.71670929439931,2.25483510527093));
#41269=CARTESIAN_POINT('Ctrl Pts',(-10.6020163495018,4.91630961176043,1.93759246460366));
#41270=CARTESIAN_POINT('Ctrl Pts',(-10.6084882172266,5.01965141413363,1.73663506835275));
#41271=CARTESIAN_POINT('Ctrl Pts',(-10.6205587464262,5.17287461575667,1.3634604433922));
#41272=CARTESIAN_POINT('Ctrl Pts',(-10.6259588258771,5.22918660095898,1.19541593695418));
#41273=CARTESIAN_POINT('Ctrl Pts',(-10.6423653971073,5.36562042592812,0.678895814094211));
#41274=CARTESIAN_POINT('Ctrl Pts',(-10.6534679352852,5.41143141899804,0.321003183428782));
#41275=CARTESIAN_POINT('Ctrl Pts',(-10.6684083871825,5.40786865333887,-0.184422482507212));
#41276=CARTESIAN_POINT('Ctrl Pts',(-10.6726466517092,5.39854196104777,-0.331641454778599));
#41277=CARTESIAN_POINT('Ctrl Pts',(-10.6832935495075,5.35402793405433,-0.701737652690854));
#41278=CARTESIAN_POINT('Ctrl Pts',(-10.689724630813,5.30815987282224,-0.921509015215272));
#41279=CARTESIAN_POINT('Ctrl Pts',(-10.7017378455914,5.19311101656967,-1.30622602262263));
#41280=CARTESIAN_POINT('Ctrl Pts',(-10.7071253608828,5.13135976370246,-1.47193389142936));
#41281=CARTESIAN_POINT('Ctrl Pts',(-10.7235583995194,4.91233815883653,-1.96019232383478));
#41282=CARTESIAN_POINT('Ctrl Pts',(-10.7347025093434,4.72210818287561,-2.26833649793867));
#41283=CARTESIAN_POINT('Ctrl Pts',(-10.749676954179,4.40044025166506,-2.65973903608302));
#41284=CARTESIAN_POINT('Ctrl Pts',(-10.7539120496034,4.30059582846155,-2.76819109251104));
#41285=CARTESIAN_POINT('Ctrl Pts',(-10.7645484338315,4.03332647440469,-3.02751190420293));
#41286=CARTESIAN_POINT('Ctrl Pts',(-10.7709721639332,3.85957691637718,-3.16927194024045));
#41287=CARTESIAN_POINT('Ctrl Pts',(-10.7829750644081,3.52835270750287,-3.39569146699147));
#41288=CARTESIAN_POINT('Ctrl Pts',(-10.7883603277257,3.37614985856842,-3.48559111068736));
#41289=CARTESIAN_POINT('Ctrl Pts',(-10.8047979820205,2.89856072894582,-3.72734106315919));
#41290=CARTESIAN_POINT('Ctrl Pts',(-10.8159494144163,2.55659015861143,-3.84719422135782));
#41291=CARTESIAN_POINT('Ctrl Pts',(-10.8309298036846,2.06008374208132,-3.94896588298085));
#41292=CARTESIAN_POINT('Ctrl Pts',(-10.8351643065083,1.91425722535568,-3.97040873696884));
#41293=CARTESIAN_POINT('Ctrl Pts',(-10.845799102281,1.54340786781898,-4.00373022752363));
#41294=CARTESIAN_POINT('Ctrl Pts',(-10.8522218321573,1.31920204806696,-4.00455379063362));
#41295=CARTESIAN_POINT('Ctrl Pts',(-10.86422325653,0.919348748111904,-3.97207705536693));
#41296=CARTESIAN_POINT('Ctrl Pts',(-10.8696081359326,0.744500468340475,
-3.94616230546156));
#41297=CARTESIAN_POINT('Ctrl Pts',(-10.8860469497402,0.221165463968839,
-3.83348293218832));
#41298=CARTESIAN_POINT('Ctrl Pts',(-10.8972000195863,-0.120070896657474,
-3.71140022738352));
#41299=CARTESIAN_POINT('Ctrl Pts',(-10.9121818333282,-0.570015541435581,
-3.47799933620615));
#41300=CARTESIAN_POINT('Ctrl Pts',(-10.9164162819486,-0.696835886350252,
-3.40289049026002));
#41301=CARTESIAN_POINT('Ctrl Pts',(-10.9270500962871,-1.00597629144814,
-3.1954181329681));
#41302=CARTESIAN_POINT('Ctrl Pts',(-10.933471910365,-1.18070770031624,-3.05498200480715));
#41303=CARTESIAN_POINT('Ctrl Pts',(-10.9454724639931,-1.47099500267918,
-2.77813020528333));
#41304=CARTESIAN_POINT('Ctrl Pts',(-10.9508575091326,-1.59057346493261,
-2.64795208549007));
#41305=CARTESIAN_POINT('Ctrl Pts',(-10.9672957226068,-1.92635978655342,
-2.23105522557671));
#41306=CARTESIAN_POINT('Ctrl Pts',(-10.9784479704523,-2.11471224113583,
-1.92145639935711));
#41307=CARTESIAN_POINT('Ctrl Pts',(-10.9934292463538,-2.31750461921738,
-1.45693204652551));
#41308=CARTESIAN_POINT('Ctrl Pts',(-10.9976638817805,-2.36880024259132,
-1.31874592294464));
#41309=CARTESIAN_POINT('Ctrl Pts',(-11.0082978931886,-2.47849044690317,
-0.962954122100787));
#41310=CARTESIAN_POINT('Ctrl Pts',(-11.0147196930115,-2.52590757199542,
-0.743850529451884));
#41311=CARTESIAN_POINT('Ctrl Pts',(-11.0267188429428,-2.57727552756237,
-0.34605818607726));
#41312=CARTESIAN_POINT('Ctrl Pts',(-11.0321023801037,-2.58828479071026,
-0.169686925643484));
#41313=CARTESIAN_POINT('Ctrl Pts',(-11.0485403456435,-2.58690626763649,
0.365610443292089));
#41314=CARTESIAN_POINT('Ctrl Pts',(-11.0596940741681,-2.53845513269296,
0.724789970060807));
#41315=CARTESIAN_POINT('Ctrl Pts',(-11.0746745975932,-2.40373806791304,
1.21339296651227));
#41316=CARTESIAN_POINT('Ctrl Pts',(-11.0789074289317,-2.35666607982398,
1.35300673589102));
#41317=CARTESIAN_POINT('Ctrl Pts',(-11.0895490982095,-2.21792479375506,
1.69880872528293));
#41318=CARTESIAN_POINT('Ctrl Pts',(-11.0959803388385,-2.11672128528476,
1.89922480552137));
#41319=CARTESIAN_POINT('Ctrl Pts',(-11.1079949941462,-1.90596565912335,
2.24109766425555));
#41320=CARTESIAN_POINT('Ctrl Pts',(-11.1133839304883,-1.80338731043011,
2.38521224645819));
#41321=CARTESIAN_POINT('Ctrl Pts',(-11.1298339556531,-1.46505782436029,
2.80055387367309));
#41322=CARTESIAN_POINT('Ctrl Pts',(-11.1409940587441,-1.20110074462961,
3.04925145424864));
#41323=CARTESIAN_POINT('Ctrl Pts',(-11.1559893263683,-0.788365636720366,
3.3442816688788));
#41324=CARTESIAN_POINT('Ctrl Pts',(-11.1602297731123,-0.663644245149938,
3.42323090938001));
#41325=CARTESIAN_POINT('Ctrl Pts',(-11.1708232940868,-0.339642445151675,
3.6035615679563));
#41326=CARTESIAN_POINT('Ctrl Pts',(-11.1771992020061,-0.136755697950704,
3.69480174137272));
#41327=CARTESIAN_POINT('Ctrl Pts',(-11.1891423376604,0.23977664199463,3.82737754525561));
#41328=CARTESIAN_POINT('Ctrl Pts',(-11.1945206374603,0.40978980570469,3.87489124106396));
#41329=CARTESIAN_POINT('Ctrl Pts',(-11.2109056449069,0.931879281381264,
3.98489475412638));
#41330=CARTESIAN_POINT('Ctrl Pts',(-11.2220100452921,1.29164583404792,4.01254222052902));
#41331=CARTESIAN_POINT('Ctrl Pts',(-11.2369319057045,1.79563625227147,3.9834622357161));
#41332=CARTESIAN_POINT('Ctrl Pts',(-11.2411533761928,1.94160496329731,3.96680896786886));
#41333=CARTESIAN_POINT('Ctrl Pts',(-11.2514157657781,2.29607364367905,3.90602338247599));
#41334=CARTESIAN_POINT('Ctrl Pts',(-11.2574649232284,2.50143665498611,3.85336742407973));
#41335=CARTESIAN_POINT('Ctrl Pts',(-11.2687667488048,2.86029422951289,3.72988603275378));
#41336=CARTESIAN_POINT('Ctrl Pts',(-11.2738366549422,3.01458057559514,3.66573307315122));
#41337=CARTESIAN_POINT('Ctrl Pts',(-11.290025581993,3.48904557328449,3.43329883790693));
#41338=CARTESIAN_POINT('Ctrl Pts',(-11.3012973732444,3.79283470686785,3.2307315058391));
#41339=CARTESIAN_POINT('Ctrl Pts',(-11.3173736352187,4.19739582695453,2.87344615271929));
#41340=CARTESIAN_POINT('Ctrl Pts',(-11.3224917296601,4.32232029305708,2.74716689547289));
#41341=CARTESIAN_POINT('Ctrl Pts',(-11.33179988888,4.53477391826449,2.50096807962284));
#41342=CARTESIAN_POINT('Ctrl Pts',(-11.3360024161493,4.62443130074115,2.38445811548733));
#41343=CARTESIAN_POINT('Ctrl Pts',(-11.3433948737295,4.76619281627191,2.17704619649897));
#41344=CARTESIAN_POINT('Ctrl Pts',(-11.3464900793102,4.82130673923218,2.08917298194309));
#41345=CARTESIAN_POINT('Ctrl Pts',(-11.3496160435307,4.87293858259124,1.99930017380816));
#41346=CARTESIAN_POINT('Ctrl Pts',(-11.6558295573,4.94740519195,0.3717962675248));
#41347=CARTESIAN_POINT('Ctrl Pts',(-11.62874622397,4.863047294756,1.174408046021));
#41348=CARTESIAN_POINT('Ctrl Pts',(-11.5745795573,4.126976592789,2.716457858798));
#41349=CARTESIAN_POINT('Ctrl Pts',(-11.4933295573,1.811618102055,3.821392544123));
#41350=CARTESIAN_POINT('Ctrl Pts',(-11.4120795573,-0.6826713958586,3.22240311641));
#41351=CARTESIAN_POINT('Ctrl Pts',(-11.3308295573,-2.244260024069,1.187349778821));
#41352=CARTESIAN_POINT('Ctrl Pts',(-11.2495795573,-2.177110172115,-1.37696510205));
#41353=CARTESIAN_POINT('Ctrl Pts',(-11.1683295573,-0.5111577555903,-3.327542075668));
#41354=CARTESIAN_POINT('Ctrl Pts',(-11.0870795573,2.011070568446,-3.795010270395));
#41355=CARTESIAN_POINT('Ctrl Pts',(-11.0058295573,4.265396783812,-2.571010770076));
#41356=CARTESIAN_POINT('Ctrl Pts',(-10.9245795573,5.247049616522,-0.2010912618048));
#41357=CARTESIAN_POINT('Ctrl Pts',(-10.8433295573,4.518498435686,2.258456315361));
#41358=CARTESIAN_POINT('Ctrl Pts',(-10.7620795573,2.404464396407,3.711391652462));
#41359=CARTESIAN_POINT('Ctrl Pts',(-10.6808295573,-0.1528104572481,3.510129757805));
#41360=CARTESIAN_POINT('Ctrl Pts',(-10.5995795573,-2.013528067013,1.744374677141));
#41361=CARTESIAN_POINT('Ctrl Pts',(-10.5183295573,-2.348351565217,-0.798862286232));
#41362=CARTESIAN_POINT('Ctrl Pts',(-10.4370795573,-1.008047414265,-2.986039876248));
#41363=CARTESIAN_POINT('Ctrl Pts',(-10.3558295573,1.41,-3.842315374891));
#41364=CARTESIAN_POINT('Ctrl Pts',(-10.2745795573,3.828047414265,-2.986039876248));
#41365=CARTESIAN_POINT('Ctrl Pts',(-10.1933295573,5.168351565217,-0.7988622862319));
#41366=CARTESIAN_POINT('Ctrl Pts',(-10.1120795573,4.833528067013,1.744374677141));
#41367=CARTESIAN_POINT('Ctrl Pts',(-10.0308295573,2.972810457248,3.510129757805));
#41368=CARTESIAN_POINT('Ctrl Pts',(-9.949579557301,0.4155356035931,3.711391652462));
#41369=CARTESIAN_POINT('Ctrl Pts',(-9.868329557301,-1.698498435686,2.258456315361));
#41370=CARTESIAN_POINT('Ctrl Pts',(-9.787079557301,-2.427049616522,-0.2010912618048));
#41371=CARTESIAN_POINT('Ctrl Pts',(-9.705829557301,-1.445396783812,-2.571010770076));
#41372=CARTESIAN_POINT('Ctrl Pts',(-9.624579557301,0.8089294315536,-3.795010270395));
#41373=CARTESIAN_POINT('Ctrl Pts',(-9.543329557301,3.33115775559,-3.327542075668));
#41374=CARTESIAN_POINT('Ctrl Pts',(-9.462079557301,4.997110172115,-1.37696510205));
#41375=CARTESIAN_POINT('Ctrl Pts',(-9.380829557301,5.064260024069,1.187349778821));
#41376=CARTESIAN_POINT('Ctrl Pts',(-9.299579557301,3.502671395859,3.22240311641));
#41377=CARTESIAN_POINT('Ctrl Pts',(-9.218329557301,1.008381897945,3.821392544123));
#41378=CARTESIAN_POINT('Ctrl Pts',(-9.137079557301,-1.306976592789,2.716457858798));
#41379=CARTESIAN_POINT('Ctrl Pts',(-9.082912890634,-2.043047294756,1.174408046021));
#41380=CARTESIAN_POINT('Ctrl Pts',(-9.055829557301,-2.12740519195,0.3717962675247));
#41381=CARTESIAN_POINT('Ctrl Pts',(-11.56225655499,5.10859053225,0.388737529453));
#41382=CARTESIAN_POINT('Ctrl Pts',(-11.53517322166,5.020388784654,1.227921101574));
#41383=CARTESIAN_POINT('Ctrl Pts',(-11.48100655499,4.250778298539,2.840235927925));
#41384=CARTESIAN_POINT('Ctrl Pts',(-11.39975655499,1.82991822515,3.99551804692));
#41385=CARTESIAN_POINT('Ctrl Pts',(-11.31850655499,-0.7780260224205,3.369235077895));
#41386=CARTESIAN_POINT('Ctrl Pts',(-11.23725655499,-2.410769969513,1.241452537133));
#41387=CARTESIAN_POINT('Ctrl Pts',(-11.15600655499,-2.340560368632,-1.439707868714));
#41388=CARTESIAN_POINT('Ctrl Pts',(-11.07475655499,-0.5986971947557,-3.479164797048));
#41389=CARTESIAN_POINT('Ctrl Pts',(-10.99350655499,2.038458938978,-3.967933638989));
#41390=CARTESIAN_POINT('Ctrl Pts',(-10.91225655499,4.395505741456,-2.688161399818));
#41391=CARTESIAN_POINT('Ctrl Pts',(-10.83100655499,5.421888549192,-0.2102541825635));
#41392=CARTESIAN_POINT('Ctrl Pts',(-10.74975655499,4.660140218572,2.361365094534));
#41393=CARTESIAN_POINT('Ctrl Pts',(-10.66850655499,2.449778142911,3.88050485664));
#41394=CARTESIAN_POINT('Ctrl Pts',(-10.58725655499,-0.2240214499691,3.670072266171));
#41395=CARTESIAN_POINT('Ctrl Pts',(-10.50600655499,-2.16952448432,1.823858821786));
#41396=CARTESIAN_POINT('Ctrl Pts',(-10.42475655499,-2.519604543921,-0.8352632305602));
#41397=CARTESIAN_POINT('Ctrl Pts',(-10.34350655499,-1.118228118532,-3.122101714653));
#41398=CARTESIAN_POINT('Ctrl Pts',(-10.26225655499,1.41,-4.017394247012));
#41399=CARTESIAN_POINT('Ctrl Pts',(-10.18100655499,3.938228118532,-3.122101714653));
#41400=CARTESIAN_POINT('Ctrl Pts',(-10.09975655499,5.339604543921,-0.8352632305602));
#41401=CARTESIAN_POINT('Ctrl Pts',(-10.01850655499,4.98952448432,1.823858821786));
#41402=CARTESIAN_POINT('Ctrl Pts',(-9.937256554992,3.044021449969,3.670072266171));
#41403=CARTESIAN_POINT('Ctrl Pts',(-9.856006554992,0.3702218570889,3.88050485664));
#41404=CARTESIAN_POINT('Ctrl Pts',(-9.774756554992,-1.840140218572,2.361365094534));
#41405=CARTESIAN_POINT('Ctrl Pts',(-9.693506554992,-2.601888549192,-0.2102541825635));
#41406=CARTESIAN_POINT('Ctrl Pts',(-9.612256554992,-1.575505741456,-2.688161399818));
#41407=CARTESIAN_POINT('Ctrl Pts',(-9.531006554992,0.7815410610216,-3.967933638989));
#41408=CARTESIAN_POINT('Ctrl Pts',(-9.449756554992,3.418697194756,-3.479164797048));
#41409=CARTESIAN_POINT('Ctrl Pts',(-9.368506554992,5.160560368632,-1.439707868714));
#41410=CARTESIAN_POINT('Ctrl Pts',(-9.287256554992,5.230769969513,1.241452537133));
#41411=CARTESIAN_POINT('Ctrl Pts',(-9.206006554992,3.59802602242,3.369235077895));
#41412=CARTESIAN_POINT('Ctrl Pts',(-9.124756554992,0.9900817748502,3.99551804692));
#41413=CARTESIAN_POINT('Ctrl Pts',(-9.043506554992,-1.430778298539,2.840235927925));
#41414=CARTESIAN_POINT('Ctrl Pts',(-8.989339888326,-2.200388784654,1.227921101574));
#41415=CARTESIAN_POINT('Ctrl Pts',(-8.962256554992,-2.28859053225,0.388737529453));
#41416=CARTESIAN_POINT('Ctrl Pts',(-11.46868355268,5.269775872549,0.4056787913812));
#41417=CARTESIAN_POINT('Ctrl Pts',(-11.44160021935,5.177730274553,1.281434157126));
#41418=CARTESIAN_POINT('Ctrl Pts',(-11.38743355268,4.37458000429,2.964013997052));
#41419=CARTESIAN_POINT('Ctrl Pts',(-11.30618355268,1.848218348245,4.169643549716));
#41420=CARTESIAN_POINT('Ctrl Pts',(-11.22493355268,-0.8733806489824,3.51606703938));
#41421=CARTESIAN_POINT('Ctrl Pts',(-11.14368355268,-2.577279914956,1.295555295446));
#41422=CARTESIAN_POINT('Ctrl Pts',(-11.06243355268,-2.504010565149,-1.502450635378));
#41423=CARTESIAN_POINT('Ctrl Pts',(-10.98118355268,-0.686236633921,-3.630787518428));
#41424=CARTESIAN_POINT('Ctrl Pts',(-10.89993355268,2.06584730951,-4.140857007583));
#41425=CARTESIAN_POINT('Ctrl Pts',(-10.81868355268,4.5256146991,-2.805312029559));
#41426=CARTESIAN_POINT('Ctrl Pts',(-10.73743355268,5.596727481863,-0.2194171033222));
#41427=CARTESIAN_POINT('Ctrl Pts',(-10.65618355268,4.801782001457,2.464273873707));
#41428=CARTESIAN_POINT('Ctrl Pts',(-10.57493355268,2.495091889415,4.049618060818));
#41429=CARTESIAN_POINT('Ctrl Pts',(-10.49368355268,-0.2952324426901,3.830014774536));
#41430=CARTESIAN_POINT('Ctrl Pts',(-10.41243355268,-2.325520901626,1.903342966431));
#41431=CARTESIAN_POINT('Ctrl Pts',(-10.33118355268,-2.690857522625,-0.8716641748885));
#41432=CARTESIAN_POINT('Ctrl Pts',(-10.24993355268,-1.2284088228,-3.258163553058));
#41433=CARTESIAN_POINT('Ctrl Pts',(-10.16868355268,1.41,-4.192473119132));
#41434=CARTESIAN_POINT('Ctrl Pts',(-10.08743355268,4.0484088228,-3.258163553058));
#41435=CARTESIAN_POINT('Ctrl Pts',(-10.00618355268,5.510857522625,-0.8716641748885));
#41436=CARTESIAN_POINT('Ctrl Pts',(-9.924933552684,5.145520901626,1.903342966431));
#41437=CARTESIAN_POINT('Ctrl Pts',(-9.843683552684,3.11523244269,3.830014774536));
#41438=CARTESIAN_POINT('Ctrl Pts',(-9.762433552684,0.3249081105847,4.049618060818));
#41439=CARTESIAN_POINT('Ctrl Pts',(-9.681183552684,-1.981782001457,2.464273873707));
#41440=CARTESIAN_POINT('Ctrl Pts',(-9.599933552684,-2.776727481863,-0.2194171033222));
#41441=CARTESIAN_POINT('Ctrl Pts',(-9.518683552684,-1.7056146991,-2.805312029559));
#41442=CARTESIAN_POINT('Ctrl Pts',(-9.437433552684,0.7541526904896,-4.140857007583));
#41443=CARTESIAN_POINT('Ctrl Pts',(-9.356183552684,3.506236633921,-3.630787518428));
#41444=CARTESIAN_POINT('Ctrl Pts',(-9.274933552684,5.324010565149,-1.502450635378));
#41445=CARTESIAN_POINT('Ctrl Pts',(-9.193683552684,5.397279914956,1.295555295446));
#41446=CARTESIAN_POINT('Ctrl Pts',(-9.112433552684,3.693380648982,3.51606703938));
#41447=CARTESIAN_POINT('Ctrl Pts',(-9.031183552684,0.9717816517551,4.169643549716));
#41448=CARTESIAN_POINT('Ctrl Pts',(-8.949933552684,-1.55458000429,2.964013997052));
#41449=CARTESIAN_POINT('Ctrl Pts',(-8.895766886017,-2.357730274553,1.281434157126));
#41450=CARTESIAN_POINT('Ctrl Pts',(-8.868683552684,-2.449775872549,0.4056787913812));
#41451=CARTESIAN_POINT('Ctrl Pts',(-11.37511055037,5.430961212849,0.4226200533094));
#41452=CARTESIAN_POINT('Ctrl Pts',(-11.34802721704,5.335071764451,1.334947212679));
#41453=CARTESIAN_POINT('Ctrl Pts',(-11.29386055037,4.49838171004,3.087792066179));
#41454=CARTESIAN_POINT('Ctrl Pts',(-11.21261055037,1.86651847134,4.343769052512));
#41455=CARTESIAN_POINT('Ctrl Pts',(-11.13136055037,-0.9687352755443,3.662899000864));
#41456=CARTESIAN_POINT('Ctrl Pts',(-11.05011055037,-2.743789860399,1.349658053758));
#41457=CARTESIAN_POINT('Ctrl Pts',(-10.96886055037,-2.667460761666,-1.565193402042));
#41458=CARTESIAN_POINT('Ctrl Pts',(-10.88761055037,-0.7737760730864,-3.782410239809));
#41459=CARTESIAN_POINT('Ctrl Pts',(-10.80636055037,2.093235680042,-4.313780376177));
#41460=CARTESIAN_POINT('Ctrl Pts',(-10.72511055037,4.655723656744,-2.922462659301));
#41461=CARTESIAN_POINT('Ctrl Pts',(-10.64386055037,5.771566414534,-0.2285800240809));
#41462=CARTESIAN_POINT('Ctrl Pts',(-10.56261055037,4.943423784343,2.56718265288));
#41463=CARTESIAN_POINT('Ctrl Pts',(-10.48136055037,2.540405635919,4.218731264996));
#41464=CARTESIAN_POINT('Ctrl Pts',(-10.40011055037,-0.3664434354111,3.989957282902));
#41465=CARTESIAN_POINT('Ctrl Pts',(-10.31886055037,-2.481517318933,1.982827111076));
#41466=CARTESIAN_POINT('Ctrl Pts',(-10.23761055037,-2.862110501329,-0.9080651192168));
#41467=CARTESIAN_POINT('Ctrl Pts',(-10.15636055037,-1.338589527067,-3.394225391463));
#41468=CARTESIAN_POINT('Ctrl Pts',(-10.07511055037,1.41,-4.367551991253));
#41469=CARTESIAN_POINT('Ctrl Pts',(-9.993860550375,4.158589527067,-3.394225391463));
#41470=CARTESIAN_POINT('Ctrl Pts',(-9.912610550375,5.682110501329,-0.9080651192168));
#41471=CARTESIAN_POINT('Ctrl Pts',(-9.831360550375,5.301517318933,1.982827111076));
#41472=CARTESIAN_POINT('Ctrl Pts',(-9.750110550375,3.186443435411,3.989957282902));
#41473=CARTESIAN_POINT('Ctrl Pts',(-9.668860550375,0.2795943640806,4.218731264996));
#41474=CARTESIAN_POINT('Ctrl Pts',(-9.587610550375,-2.123423784343,2.56718265288));
#41475=CARTESIAN_POINT('Ctrl Pts',(-9.506360550375,-2.951566414534,-0.2285800240809));
#41476=CARTESIAN_POINT('Ctrl Pts',(-9.425110550375,-1.835723656744,-2.922462659301));
#41477=CARTESIAN_POINT('Ctrl Pts',(-9.343860550375,0.7267643199575,-4.313780376177));
#41478=CARTESIAN_POINT('Ctrl Pts',(-9.262610550375,3.593776073086,-3.782410239809));
#41479=CARTESIAN_POINT('Ctrl Pts',(-9.181360550375,5.487460761666,-1.565193402042));
#41480=CARTESIAN_POINT('Ctrl Pts',(-9.100110550375,5.563789860399,1.349658053758));
#41481=CARTESIAN_POINT('Ctrl Pts',(-9.018860550375,3.788735275544,3.662899000864));
#41482=CARTESIAN_POINT('Ctrl Pts',(-8.937610550375,0.9534815286599,4.343769052512));
#41483=CARTESIAN_POINT('Ctrl Pts',(-8.856360550375,-1.67838171004,3.087792066179));
#41484=CARTESIAN_POINT('Ctrl Pts',(-8.802193883708,-2.515071764451,1.334947212679));
#41485=CARTESIAN_POINT('Ctrl Pts',(-8.775110550375,-2.610961212849,0.4226200533094));
#41486=CARTESIAN_POINT('',(-8.85049707793188,-2.05335595069089,1.99956949126325));
#41487=CARTESIAN_POINT('Ctrl Pts',(-9.60040561164376,-2.05290755290942,
1.99927856802735));
#41488=CARTESIAN_POINT('Ctrl Pts',(-9.592648539488,-2.1776137658591,1.78299963277453));
#41489=CARTESIAN_POINT('Ctrl Pts',(-9.58470884554327,-2.28217153326222,
1.55504283182618));
#41490=CARTESIAN_POINT('Ctrl Pts',(-9.57348439445244,-2.40287751946333,
1.21030822786898));
#41491=CARTESIAN_POINT('Ctrl Pts',(-9.56998824900667,-2.43637685170845,
1.09948652005087));
#41492=CARTESIAN_POINT('Ctrl Pts',(-9.56104116063325,-2.51151184159235,
0.804747256195322));
#41493=CARTESIAN_POINT('Ctrl Pts',(-9.55572697913885,-2.54503434182388,
0.6189391301607));
#41494=CARTESIAN_POINT('Ctrl Pts',(-9.54639135395835,-2.58076150842344,
0.289758296971684));
#41495=CARTESIAN_POINT('Ctrl Pts',(-9.5423673684783,-2.58858131215265,0.147003740181955));
#41496=CARTESIAN_POINT('Ctrl Pts',(-9.53507432994476,-2.58884776661925,
-0.105680704039776));
#41497=CARTESIAN_POINT('Ctrl Pts',(-9.53184207956503,-2.58441720541216,
-0.215490452908572));
#41498=CARTESIAN_POINT('Ctrl Pts',(-9.52280012432087,-2.55989678693276,
-0.513982059176623));
#41499=CARTESIAN_POINT('Ctrl Pts',(-9.51686679260937,-2.53091011969018,
-0.701672132362012));
#41500=CARTESIAN_POINT('Ctrl Pts',(-9.50588507958739,-2.45341801109884,
-1.04246274749219));
#41501=CARTESIAN_POINT('Ctrl Pts',(-9.50084214484328,-2.40862312286159,
-1.19645621581327));
#41502=CARTESIAN_POINT('Ctrl Pts',(-9.49233887140167,-2.3158703794896,-1.45621742318579));
#41503=CARTESIAN_POINT('Ctrl Pts',(-9.48882592440186,-2.27219666730552,
-1.56360618312295));
#41504=CARTESIAN_POINT('Ctrl Pts',(-9.48029499114608,-2.15159532242807,
-1.82637699560855));
#41505=CARTESIAN_POINT('Ctrl Pts',(-9.47538062504686,-2.069064105986,-1.97900341303359));
#41506=CARTESIAN_POINT('Ctrl Pts',(-9.46615567140573,-1.89546155828856,
-2.25561353392233));
#41507=CARTESIAN_POINT('Ctrl Pts',(-9.46183917000714,-1.80644120827349,
-2.38087096327682));
#41508=CARTESIAN_POINT('Ctrl Pts',(-9.45415180995853,-1.63964141944734,
-2.58902989023001));
#41509=CARTESIAN_POINT('Ctrl Pts',(-9.45082545411876,-1.56505867046786,
-2.67437719622726));
#41510=CARTESIAN_POINT('Ctrl Pts',(-9.44193507944392,-1.3616794778249,-2.88785816818869));
#41511=CARTESIAN_POINT('Ctrl Pts',(-9.4362720629285,-1.22761667937358,-3.01060219187097));
#41512=CARTESIAN_POINT('Ctrl Pts',(-9.42537925227153,-0.956317980604446,
-3.22729703651813));
#41513=CARTESIAN_POINT('Ctrl Pts',(-9.42015377674645,-0.820292770316238,
-3.32283525765303));
#41514=CARTESIAN_POINT('Ctrl Pts',(-9.41140145470753,-0.578262866398371,
-3.47131975099939));
#41515=CARTESIAN_POINT('Ctrl Pts',(-9.40781778162555,-0.474838742752067,
-3.52864839224943));
#41516=CARTESIAN_POINT('Ctrl Pts',(-9.39902837168875,-0.208041882939476,
-3.66125372848236));
#41517=CARTESIAN_POINT('Ctrl Pts',(-9.39393789067322,-0.0417324379309015,
-3.73027639780195));
#41518=CARTESIAN_POINT('Ctrl Pts',(-9.38462373683353,0.270802409734637,
-3.83600739585551));
#41519=CARTESIAN_POINT('Ctrl Pts',(-9.3803935544249,0.415853012911651,-3.87615241357383));
#41520=CARTESIAN_POINT('Ctrl Pts',(-9.37282172899103,0.672504693060417,
-3.93180158109821));
#41521=CARTESIAN_POINT('Ctrl Pts',(-9.36952225777246,0.783217461030843,
-3.95094716539007));
#41522=CARTESIAN_POINT('Ctrl Pts',(-9.36057767995255,1.07730095533725,-3.98898846612685));
#41523=CARTESIAN_POINT('Ctrl Pts',(-9.35482582565714,1.26143084800293,-3.99993400067362));
#41524=CARTESIAN_POINT('Ctrl Pts',(-9.34390302474602,1.60941374719111,-3.996804169109));
#41525=CARTESIAN_POINT('Ctrl Pts',(-9.33873705567264,1.77333514304933,-3.985318970206));
#41526=CARTESIAN_POINT('Ctrl Pts',(-9.33006499181736,2.05225354082227,-3.94849144148094));
#41527=CARTESIAN_POINT('Ctrl Pts',(-9.32650344265707,2.16798340920093,-3.92801068498396));
#41528=CARTESIAN_POINT('Ctrl Pts',(-9.31770187978694,2.45914821402567,-3.8629718548007));
#41529=CARTESIAN_POINT('Ctrl Pts',(-9.31258089141444,2.63287631226559,-3.81149482924049));
#41530=CARTESIAN_POINT('Ctrl Pts',(-9.30325830244933,2.94244192303581,-3.69650349598188));
#41531=CARTESIAN_POINT('Ctrl Pts',(-9.29905027707537,3.07961834901688,-3.63662675072915));
#41532=CARTESIAN_POINT('Ctrl Pts',(-9.29150488237336,3.31315682168349,-3.51865862815614));
#41533=CARTESIAN_POINT('Ctrl Pts',(-9.28820897884544,3.41107967410374,-3.4638869342709));
#41534=CARTESIAN_POINT('Ctrl Pts',(-9.27854372821509,3.6837784145769,-3.29574888792376));
#41535=CARTESIAN_POINT('Ctrl Pts',(-9.27201150657151,3.85227437190568,-3.17269744237438));
#41536=CARTESIAN_POINT('Ctrl Pts',(-9.26076563378601,4.12433811974851,-2.93979520510097));
#41537=CARTESIAN_POINT('Ctrl Pts',(-9.25605159748808,4.23295854266567,-2.83576544018229));
#41538=CARTESIAN_POINT('Ctrl Pts',(-9.2479582242247,4.4126197712042,-2.64320887657756));
#41539=CARTESIAN_POINT('Ctrl Pts',(-9.24453637118187,4.48636945008601,-2.55712563604215));
#41540=CARTESIAN_POINT('Ctrl Pts',(-9.23527915118763,4.68063272081885,-2.30955700187998));
#41541=CARTESIAN_POINT('Ctrl Pts',(-9.22961408698511,4.79281112244183,-2.14179114553789));
#41542=CARTESIAN_POINT('Ctrl Pts',(-9.21884251351113,4.98047464746399,-1.80954647457836));
#41543=CARTESIAN_POINT('Ctrl Pts',(-9.21373710578579,5.05855440007191,-1.64655360337947));
#41544=CARTESIAN_POINT('Ctrl Pts',(-9.20505023257498,5.16751183864385,-1.37267062905776));
#41545=CARTESIAN_POINT('Ctrl Pts',(-9.20158993180501,5.20513996551312,-1.26465070786087));
#41546=CARTESIAN_POINT('Ctrl Pts',(-9.19343918098472,5.28149413823754,-1.01106616003464));
#41547=CARTESIAN_POINT('Ctrl Pts',(-9.18870681802321,5.31678442944973,-0.864384964301256));
#41548=CARTESIAN_POINT('Ctrl Pts',(-9.17739515814574,5.38131982281984,-0.509975379617664));
#41549=CARTESIAN_POINT('Ctrl Pts',(-9.17081921067416,5.40279186905983,-0.300777659727165));
#41550=CARTESIAN_POINT('Ctrl Pts',(-9.16110302171323,5.41033007588258,0.0221346401150478));
#41551=CARTESIAN_POINT('Ctrl Pts',(-9.15779006413838,5.40810872064692,0.13533898255474));
#41552=CARTESIAN_POINT('Ctrl Pts',(-9.1501099337789,5.39152354672244,0.401818718343227));
#41553=CARTESIAN_POINT('Ctrl Pts',(-9.14578574227475,5.37308243798484,0.554813369105755));
#41554=CARTESIAN_POINT('Ctrl Pts',(-9.1365314088165,5.31523418561994,0.877269127846519));
#41555=CARTESIAN_POINT('Ctrl Pts',(-9.13159401369815,5.27342523279836,1.04628752255256));
#41556=CARTESIAN_POINT('Ctrl Pts',(-9.12291148671605,5.1843800684607,1.32601600955524));
#41557=CARTESIAN_POINT('Ctrl Pts',(-9.11926957743045,5.14287952611652,1.43844054224961));
#41558=CARTESIAN_POINT('Ctrl Pts',(-9.11039177534989,5.03139259821727,1.70335638586575));
#41559=CARTESIAN_POINT('Ctrl Pts',(-9.10510023615257,4.95660383324509,1.85391807599278));
#41560=CARTESIAN_POINT('Ctrl Pts',(-9.09423927196797,4.78354047908282,2.15381290277887));
#41561=CARTESIAN_POINT('Ctrl Pts',(-9.08867386848596,4.68404755562057,2.30249311099628));
#41562=CARTESIAN_POINT('Ctrl Pts',(-9.07990374444557,4.50603297095058,2.53329501675828));
#41563=CARTESIAN_POINT('Ctrl Pts',(-9.07660075824385,4.43335574420623,2.61961582623421));
#41564=CARTESIAN_POINT('Ctrl Pts',(-9.06896979110242,4.25409634850611,2.81507344530256));
#41565=CARTESIAN_POINT('Ctrl Pts',(-9.06468373933528,4.14461929465385,2.92151190694135));
#41566=CARTESIAN_POINT('Ctrl Pts',(-9.05539340321852,3.89608227609904,3.13700171113091));
#41567=CARTESIAN_POINT('Ctrl Pts',(-9.05038120579234,3.75508985350886,3.24380605163546));
#41568=CARTESIAN_POINT('Ctrl Pts',(-9.04159512009966,3.50686187688791,3.40699539292465));
#41569=CARTESIAN_POINT('Ctrl Pts',(-9.03792977313163,3.4031621408114,3.4685727911801));
#41570=CARTESIAN_POINT('Ctrl Pts',(-9.02896739234424,3.14725711947419,3.60535098970956));
#41571=CARTESIAN_POINT('Ctrl Pts',(-9.0236134674557,2.99245342224551,3.67586783017103));
#41572=CARTESIAN_POINT('Ctrl Pts',(-9.01278533577553,2.66972272653378,3.79894303584769));
#41573=CARTESIAN_POINT('Ctrl Pts',(-9.00731356779278,2.50148472998555,3.85080686984647));
#41574=CARTESIAN_POINT('Ctrl Pts',(-8.99860131029036,2.21963774923441,3.91764290759745));
#41575=CARTESIAN_POINT('Ctrl Pts',(-8.99527062217913,2.10782053336575,3.93910479370828));
#41576=CARTESIAN_POINT('Ctrl Pts',(-8.98752159965826,1.84129132913886,3.97852936330207));
#41577=CARTESIAN_POINT('Ctrl Pts',(-8.98314744245908,1.68598465452508,3.99229038034456));
#41578=CARTESIAN_POINT('Ctrl Pts',(-8.97394664224195,1.36059820382706,4.00209870554907));
#41579=CARTESIAN_POINT('Ctrl Pts',(-8.9691140595699,1.19047788812806,3.99641147226209));
#41580=CARTESIAN_POINT('Ctrl Pts',(-8.96059716426728,0.903927748838954,
3.96834102692915));
#41581=CARTESIAN_POINT('Ctrl Pts',(-8.95700957819773,0.787066552216668,
3.95158223146842));
#41582=CARTESIAN_POINT('Ctrl Pts',(-8.94831693167847,0.510559749166548,
3.89940737616986));
#41583=CARTESIAN_POINT('Ctrl Pts',(-8.94315879217041,0.351720107753647,
3.85925077816371));
#41584=CARTESIAN_POINT('Ctrl Pts',(-8.93223114940881,0.0201993913987,3.75364135889862));
#41585=CARTESIAN_POINT('Ctrl Pts',(-8.92646800622479,-0.151703930561329,
3.68559482016283));
#41586=CARTESIAN_POINT('Ctrl Pts',(-8.91759357809553,-0.41751404746469,
3.55838411955562));
#41587=CARTESIAN_POINT('Ctrl Pts',(-8.91436575366286,-0.514758393542523,
3.50675051154773));
#41588=CARTESIAN_POINT('Ctrl Pts',(-8.90704049634875,-0.734254785941745,
3.37829084050234));
#41589=CARTESIAN_POINT('Ctrl Pts',(-8.9029793843837,-0.854810071293984,
3.29866643381797));
#41590=CARTESIAN_POINT('Ctrl Pts',(-8.89365713134142,-1.12044496397458,
3.10185526197797));
#41591=CARTESIAN_POINT('Ctrl Pts',(-8.88838974677078,-1.2624183779927,2.98049157119333));
#41592=CARTESIAN_POINT('Ctrl Pts',(-8.8794044082883,-1.47951408331325,2.7667175653459));
#41593=CARTESIAN_POINT('Ctrl Pts',(-8.87581931075566,-1.56003831183313,
2.6799717451396));
#41594=CARTESIAN_POINT('Ctrl Pts',(-8.86475153953041,-1.79264008377585,
2.40606890783807));
#41595=CARTESIAN_POINT('Ctrl Pts',(-8.85708769733734,-1.93217852399906,
2.20811551137394));
#41596=CARTESIAN_POINT('Ctrl Pts',(-8.84959438835624,-2.05287980560813,
1.99932662776271));
#41597=CARTESIAN_POINT('',(-9.080940107676,-1.707691453624,1.8));
#41598=CARTESIAN_POINT('Ctrl Pts',(-9.155829557301,-0.6806876086837,2.877584625945));
#41599=CARTESIAN_POINT('Ctrl Pts',(-9.128746223968,-1.333590849641,2.403222654717));
#41600=CARTESIAN_POINT('Ctrl Pts',(-9.074579557301,-2.301009810423,0.9947418214436));
#41601=CARTESIAN_POINT('Ctrl Pts',(-8.993329557301,-2.10023207207,-1.562884793063));
#41602=CARTESIAN_POINT('Ctrl Pts',(-8.912079557301,-0.3343472621158,-3.423508148791));
#41603=CARTESIAN_POINT('Ctrl Pts',(-8.830829557301,2.208854940398,-3.758356902288));
#41604=CARTESIAN_POINT('Ctrl Pts',(-8.749579557301,4.396041844558,-2.418045984201));
#41605=CARTESIAN_POINT('Ctrl Pts',(-8.668329557301,5.252314847485,-3.831845932778E-7));
#41606=CARTESIAN_POINT('Ctrl Pts',(-8.587079557301,4.396040017561,2.418047516939));
#41607=CARTESIAN_POINT('Ctrl Pts',(-8.505829557301,2.208862248383,3.758351537704));
#41608=CARTESIAN_POINT('Ctrl Pts',(-8.424579557301,-0.3343746670588,3.423528074391));
#41609=CARTESIAN_POINT('Ctrl Pts',(-8.343329557301,-2.100129760283,1.562810455248));
#41610=CARTESIAN_POINT('Ctrl Pts',(-8.262079557301,-2.301391652629,-0.9944643957835));
#41611=CARTESIAN_POINT('Ctrl Pts',(-8.180829557301,-0.8484563122144,-3.108498436179));
#41612=CARTESIAN_POINT('Ctrl Pts',(-8.099579557301,1.611091249384,-3.837049615173));
#41613=CARTESIAN_POINT('Ctrl Pts',(-8.018329557301,3.981010816611,-2.855396788715));
#41614=CARTESIAN_POINT('Ctrl Pts',(-7.937079557301,5.205010096676,-0.6010705501845));
#41615=CARTESIAN_POINT('Ctrl Pts',(-7.855829557301,4.737542724007,1.921157687446));
#41616=CARTESIAN_POINT('Ctrl Pts',(-7.774579557301,2.786962682412,3.587110426432));
#41617=CARTESIAN_POINT('Ctrl Pts',(-7.693329557301,0.2226592513938,3.654259074947));
#41618=CARTESIAN_POINT('Ctrl Pts',(-7.612079557301,-1.812436817629,2.092674938032));
#41619=CARTESIAN_POINT('Ctrl Pts',(-7.530829557301,-2.411266769463,-0.4016313216255));
#41620=CARTESIAN_POINT('Ctrl Pts',(-7.449579557301,-1.306927256222,-2.716927256679));
#41621=CARTESIAN_POINT('Ctrl Pts',(-7.368329557301,1.008368675403,-3.821266770609));
#41622=CARTESIAN_POINT('Ctrl Pts',(-7.287079557301,3.502674949463,-3.222436812587));
#41623=CARTESIAN_POINT('Ctrl Pts',(-7.205829557301,5.064259032195,-1.187340767628));
#41624=CARTESIAN_POINT('Ctrl Pts',(-7.124579557301,4.997110586008,1.376962753456));
#41625=CARTESIAN_POINT('Ctrl Pts',(-7.043329557301,3.331157091895,3.327542458853));
#41626=CARTESIAN_POINT('Ctrl Pts',(-6.962079557301,0.8089316724422,3.795011086251));
#41627=CARTESIAN_POINT('Ctrl Pts',(-6.880829557301,-1.445405083671,2.571007123468));
#41628=CARTESIAN_POINT('Ctrl Pts',(-6.799579557301,-2.427018657974,0.2011050323817));
#41629=CARTESIAN_POINT('Ctrl Pts',(-6.718329557301,-1.698613970016,-2.258507751061));
#41630=CARTESIAN_POINT('Ctrl Pts',(-6.637079557301,0.4159667823653,-3.711199680242));
#41631=CARTESIAN_POINT('Ctrl Pts',(-6.582912890634,2.119456445115,-3.577630700739));
#41632=CARTESIAN_POINT('Ctrl Pts',(-6.555829557301,2.856717583266,-3.24938089347));
#41633=CARTESIAN_POINT('Ctrl Pts',(-9.062256554992,-0.7759518420355,3.008704594398));
#41634=CARTESIAN_POINT('Ctrl Pts',(-9.035173221659,-1.458605260133,2.512727854262));
#41635=CARTESIAN_POINT('Ctrl Pts',(-8.981006554992,-2.470105615594,1.040068209092));
#41636=CARTESIAN_POINT('Ctrl Pts',(-8.899756554992,-2.260179242486,-1.634099172968));
#41637=CARTESIAN_POINT('Ctrl Pts',(-8.818506554992,-0.4138301575682,-3.579503658505));
#41638=CARTESIAN_POINT('Ctrl Pts',(-8.737256554992,2.245255550006,-3.929610124181));
#41639=CARTESIAN_POINT('Ctrl Pts',(-8.656006554992,4.532103772651,-2.528226623306));
#41640=CARTESIAN_POINT('Ctrl Pts',(-8.574756554992,5.427393695574,-4.006447741335E-7));
#41641=CARTESIAN_POINT('Ctrl Pts',(-8.493506554992,4.532101862406,2.528228225885));
#41642=CARTESIAN_POINT('Ctrl Pts',(-8.412256554992,2.245263190987,3.929604515154));
#41643=CARTESIAN_POINT('Ctrl Pts',(-8.331006554992,-0.4138588112444,3.579524492034));
#41644=CARTESIAN_POINT('Ctrl Pts',(-8.249756554992,-2.260072268762,1.634021447877));
#41645=CARTESIAN_POINT('Ctrl Pts',(-8.168506554992,-2.470504856815,-1.039778142259));
#41646=CARTESIAN_POINT('Ctrl Pts',(-8.087256554992,-0.9513650912439,-3.250140219087));
#41647=CARTESIAN_POINT('Ctrl Pts',(-8.006006554992,1.620254169577,-4.011888547782));
#41648=CARTESIAN_POINT('Ctrl Pts',(-7.924756554992,4.098161448473,-2.985505746582));
#41649=CARTESIAN_POINT('Ctrl Pts',(-7.843506554992,5.377933457354,-0.6284589198844));
#41650=CARTESIAN_POINT('Ctrl Pts',(-7.762256554992,4.88916547493,2.008697123506));
#41651=CARTESIAN_POINT('Ctrl Pts',(-7.681006554992,2.849705338822,3.750560634537));
#41652=CARTESIAN_POINT('Ctrl Pts',(-7.599756554992,0.1685569045517,3.820768977142));
#41653=CARTESIAN_POINT('Ctrl Pts',(-7.518506554992,-1.959270314743,2.188029725996));
#41654=CARTESIAN_POINT('Ctrl Pts',(-7.437256554992,-2.585386541213,-0.4199320470833));
#41655=CARTESIAN_POINT('Ctrl Pts',(-7.356006554992,-1.430726713904,-2.840726714381));
#41656=CARTESIAN_POINT('Ctrl Pts',(-7.274756554992,0.9900679498094,-3.995386542412));
#41657=CARTESIAN_POINT('Ctrl Pts',(-7.193506554992,3.598029737948,-3.369270309471));
#41658=CARTESIAN_POINT('Ctrl Pts',(-7.112256554992,5.230768932443,-1.241443115336));
#41659=CARTESIAN_POINT('Ctrl Pts',(-7.031006554992,5.160560801384,1.439705413104));
#41660=CARTESIAN_POINT('Ctrl Pts',(-6.949756554992,3.418696500819,3.479165197693));
#41661=CARTESIAN_POINT('Ctrl Pts',(-6.868506554992,0.7815434040185,3.96793449202));
#41662=CARTESIAN_POINT('Ctrl Pts',(-6.787256554992,-1.575514419506,2.688157587048));
#41663=CARTESIAN_POINT('Ctrl Pts',(-6.706006554992,-2.601856179989,0.2102685806102));
#41664=CARTESIAN_POINT('Ctrl Pts',(-6.624756554992,-1.840261017337,-2.361418873952));
#41665=CARTESIAN_POINT('Ctrl Pts',(-6.543506554992,0.3706726829451,-3.880304137017));
#41666=CARTESIAN_POINT('Ctrl Pts',(-6.489339888326,2.151783524521,-3.740648955836));
#41667=CARTESIAN_POINT('Ctrl Pts',(-6.462256554992,2.922638690214,-3.397442123851));
#41668=CARTESIAN_POINT('Ctrl Pts',(-8.968683552684,-0.8712160753873,3.139824562851));
#41669=CARTESIAN_POINT('Ctrl Pts',(-8.94160021935,-1.583619670625,2.622233053807));
#41670=CARTESIAN_POINT('Ctrl Pts',(-8.887433552684,-2.639201420765,1.08539459674));
#41671=CARTESIAN_POINT('Ctrl Pts',(-8.806183552684,-2.420126412902,-1.705313552873));
#41672=CARTESIAN_POINT('Ctrl Pts',(-8.724933552684,-0.4933130530206,-3.735499168218));
#41673=CARTESIAN_POINT('Ctrl Pts',(-8.643683552684,2.281656159615,-4.100863346074));
#41674=CARTESIAN_POINT('Ctrl Pts',(-8.562433552684,4.668165700744,-2.638407262411));
#41675=CARTESIAN_POINT('Ctrl Pts',(-8.481183552684,5.602472543663,-4.181049654858E-7));
#41676=CARTESIAN_POINT('Ctrl Pts',(-8.399933552684,4.66816370725,2.638408934831));
#41677=CARTESIAN_POINT('Ctrl Pts',(-8.318683552684,2.28166413359,4.100857492604));
#41678=CARTESIAN_POINT('Ctrl Pts',(-8.237433552684,-0.4933429554299,3.735520909677));
#41679=CARTESIAN_POINT('Ctrl Pts',(-8.156183552684,-2.420014777241,1.705232440507));
#41680=CARTESIAN_POINT('Ctrl Pts',(-8.074933552684,-2.639618061001,-1.085091888735));
#41681=CARTESIAN_POINT('Ctrl Pts',(-7.993683552684,-1.054273870273,-3.391782001995));
#41682=CARTESIAN_POINT('Ctrl Pts',(-7.912433552684,1.62941708977,-4.186727480392));
#41683=CARTESIAN_POINT('Ctrl Pts',(-7.831183552684,4.215312080335,-3.11561470445));
#41684=CARTESIAN_POINT('Ctrl Pts',(-7.749933552684,5.550856818033,-0.6558472895843));
#41685=CARTESIAN_POINT('Ctrl Pts',(-7.668683552684,5.040788225852,2.096236559566));
#41686=CARTESIAN_POINT('Ctrl Pts',(-7.587433552684,2.912447995233,3.914010842643));
#41687=CARTESIAN_POINT('Ctrl Pts',(-7.506183552684,0.1144545577098,3.987278879338));
#41688=CARTESIAN_POINT('Ctrl Pts',(-7.424933552684,-2.106103811857,2.283384513961));
#41689=CARTESIAN_POINT('Ctrl Pts',(-7.343683552684,-2.759506312963,-0.4382327725412));
#41690=CARTESIAN_POINT('Ctrl Pts',(-7.262433552684,-1.554526171585,-2.964526172083));
#41691=CARTESIAN_POINT('Ctrl Pts',(-7.181183552684,0.9717672242161,-4.169506314214));
#41692=CARTESIAN_POINT('Ctrl Pts',(-7.099933552684,3.693384526433,-3.516103806355));
#41693=CARTESIAN_POINT('Ctrl Pts',(-7.018683552684,5.39727883269,-1.295545463045));
#41694=CARTESIAN_POINT('Ctrl Pts',(-6.937433552684,5.324011016761,1.502448072752));
#41695=CARTESIAN_POINT('Ctrl Pts',(-6.856183552684,3.506235909742,3.630787936533));
#41696=CARTESIAN_POINT('Ctrl Pts',(-6.774933552684,0.7541551355947,4.140857897789));
#41697=CARTESIAN_POINT('Ctrl Pts',(-6.693683552684,-1.705623755341,2.805308050628));
#41698=CARTESIAN_POINT('Ctrl Pts',(-6.612433552684,-2.776693702003,0.2194321288388));
#41699=CARTESIAN_POINT('Ctrl Pts',(-6.531183552684,-1.981908064657,-2.464329996843));
#41700=CARTESIAN_POINT('Ctrl Pts',(-6.449933552684,0.325378583525,-4.049408593792));
#41701=CARTESIAN_POINT('Ctrl Pts',(-6.395766886017,2.184110603928,-3.903667210934));
#41702=CARTESIAN_POINT('Ctrl Pts',(-6.368683552684,2.988559797162,-3.545503354232));
#41703=CARTESIAN_POINT('Ctrl Pts',(-8.875110550375,-0.9664803087391,3.270944531304));
#41704=CARTESIAN_POINT('Ctrl Pts',(-8.848027217042,-1.708634081117,2.731738253352));
#41705=CARTESIAN_POINT('Ctrl Pts',(-8.793860550375,-2.808297225935,1.130720984389));
#41706=CARTESIAN_POINT('Ctrl Pts',(-8.712610550375,-2.580073583318,-1.776527932779));
#41707=CARTESIAN_POINT('Ctrl Pts',(-8.631360550375,-0.5727959484731,-3.891494677932));
#41708=CARTESIAN_POINT('Ctrl Pts',(-8.550110550375,2.318056769223,-4.272116567967));
#41709=CARTESIAN_POINT('Ctrl Pts',(-8.468860550375,4.804227628837,-2.748587901516));
#41710=CARTESIAN_POINT('Ctrl Pts',(-8.387610550375,5.777551391752,-4.35565146617E-7));
#41711=CARTESIAN_POINT('Ctrl Pts',(-8.306360550375,4.804225552094,2.748589643777));
#41712=CARTESIAN_POINT('Ctrl Pts',(-8.225110550375,2.318065076194,4.272110470055));
#41713=CARTESIAN_POINT('Ctrl Pts',(-8.143860550375,-0.5728270996155,3.89151732732));
#41714=CARTESIAN_POINT('Ctrl Pts',(-8.062610550375,-2.57995728572,1.776443433137));
#41715=CARTESIAN_POINT('Ctrl Pts',(-7.981360550375,-2.808731265186,-1.130405635211));
#41716=CARTESIAN_POINT('Ctrl Pts',(-7.900110550375,-1.157182649303,-3.533423784903));
#41717=CARTESIAN_POINT('Ctrl Pts',(-7.818860550375,1.638580009963,-4.361566413001));
#41718=CARTESIAN_POINT('Ctrl Pts',(-7.737610550375,4.332462712197,-3.245723662317));
#41719=CARTESIAN_POINT('Ctrl Pts',(-7.656360550375,5.723780178711,-0.6832356592843));
#41720=CARTESIAN_POINT('Ctrl Pts',(-7.575110550375,5.192410976774,2.183775995627));
#41721=CARTESIAN_POINT('Ctrl Pts',(-7.493860550375,2.975190651644,4.077461050748));
#41722=CARTESIAN_POINT('Ctrl Pts',(-7.412610550375,0.06035221086774,4.153788781534));
#41723=CARTESIAN_POINT('Ctrl Pts',(-7.331360550375,-2.252937308971,2.378739301925));
#41724=CARTESIAN_POINT('Ctrl Pts',(-7.250110550375,-2.933626084714,-0.4565334979991));
#41725=CARTESIAN_POINT('Ctrl Pts',(-7.168860550375,-1.678325629267,-3.088325629786));
#41726=CARTESIAN_POINT('Ctrl Pts',(-7.087610550375,0.9534664986228,-4.343626086017));
#41727=CARTESIAN_POINT('Ctrl Pts',(-7.006360550375,3.788739314919,-3.662937303239));
#41728=CARTESIAN_POINT('Ctrl Pts',(-6.925110550375,5.563788732938,-1.349647810754));
#41729=CARTESIAN_POINT('Ctrl Pts',(-6.843860550375,5.487461232137,1.5651907324));
#41730=CARTESIAN_POINT('Ctrl Pts',(-6.762610550375,3.593775318665,3.782410675374));
#41731=CARTESIAN_POINT('Ctrl Pts',(-6.681360550375,0.726766867171,4.313781303558));
#41732=CARTESIAN_POINT('Ctrl Pts',(-6.600110550375,-1.835733091177,2.922458514209));
#41733=CARTESIAN_POINT('Ctrl Pts',(-6.518860550375,-2.951531224017,0.2285956770674));
#41734=CARTESIAN_POINT('Ctrl Pts',(-6.437610550375,-2.123555111978,-2.567241119733));
#41735=CARTESIAN_POINT('Ctrl Pts',(-6.356360550375,0.2800844841049,-4.218513050568));
#41736=CARTESIAN_POINT('Ctrl Pts',(-6.302193883708,2.216437683334,-4.066685466031));
#41737=CARTESIAN_POINT('Ctrl Pts',(-6.275110550375,3.05448090411,-3.693564584614));
#41738=CARTESIAN_POINT('',(-7.09950292206828,1.41000000072087,-3.99913898127794));
#41739=CARTESIAN_POINT('Ctrl Pts',(-8.84961610999201,-2.05291292567607,
1.99934460346442));
#41740=CARTESIAN_POINT('Ctrl Pts',(-8.84643469718357,-2.10585184919526,
1.90810351889361));
#41741=CARTESIAN_POINT('Ctrl Pts',(-8.84328515155475,-2.15519371918908,
1.8147745582008));
#41742=CARTESIAN_POINT('Ctrl Pts',(-8.83591275217547,-2.2633832825094,1.58864351247807));
#41743=CARTESIAN_POINT('Ctrl Pts',(-8.8317778322986,-2.31848548620886,1.45490383377774));
#41744=CARTESIAN_POINT('Ctrl Pts',(-8.82247441886724,-2.4255455182645,1.14801103160697));
#41745=CARTESIAN_POINT('Ctrl Pts',(-8.81729234582501,-2.4729511085549,0.974529705226004));
#41746=CARTESIAN_POINT('Ctrl Pts',(-8.80112450537185,-2.57998489333633,
0.442598530957726));
#41747=CARTESIAN_POINT('Ctrl Pts',(-8.78983025833947,-2.60302956037622,
0.077532645670375));
#41748=CARTESIAN_POINT('Ctrl Pts',(-8.77367021457257,-2.56624884193027,
-0.44869507039522));
#41749=CARTESIAN_POINT('Ctrl Pts',(-8.7686466263556,-2.54466145780971,-0.612896922482584));
#41750=CARTESIAN_POINT('Ctrl Pts',(-8.75775263229734,-2.47454393779728,
-0.972005640751989));
#41751=CARTESIAN_POINT('Ctrl Pts',(-8.7520275571852,-2.4214708033906,-1.16480931942071));
#41752=CARTESIAN_POINT('Ctrl Pts',(-8.7421872235292,-2.30471804700921,-1.48946009464062));
#41753=CARTESIAN_POINT('Ctrl Pts',(-8.73805722520744,-2.24844822486328,
-1.62241166452016));
#41754=CARTESIAN_POINT('Ctrl Pts',(-8.72254433148797,-2.01664563597645,
-2.09553806880504));
#41755=CARTESIAN_POINT('Ctrl Pts',(-8.71065560548505,-1.79886466058706,
-2.4143220834137));
#41756=CARTESIAN_POINT('Ctrl Pts',(-8.69365907904848,-1.42570887431899,
-2.82363549841843));
#41757=CARTESIAN_POINT('Ctrl Pts',(-8.68841624212281,-1.30178161453281,
-2.94337585970706));
#41758=CARTESIAN_POINT('Ctrl Pts',(-8.67735221388011,-1.01938028138805,
-3.18302451148001));
#41759=CARTESIAN_POINT('Ctrl Pts',(-8.67165111376055,-0.859279685456863,
-3.2994802782033));
#41760=CARTESIAN_POINT('Ctrl Pts',(-8.66190045517826,-0.568761868358127,
-3.47877777326836));
#41761=CARTESIAN_POINT('Ctrl Pts',(-8.65782410662076,-0.443317057013741,
-3.54706086873473));
#41762=CARTESIAN_POINT('Ctrl Pts',(-8.64132703477721,0.0640327092394041,
-3.7882575867043));
#41763=CARTESIAN_POINT('Ctrl Pts',(-8.62824850589926,0.470640809013835,
-3.90791123447323));
#41764=CARTESIAN_POINT('Ctrl Pts',(-8.61044140350239,1.04713748034553,-3.98502302993153));
#41765=CARTESIAN_POINT('Ctrl Pts',(-8.60548443803191,1.2102545500858,-3.9969078795374));
#41766=CARTESIAN_POINT('Ctrl Pts',(-8.59515651420951,1.55741612539018,-4.00083483168217));
#41767=CARTESIAN_POINT('Ctrl Pts',(-8.5898895028002,1.74049468293642,-3.99015660630172));
#41768=CARTESIAN_POINT('Ctrl Pts',(-8.58056869571077,2.06425917812041,-3.94831799296271));
#41769=CARTESIAN_POINT('Ctrl Pts',(-8.57650147557731,2.20438669944499,-3.92240383461698));
#41770=CARTESIAN_POINT('Ctrl Pts',(-8.56002073851416,2.74983692291422,-3.79040103014612));
#41771=CARTESIAN_POINT('Ctrl Pts',(-8.54694915183239,3.14082122272124,-3.62743044270923));
#41772=CARTESIAN_POINT('Ctrl Pts',(-8.52915529031549,3.63689263990031,-3.32460692390838));
#41773=CARTESIAN_POINT('Ctrl Pts',(-8.52420398753128,3.77095831295386,-3.23125759146068));
#41774=CARTESIAN_POINT('Ctrl Pts',(-8.51389411669355,4.04270443314504,-3.01614686497048));
#41775=CARTESIAN_POINT('Ctrl Pts',(-8.50863879372461,4.17794605317645,-2.89290537102979));
#41776=CARTESIAN_POINT('Ctrl Pts',(-8.49932745081146,4.40301277325326,-2.65690966990474));
#41777=CARTESIAN_POINT('Ctrl Pts',(-8.49525813554999,4.49565973671551,-2.54853493962672));
#41778=CARTESIAN_POINT('Ctrl Pts',(-8.47877701820019,4.83650831458462,-2.10268780431962));
#41779=CARTESIAN_POINT('Ctrl Pts',(-8.46570772144381,5.03779224688927,-1.73004875918671));
#41780=CARTESIAN_POINT('Ctrl Pts',(-8.44791389274035,5.23278312210009,-1.18254251514403));
#41781=CARTESIAN_POINT('Ctrl Pts',(-8.44296082188042,5.27825054675726,-1.02557489464891));
#41782=CARTESIAN_POINT('Ctrl Pts',(-8.43264709904295,5.35410471824543,-0.687268766736908));
#41783=CARTESIAN_POINT('Ctrl Pts',(-8.42738976494414,5.38166207631401,-0.506314523396236));
#41784=CARTESIAN_POINT('Ctrl Pts',(-8.41807628569901,5.40805734092156,-0.181200078776905));
#41785=CARTESIAN_POINT('Ctrl Pts',(-8.41400681584487,5.4118535287336,-0.038669047923537));
#41786=CARTESIAN_POINT('Ctrl Pts',(-8.39752963410245,5.39615862362053,0.52218033981318));
#41787=CARTESIAN_POINT('Ctrl Pts',(-8.38446506662701,5.31812128108418,0.938302420612284));
#41788=CARTESIAN_POINT('Ctrl Pts',(-8.36667436630585,5.12518920830089,1.48642197477676));
#41789=CARTESIAN_POINT('Ctrl Pts',(-8.36172010839471,5.06173943130446,1.63706105192243));
#41790=CARTESIAN_POINT('Ctrl Pts',(-8.35139853909729,4.90769379927833,1.9479521346632));
#41791=CARTESIAN_POINT('Ctrl Pts',(-8.34613505129627,4.81511847895967,2.10611122227327));
#41792=CARTESIAN_POINT('Ctrl Pts',(-8.33681436091682,4.63086025725661,2.37557631433623));
#41793=CARTESIAN_POINT('Ctrl Pts',(-8.33274379702978,4.54407997861189,2.48874957051106));
#41794=CARTESIAN_POINT('Ctrl Pts',(-8.31628231271703,4.17924031072928,2.91426545442384));
#41795=CARTESIAN_POINT('Ctrl Pts',(-8.30323722853692,3.85721688860602,3.1881762018038));
#41796=CARTESIAN_POINT('Ctrl Pts',(-8.28545952434312,3.36281797574608,3.49265111290003));
#41797=CARTESIAN_POINT('Ctrl Pts',(-8.28050056801215,3.21860185244998,3.56989604452081));
#41798=CARTESIAN_POINT('Ctrl Pts',(-8.27015399752479,2.90252714976439,3.71496809787658));
#41799=CARTESIAN_POINT('Ctrl Pts',(-8.2648716942581,2.73042207311042,3.77985135598681));
#41800=CARTESIAN_POINT('Ctrl Pts',(-8.25552815725815,2.4168523873549,3.87344601601425));
#41801=CARTESIAN_POINT('Ctrl Pts',(-8.25145344246759,2.27805406488937,3.90676794863051));
#41802=CARTESIAN_POINT('Ctrl Pts',(-8.23504627533598,1.72859796267692,4.00729376382368));
#41803=CARTESIAN_POINT('Ctrl Pts',(-8.22206902177147,1.30810857964516,4.01761971390415));
#41804=CARTESIAN_POINT('Ctrl Pts',(-8.20433605616193,0.73372767392041,3.94396573773987));
#41805=CARTESIAN_POINT('Ctrl Pts',(-8.19936022590262,0.572500695069959,
3.91329702216157));
#41806=CARTESIAN_POINT('Ctrl Pts',(-8.18892380739151,0.232662762010082,
3.82666841761553));
#41807=CARTESIAN_POINT('Ctrl Pts',(-8.1835739289633,0.055804878837681,3.76800568319578));
#41808=CARTESIAN_POINT('Ctrl Pts',(-8.17414828388991,-0.24931686021425,
3.64199374421524));
#41809=CARTESIAN_POINT('Ctrl Pts',(-8.17005862117415,-0.378491633600513,
3.58018568526668));
#41810=CARTESIAN_POINT('Ctrl Pts',(-8.15385090523078,-0.862176067366126,
3.31524999388456));
#41811=CARTESIAN_POINT('Ctrl Pts',(-8.14112155289688,-1.1896129757399,3.06391314723039));
#41812=CARTESIAN_POINT('Ctrl Pts',(-8.12355106804285,-1.58751208926258,
2.65094746033788));
#41813=CARTESIAN_POINT('Ctrl Pts',(-8.11851185870086,-1.69521545317531,
2.52454464835922));
#41814=CARTESIAN_POINT('Ctrl Pts',(-8.10774692043597,-1.91202275223654,
2.23539747847899));
#41815=CARTESIAN_POINT('Ctrl Pts',(-8.10215212382597,-2.01718949125223,
2.07111639983117));
#41816=CARTESIAN_POINT('Ctrl Pts',(-8.09242214684246,-2.17897934001922,
1.77120100599946));
#41817=CARTESIAN_POINT('Ctrl Pts',(-8.08827176158543,-2.24068067267691,
1.63990604557891));
#41818=CARTESIAN_POINT('Ctrl Pts',(-8.07277346807375,-2.43777648938402,
1.15189321164572));
#41819=CARTESIAN_POINT('Ctrl Pts',(-8.06092748807461,-2.52942794093955,
0.778194848400361));
#41820=CARTESIAN_POINT('Ctrl Pts',(-8.0439329940201,-2.58532310514898,0.227278919275189));
#41821=CARTESIAN_POINT('Ctrl Pts',(-8.0386545985082,-2.59180184588262,0.0539466788231075));
#41822=CARTESIAN_POINT('Ctrl Pts',(-8.02676493514619,-2.58083524313243,
-0.343816479428662));
#41823=CARTESIAN_POINT('Ctrl Pts',(-8.02035871879499,-2.55569647006428,
-0.566535524687872));
#41824=CARTESIAN_POINT('Ctrl Pts',(-8.0095271388049,-2.48102652403134,-0.938235635197529));
#41825=CARTESIAN_POINT('Ctrl Pts',(-8.00508399092669,-2.44177743325494,
-1.08737917292164));
#41826=CARTESIAN_POINT('Ctrl Pts',(-7.99246936242149,-2.30960412619161,
-1.49174308730004));
#41827=CARTESIAN_POINT('Ctrl Pts',(-7.98414661604672,-2.19915574141526,
-1.74055185695866));
#41828=CARTESIAN_POINT('Ctrl Pts',(-7.96641282816883,-1.91427179669719,
-2.24147382111215));
#41829=CARTESIAN_POINT('Ctrl Pts',(-7.95699926375979,-1.73327257169777,
-2.4902085265274));
#41830=CARTESIAN_POINT('Ctrl Pts',(-7.94367664760113,-1.42749794893696,
-2.8222559768075));
#41831=CARTESIAN_POINT('Ctrl Pts',(-7.93950682957255,-1.32326419294921,
-2.92355007450332));
#41832=CARTESIAN_POINT('Ctrl Pts',(-7.92909444821615,-1.04808197102979,
-3.16273656141954));
#41833=CARTESIAN_POINT('Ctrl Pts',(-7.92282961016138,-0.871721932073699,
-3.29180018360956));
#41834=CARTESIAN_POINT('Ctrl Pts',(-7.91104846735441,-0.535623827938592,
-3.49747550084486));
#41835=CARTESIAN_POINT('Ctrl Pts',(-7.9057109061316,-0.380428706964164,
-3.57897918373674));
#41836=CARTESIAN_POINT('Ctrl Pts',(-7.88857829163988,0.129325875921738,
-3.80611417105785));
#41837=CARTESIAN_POINT('Ctrl Pts',(-7.87666038551479,0.501701075827734,
-3.91275031985627));
#41838=CARTESIAN_POINT('Ctrl Pts',(-7.86126248587222,1.02093550287008,-3.98298630746433));
#41839=CARTESIAN_POINT('Ctrl Pts',(-7.85725423808037,1.16073590492058,-3.99430115306265));
#41840=CARTESIAN_POINT('Ctrl Pts',(-7.84749742147575,1.50232643507186,-4.00360908631064));
#41841=CARTESIAN_POINT('Ctrl Pts',(-7.84172746727987,1.70292087807701,-3.99362152230159));
#41842=CARTESIAN_POINT('Ctrl Pts',(-7.83062259574907,2.07207861054924,-3.94695937181635));
#41843=CARTESIAN_POINT('Ctrl Pts',(-7.82542178055052,2.24008519917537,-3.91467830952474));
#41844=CARTESIAN_POINT('Ctrl Pts',(-7.80796444285909,2.79114901220283,-3.7723593348863));
#41845=CARTESIAN_POINT('Ctrl Pts',(-7.7955482729733,3.16267514216532,-3.61589653192316));
#41846=CARTESIAN_POINT('Ctrl Pts',(-7.77974656484461,3.62187610157493,-3.33511324646981));
#41847=CARTESIAN_POINT('Ctrl Pts',(-7.77576926878808,3.73666685794663,-3.25621775732238));
#41848=CARTESIAN_POINT('Ctrl Pts',(-7.76616137317479,4.00347215087133,-3.05116023396499));
#41849=CARTESIAN_POINT('Ctrl Pts',(-7.76050972811701,4.14990634499246,-2.91994128613319));
#41850=CARTESIAN_POINT('Ctrl Pts',(-7.74956344298934,4.40422140540033,-2.65542404049085));
#41851=CARTESIAN_POINT('Ctrl Pts',(-7.74439281601866,4.5140925868034,-2.52550074770107));
#41852=CARTESIAN_POINT('Ctrl Pts',(-7.72686007370345,4.85524575071136,-2.06671020327493));
#41853=CARTESIAN_POINT('Ctrl Pts',(-7.71432915419634,5.04748430892309,-1.70824460230927));
#41854=CARTESIAN_POINT('Ctrl Pts',(-7.69843468145297,5.22844258390508,-1.19784564861864));
#41855=CARTESIAN_POINT('Ctrl Pts',(-7.69446426354047,5.26787075238927,-1.06447768018486));
#41856=CARTESIAN_POINT('Ctrl Pts',(-7.68489100187416,5.34574648758367,-0.738358811855705));
#41857=CARTESIAN_POINT('Ctrl Pts',(-7.67926720125676,5.37680047670683,-0.545206265220628));
#41858=CARTESIAN_POINT('Ctrl Pts',(-7.66835808107404,5.40798735545737,-0.180806195381952));
#41859=CARTESIAN_POINT('Ctrl Pts',(-7.6631944340885,5.41167212919348,-0.0109084292610411));
#41860=CARTESIAN_POINT('Ctrl Pts',(-7.64564410891077,5.38831496683481,0.560947118691117));
#41861=CARTESIAN_POINT('Ctrl Pts',(-7.63308645584631,5.3120322444401,0.961350579724166));
#41862=CARTESIAN_POINT('Ctrl Pts',(-7.61717046027468,5.13113362775074,1.47258037647918));
#41863=CARTESIAN_POINT('Ctrl Pts',(-7.61320169525421,5.07784838133224,1.60098553140313));
#41864=CARTESIAN_POINT('Ctrl Pts',(-7.60363636244069,4.93322578023245,1.90317190361519));
#41865=CARTESIAN_POINT('Ctrl Pts',(-7.5980188583853,4.83591371367482,2.07262712512135));
#41866=CARTESIAN_POINT('Ctrl Pts',(-7.58711818588042,4.63100129230278,2.375233244504));
#41867=CARTESIAN_POINT('Ctrl Pts',(-7.58195616510477,4.52698715077923,2.50955735486238));
#41868=CARTESIAN_POINT('Ctrl Pts',(-7.56440132806299,4.1488985576194,2.93942952767956));
#41869=CARTESIAN_POINT('Ctrl Pts',(-7.55183700381181,3.83748071484364,3.20274145831215));
#41870=CARTESIAN_POINT('Ctrl Pts',(-7.53591553578612,3.37499075557905,3.48627865256812));
#41871=CARTESIAN_POINT('Ctrl Pts',(-7.53194708936957,3.25277819857129,3.55252490237572));
#41872=CARTESIAN_POINT('Ctrl Pts',(-7.52238434054904,2.95029152413514,3.69630262689152));
#41873=CARTESIAN_POINT('Ctrl Pts',(-7.51676910519429,2.76810053092606,3.76672276634242));
#41874=CARTESIAN_POINT('Ctrl Pts',(-7.50587110941699,2.41850472499507,3.87291915771657));
#41875=CARTESIAN_POINT('Ctrl Pts',(-7.50070928331498,2.25314440176428,3.91185336740775));
#41876=CARTESIAN_POINT('Ctrl Pts',(-7.48315412510653,1.68877799028105,4.00800581000016));
#41877=CARTESIAN_POINT('Ctrl Pts',(-7.47058925348492,1.28103513176941,4.01666501820596));
#41878=CARTESIAN_POINT('Ctrl Pts',(-7.4546672235838,0.743155605801197,3.94596580112017));
#41879=CARTESIAN_POINT('Ctrl Pts',(-7.45069871652713,0.606485421942205,
3.92053935865417));
#41880=CARTESIAN_POINT('Ctrl Pts',(-7.44113632603371,0.280935375524862,
3.84192110553983));
#41881=CARTESIAN_POINT('Ctrl Pts',(-7.4355215328099,0.0950404895053442,
3.78199857509237));
#41882=CARTESIAN_POINT('Ctrl Pts',(-7.42462540897175,-0.243425406291763,
3.64455115422927));
#41883=CARTESIAN_POINT('Ctrl Pts',(-7.41946507362647,-0.396396210947056,
3.570771188204));
#41884=CARTESIAN_POINT('Ctrl Pts',(-7.40191019799819,-0.895509931253181,
3.29036186734888));
#41885=CARTESIAN_POINT('Ctrl Pts',(-7.38934378813035,-1.21787775746866,
3.04047992587711));
#41886=CARTESIAN_POINT('Ctrl Pts',(-7.37342249874026,-1.5913904607136,2.6470668369273));
#41887=CARTESIAN_POINT('Ctrl Pts',(-7.36945579441319,-1.68156625222372,
2.54135046778569));
#41888=CARTESIAN_POINT('Ctrl Pts',(-7.35988526470485,-1.88529164648697,
2.27515597070471));
#41889=CARTESIAN_POINT('Ctrl Pts',(-7.35426042843444,-1.99223519290982,
2.11129129683516));
#41890=CARTESIAN_POINT('Ctrl Pts',(-7.34334831524404,-2.16897000334207,
1.79096734915893));
#41891=CARTESIAN_POINT('Ctrl Pts',(-7.33818263269869,-2.24145480846847,
1.6371831953705));
#41892=CARTESIAN_POINT('Ctrl Pts',(-7.32061520538891,-2.45285389888773,
1.10470660786811));
#41893=CARTESIAN_POINT('Ctrl Pts',(-7.30804205117675,-2.54602121212175,
0.707359986720556));
#41894=CARTESIAN_POINT('Ctrl Pts',(-7.29210548837713,-2.58848143003375,
0.166017920341317));
#41895=CARTESIAN_POINT('Ctrl Pts',(-7.28813054711029,-2.59195385365601,
0.0268232157132258));
#41896=CARTESIAN_POINT('Ctrl Pts',(-7.2786095950252,-2.58256970679197,-0.306399647676443));
#41897=CARTESIAN_POINT('Ctrl Pts',(-7.27304288623182,-2.5627955459446,-0.49893328789067));
#41898=CARTESIAN_POINT('Ctrl Pts',(-7.26220556584929,-2.49932381543594,
-0.856657746582581));
#41899=CARTESIAN_POINT('Ctrl Pts',(-7.25705175808226,-2.45914226539997,
-1.02143552756869));
#41900=CARTESIAN_POINT('Ctrl Pts',(-7.23954859536847,-2.28960376308852,
-1.56645372978732));
#41901=CARTESIAN_POINT('Ctrl Pts',(-7.22702922529765,-2.1133726816539,-1.9325863528688));
#41902=CARTESIAN_POINT('Ctrl Pts',(-7.21116533333725,-1.80820099873601,
-2.3787079603919));
#41903=CARTESIAN_POINT('Ctrl Pts',(-7.20721311584906,-1.72408161752784,
-2.48868157581462));
#41904=CARTESIAN_POINT('Ctrl Pts',(-7.19752151294438,-1.50366283508033,
-2.7473125400986));
#41905=CARTESIAN_POINT('Ctrl Pts',(-7.19176142535338,-1.36208549037252,
-2.8896389522497));
#41906=CARTESIAN_POINT('Ctrl Pts',(-7.18071866119574,-1.08172397574098,
-3.13164072702576));
#41907=CARTESIAN_POINT('Ctrl Pts',(-7.17557244423305,-0.946705733537348,
-3.2339897351788));
#41908=CARTESIAN_POINT('Ctrl Pts',(-7.1593907426499,-0.507092836481076,
-3.5260056698966));
#41909=CARTESIAN_POINT('Ctrl Pts',(-7.14821761855518,-0.181767730933443,
-3.68511173709286));
#41910=CARTESIAN_POINT('Ctrl Pts',(-7.13225496889577,0.32742237991983,-3.85413806620003));
#41911=CARTESIAN_POINT('Ctrl Pts',(-7.12715648571192,0.49900937139241,-3.89853576118905));
#41912=CARTESIAN_POINT('Ctrl Pts',(-7.11797189453762,0.814410352902328,
-3.95766919426007));
#41913=CARTESIAN_POINT('Ctrl Pts',(-7.11387693386829,0.956304762310888,
-3.97632621261017));
#41914=CARTESIAN_POINT('Ctrl Pts',(-7.10660144309169,1.20284245916133,-3.99507587614319));
#41915=CARTESIAN_POINT('Ctrl Pts',(-7.10350803129759,1.30643915417203,-3.99886470380827));
#41916=CARTESIAN_POINT('Ctrl Pts',(-7.10038389721637,1.41002651567319,-3.9986428669731));
#41917=CARTESIAN_POINT('',(-6.35049707793183,1.40999999927913,-3.999138981278));
#41918=CARTESIAN_POINT('Ctrl Pts',(-7.10040561164375,1.41002774730112,-3.99860519579024));
#41919=CARTESIAN_POINT('Ctrl Pts',(-7.09264853948305,1.65968390616741,-3.99846447658792));
#41920=CARTESIAN_POINT('Ctrl Pts',(-7.08470884553314,1.90937917061482,-3.97503575881809));
#41921=CARTESIAN_POINT('Ctrl Pts',(-7.07348439443978,2.26828108839417,-3.90720290721754));
#41922=CARTESIAN_POINT('Ctrl Pts',(-7.06998824899606,2.38100516871555,-3.88080332604567));
#41923=CARTESIAN_POINT('Ctrl Pts',(-7.06104116063078,2.67382435338878,-3.79850250412021));
#41924=CARTESIAN_POINT('Ctrl Pts',(-7.055726979142,2.85150016068744,-3.73462977797167));
#41925=CARTESIAN_POINT('Ctrl Pts',(-7.04639135396558,3.15444270784623,-3.60097999533984));
#41926=CARTESIAN_POINT('Ctrl Pts',(-7.04236736848393,3.28198168245327,-3.53637486560756));
#41927=CARTESIAN_POINT('Ctrl Pts',(-7.03507432994842,3.50094605759099,-3.41026339980517));
#41928=CARTESIAN_POINT('Ctrl Pts',(-7.03184207956834,3.5938288091045,-3.35152154680779));
#41929=CARTESIAN_POINT('Ctrl Pts',(-7.02280012435035,3.84006991300434,-3.18104043885625));
#41930=CARTESIAN_POINT('Ctrl Pts',(-7.01686679266736,3.98812095015316,-3.06209221266588));
#41931=CARTESIAN_POINT('Ctrl Pts',(-7.00588507965679,4.24450822583334,-2.82458677088115));
#41932=CARTESIAN_POINT('Ctrl Pts',(-7.0008421448956,4.35547303771764,-2.70879652522094));
#41933=CARTESIAN_POINT('Ctrl Pts',(-6.99233887143207,4.53405647103683,-2.49858968903497));
#41934=CARTESIAN_POINT('Ctrl Pts',(-6.98882592442692,4.60522100925099,-2.40707276472707));
#41935=CARTESIAN_POINT('Ctrl Pts',(-6.98029498517621,4.7724866533641,-2.17124336441763));
#41936=CARTESIAN_POINT('Ctrl Pts',(-6.9753806135466,4.8633994956659,-2.02345584474559));
#41937=CARTESIAN_POINT('Ctrl Pts',(-6.96615565763097,5.01614960889643,-1.73480647039514));
#41938=CARTESIAN_POINT('Ctrl Pts',(-6.96183915945002,5.08011548494544,-1.59508397302638));
#41939=CARTESIAN_POINT('Ctrl Pts',(-6.95415180342381,5.17698644045154,-1.34655178541396));
#41940=CARTESIAN_POINT('Ctrl Pts',(-6.95082544829128,5.21360798629057,-1.23928760181713));
#41941=CARTESIAN_POINT('Ctrl Pts',(-6.94193504283024,5.29679860924318,-0.956414591520403));
#41942=CARTESIAN_POINT('Ctrl Pts',(-6.9362719925443,5.33606680270269,-0.778939748243768));
#41943=CARTESIAN_POINT('Ctrl Pts',(-6.92537916887946,5.38808047222023,-0.435640326624288));
#41944=CARTESIAN_POINT('Ctrl Pts',(-6.92015371441268,5.40280624044388,-0.270070567720667));
#41945=CARTESIAN_POINT('Ctrl Pts',(-6.91140141938467,5.41038251322496,0.0137748843846125));
#41946=CARTESIAN_POINT('Ctrl Pts',(-6.90781775281387,5.40831848296732,0.132006925836137));
#41947=CARTESIAN_POINT('Ctrl Pts',(-6.89902934632707,5.38976170196528,0.429328533989616));
#41948=CARTESIAN_POINT('Ctrl Pts',(-6.89393978297168,5.36638901832164,0.60783464006324));
#41949=CARTESIAN_POINT('Ctrl Pts',(-6.88462602447094,5.30169827724794,0.931350734217961));
#41950=CARTESIAN_POINT('Ctrl Pts',(-6.88039531901273,5.26393730394495,1.07706025500683));
#41951=CARTESIAN_POINT('Ctrl Pts',(-6.87282284039256,5.1838004561804,1.3271752500617));
#41952=CARTESIAN_POINT('Ctrl Pts',(-6.86952325485292,5.14502401023233,1.43263276436424));
#41953=CARTESIAN_POINT('Ctrl Pts',(-6.86058474051734,5.03100590108868,1.70615350829162));
#41954=CARTESIAN_POINT('Ctrl Pts',(-6.85483951679451,4.94852610480644,1.87091019134176));
#41955=CARTESIAN_POINT('Ctrl Pts',(-6.84391930736957,4.77191220217314,2.17066711142937));
#41956=CARTESIAN_POINT('Ctrl Pts',(-6.83874926067223,4.67995002126213,2.30699930816388));
#41957=CARTESIAN_POINT('Ctrl Pts',(-6.83007196160328,4.50851272045314,2.53027683615581));
#41958=CARTESIAN_POINT('Ctrl Pts',(-6.82650914570957,4.43289105125086,2.6202947692206));
#41959=CARTESIAN_POINT('Ctrl Pts',(-6.81755327328165,4.22745669818194,2.84378511200389));
#41960=CARTESIAN_POINT('Ctrl Pts',(-6.81229167157356,4.09197825925759,2.9718348929275));
#41961=CARTESIAN_POINT('Ctrl Pts',(-6.80290679013607,3.83505888724771,3.18288313349167));
#41962=CARTESIAN_POINT('Ctrl Pts',(-6.79877791300063,3.71674561959577,3.26967036479431));
#41963=CARTESIAN_POINT('Ctrl Pts',(-6.79133081516892,3.50058149852532,3.41061310926603));
#41964=CARTESIAN_POINT('Ctrl Pts',(-6.78805166651218,3.40468773490404,3.46754722413532));
#41965=CARTESIAN_POINT('Ctrl Pts',(-6.77849957510682,3.12601985984053,3.61744959952603));
#41966=CARTESIAN_POINT('Ctrl Pts',(-6.77207200824075,2.93822694029586,3.70052768487301));
#41967=CARTESIAN_POINT('Ctrl Pts',(-6.7608990332163,2.60283850902814,3.81935006854174));
#41968=CARTESIAN_POINT('Ctrl Pts',(-6.75615422202189,2.45756574588288,3.8618045463782));
#41969=CARTESIAN_POINT('Ctrl Pts',(-6.74802154077296,2.19982294215036,3.92154433453711));
#41970=CARTESIAN_POINT('Ctrl Pts',(-6.74459021637031,2.08813236287482,3.94247816661047));
#41971=CARTESIAN_POINT('Ctrl Pts',(-6.73577048954965,1.79140335578528,3.98493518026796));
#41972=CARTESIAN_POINT('Ctrl Pts',(-6.73051500342436,1.6054027348797,3.9983293358653));
#41973=CARTESIAN_POINT('Ctrl Pts',(-6.71933816238249,1.20939494222431,3.9992549221185));
#41974=CARTESIAN_POINT('Ctrl Pts',(-6.71341488875577,0.999400629268839,
3.98323814803905));
#41975=CARTESIAN_POINT('Ctrl Pts',(-6.70347327430911,0.668190190731935,
3.93131425303137));
#41976=CARTESIAN_POINT('Ctrl Pts',(-6.69964972193144,0.545364264772287,
3.90603566386308));
#41977=CARTESIAN_POINT('Ctrl Pts',(-6.6900283600526,0.244337374723786,3.82925242751296));
#41978=CARTESIAN_POINT('Ctrl Pts',(-6.6841627211255,0.0678103802409079,
3.77095870914652));
#41979=CARTESIAN_POINT('Ctrl Pts',(-6.67337864743503,-0.251317973649497,
3.64055277063818));
#41980=CARTESIAN_POINT('Ctrl Pts',(-6.66844317053658,-0.395227860993703,
3.57153050297422));
#41981=CARTESIAN_POINT('Ctrl Pts',(-6.66007513270807,-0.639313085021569,
3.4358517989492));
#41982=CARTESIAN_POINT('Ctrl Pts',(-6.65658987000914,-0.741319442714824,
3.37291345569331));
#41983=CARTESIAN_POINT('Ctrl Pts',(-6.64802726253102,-0.988472565784273,
3.20464366323693));
#41984=CARTESIAN_POINT('Ctrl Pts',(-6.64301275132767,-1.12989126015751,
3.09374754301853));
#41985=CARTESIAN_POINT('Ctrl Pts',(-6.6339919336344,-1.36626465943441,2.88129956958178));
#41986=CARTESIAN_POINT('Ctrl Pts',(-6.63001547809971,-1.46446248742735,
2.78337082473436));
#41987=CARTESIAN_POINT('Ctrl Pts',(-6.62218341247131,-1.64141488645966,
2.5873616125255));
#41988=CARTESIAN_POINT('Ctrl Pts',(-6.61835047027259,-1.72110213433034,
2.49017371941394));
#41989=CARTESIAN_POINT('Ctrl Pts',(-6.60868881929315,-1.90734550988093,
2.23997675687712));
#41990=CARTESIAN_POINT('Ctrl Pts',(-6.60279163931173,-2.00823906322116,
2.08268657418761));
#41991=CARTESIAN_POINT('Ctrl Pts',(-6.5922404165828,-2.17026678416869,1.78680482365681));
#41992=CARTESIAN_POINT('Ctrl Pts',(-6.58756310012162,-2.2353280492693,1.65031709481824));
#41993=CARTESIAN_POINT('Ctrl Pts',(-6.57957839978225,-2.33582817755596,
1.40435358487513));
#41994=CARTESIAN_POINT('Ctrl Pts',(-6.57623003568454,-2.37452690980641,
1.29646580053329));
#41995=CARTESIAN_POINT('Ctrl Pts',(-6.56836257095053,-2.45580442423401,
1.03498848397479));
#41996=CARTESIAN_POINT('Ctrl Pts',(-6.56389070096702,-2.49397874547159,
0.880032145100022));
#41997=CARTESIAN_POINT('Ctrl Pts',(-6.55472662491674,-2.55264024750825,
0.56118595528033));
#41998=CARTESIAN_POINT('Ctrl Pts',(-6.55003117462333,-2.57245884526863,
0.397184356979848));
#41999=CARTESIAN_POINT('Ctrl Pts',(-6.54158642076005,-2.58898539341239,
0.112147995876195));
#42000=CARTESIAN_POINT('Ctrl Pts',(-6.53791897762239,-2.59045416366361,
-0.00851120688142535));
#42001=CARTESIAN_POINT('Ctrl Pts',(-6.52894812416622,-2.58091616443174,
-0.298783773648617));
#42002=CARTESIAN_POINT('Ctrl Pts',(-6.52358767827291,-2.56453412952355,
-0.46830403049804));
#42003=CARTESIAN_POINT('Ctrl Pts',(-6.51276365501153,-2.50968827107301,
-0.809199611323964));
#42004=CARTESIAN_POINT('Ctrl Pts',(-6.50730232689531,-2.47053421558778,
-0.980507490960601));
#42005=CARTESIAN_POINT('Ctrl Pts',(-6.49859957075455,-2.38757900086817,
-1.25771032018614));
#42006=CARTESIAN_POINT('Ctrl Pts',(-6.49526864637286,-2.35025216690491,
-1.36528598131246));
#42007=CARTESIAN_POINT('Ctrl Pts',(-6.48751837186656,-2.25110865134264,
-1.6158597727343));
#42008=CARTESIAN_POINT('Ctrl Pts',(-6.4831432271011,-2.18535260593672,-1.75727087972514));
#42009=CARTESIAN_POINT('Ctrl Pts',(-6.47394310377158,-2.03115235522827,
-2.04393838762632));
#42010=CARTESIAN_POINT('Ctrl Pts',(-6.46911221099969,-1.94119644121271,
-2.18836830501301));
#42011=CARTESIAN_POINT('Ctrl Pts',(-6.46059714177034,-1.77364756358404,
-2.42244253864324));
#42012=CARTESIAN_POINT('Ctrl Pts',(-6.45700955059748,-1.70070330793377,
-2.51526801224145));
#42013=CARTESIAN_POINT('Ctrl Pts',(-6.44831688368771,-1.51726468619222,
-2.72864293314367));
#42014=CARTESIAN_POINT('Ctrl Pts',(-6.44315872852927,-1.40306784295126,
-2.84612409470512));
#42015=CARTESIAN_POINT('Ctrl Pts',(-6.43223109663733,-1.14584714399316,
-3.08042436512098));
#42016=CARTESIAN_POINT('Ctrl Pts',(-6.42646797975804,-1.00096605520036,
-3.19527318558294));
#42017=CARTESIAN_POINT('Ctrl Pts',(-6.4175935758287,-0.75789395628627,-3.36186569224979));
#42018=CARTESIAN_POINT('Ctrl Pts',(-6.41436575114532,-0.664555757280254,
-3.4202649657445));
#42019=CARTESIAN_POINT('Ctrl Pts',(-6.40704049248205,-0.443558176644393,
-3.54612460119316));
#42020=CARTESIAN_POINT('Ctrl Pts',(-6.40297937944882,-0.314323736959716,
-3.61071635027914));
#42021=CARTESIAN_POINT('Ctrl Pts',(-6.39365712910819,-0.0110628974216484,
-3.74235727491184));
#42022=CARTESIAN_POINT('Ctrl Pts',(-6.38838974829826,0.165027719985866,
-3.80462796653876));
#42023=CARTESIAN_POINT('Ctrl Pts',(-6.37940441536318,0.458709115427309,
-3.88575132598774));
#42024=CARTESIAN_POINT('Ctrl Pts',(-6.37581931929682,0.574095268851708,
-3.91211444104551));
#42025=CARTESIAN_POINT('Ctrl Pts',(-6.36475154640872,0.927603027900314,
-3.97660210601769));
#42026=CARTESIAN_POINT('Ctrl Pts',(-6.35708770070065,1.16880502641396,-3.99846926139206));
#42027=CARTESIAN_POINT('Ctrl Pts',(-6.34959438835625,1.40997225269887,-3.99860519579024));
#42028=CARTESIAN_POINT('',(-6.5809401104541,1.40999999992274,-3.59999993641013));
#42029=CARTESIAN_POINT('',(-6.580940107676,1.41,-3.6));
#42030=CARTESIAN_POINT('Ctrl Pts',(-9.08096181831227,-1.70608631403884,
1.79907083381568));
#42031=CARTESIAN_POINT('Ctrl Pts',(-9.06844586670953,-1.89532978119226,
1.47248228906589));
#42032=CARTESIAN_POINT('Ctrl Pts',(-9.05389861244493,-2.06808131659788,
1.06106952675657));
#42033=CARTESIAN_POINT('Ctrl Pts',(-9.02143148332091,-2.2174468266351,0.0942360700324087));
#42034=CARTESIAN_POINT('Ctrl Pts',(-9.00581496806962,-2.19733524992031,
-0.385795687504495));
#42035=CARTESIAN_POINT('Ctrl Pts',(-8.97436976361075,-1.97759186945788,
-1.30821422968742));
#42036=CARTESIAN_POINT('Ctrl Pts',(-8.95892749944944,-1.7777422252897,-1.73815589466842));
#42037=CARTESIAN_POINT('Ctrl Pts',(-8.92787976811585,-1.22380952851888,
-2.49313866036759));
#42038=CARTESIAN_POINT('Ctrl Pts',(-8.91259810097365,-0.880327472077836,
-2.81351240010763));
#42039=CARTESIAN_POINT('Ctrl Pts',(-8.87894041754877,-0.0201454942556745,
-3.35073711466932));
#42040=CARTESIAN_POINT('Ctrl Pts',(-8.86328101540959,0.44237879573452,-3.48733627110525));
#42041=CARTESIAN_POINT('Ctrl Pts',(-8.8354748649651,1.27037395437224,-3.62272692428968));
#42042=CARTESIAN_POINT('Ctrl Pts',(-8.82056291466372,1.72790382396507,-3.61408512036349));
#42043=CARTESIAN_POINT('Ctrl Pts',(-8.78981466175988,2.63331213616278,-3.41907230663782));
#42044=CARTESIAN_POINT('Ctrl Pts',(-8.77401256964824,3.07790206736605,-3.22265134720344));
#42045=CARTESIAN_POINT('Ctrl Pts',(-8.74528579717737,3.78929212861787,-2.72756811571601));
#42046=CARTESIAN_POINT('Ctrl Pts',(-8.72998723185347,4.13772490077609,-2.41136229140778));
#42047=CARTESIAN_POINT('Ctrl Pts',(-8.69651879481636,4.68454239160939,-1.56386495711761));
#42048=CARTESIAN_POINT('Ctrl Pts',(-8.68090280181185,4.86168791594835,-1.11730839831426));
#42049=CARTESIAN_POINT('Ctrl Pts',(-8.64945534790638,5.0367005821264,-0.185338695322912));
#42050=CARTESIAN_POINT('Ctrl Pts',(-8.63400985998099,5.02931382570696,0.28881546192218));
#42051=CARTESIAN_POINT('Ctrl Pts',(-8.60295652168341,4.83089760378159,1.20411899127373));
#42052=CARTESIAN_POINT('Ctrl Pts',(-8.58767324940446,4.64768240357197,1.63666659383711));
#42053=CARTESIAN_POINT('Ctrl Pts',(-8.55402240736755,4.08104577128213,2.47750689993866));
#42054=CARTESIAN_POINT('Ctrl Pts',(-8.53836750072557,3.71444438472004,2.79062938894395));
#42055=CARTESIAN_POINT('Ctrl Pts',(-8.51055544369505,3.01325307179545,3.25164727376077));
#42056=CARTESIAN_POINT('Ctrl Pts',(-8.49564682586967,2.59196492057787,3.4300699355234));
#42057=CARTESIAN_POINT('Ctrl Pts',(-8.46490396330893,1.68581697483343,3.62085553562213));
#42058=CARTESIAN_POINT('Ctrl Pts',(-8.44910111676051,1.19975277292987,3.62259872586791));
#42059=CARTESIAN_POINT('Ctrl Pts',(-8.42038172893544,0.348598058934349,
3.46032176848038));
#42060=CARTESIAN_POINT('Ctrl Pts',(-8.40508398769246,-0.0984315066368924,
3.31357798233121));
#42061=CARTESIAN_POINT('Ctrl Pts',(-8.37161360411923,-0.943177717951458,
2.76242525451422));
#42062=CARTESIAN_POINT('Ctrl Pts',(-8.35599554789019,-1.28693865774261,
2.42674063682566));
#42063=CARTESIAN_POINT('Ctrl Pts',(-8.32454904505759,-1.82646306968818,
1.64695414520521));
#42064=CARTESIAN_POINT('Ctrl Pts',(-8.30910652452477,-2.01291298468063,
1.21103527034423));
#42065=CARTESIAN_POINT('Ctrl Pts',(-8.27804979542418,-2.20468934191018,
0.294218193195978));
#42066=CARTESIAN_POINT('Ctrl Pts',(-8.26276355706457,-2.21359613350388,
-0.17554373755032));
#42067=CARTESIAN_POINT('Ctrl Pts',(-8.22911620634852,-2.03870729715697,
-1.17419294066118));
#42068=CARTESIAN_POINT('Ctrl Pts',(-8.21346469756575,-1.83160449981305,
-1.60944010832624));
#42069=CARTESIAN_POINT('Ctrl Pts',(-8.18564692764263,-1.37897885840424,
-2.31628097671549));
#42070=CARTESIAN_POINT('Ctrl Pts',(-8.17074246494018,-1.06701032516302,
-2.65076002294469));
#42071=CARTESIAN_POINT('Ctrl Pts',(-8.14000600973343,-0.317446084704328,
-3.19417423343643));
#42072=CARTESIAN_POINT('Ctrl Pts',(-8.12420228432081,0.125743998114902,
-3.39384267259264));
#42073=CARTESIAN_POINT('Ctrl Pts',(-8.09549084818321,0.968921924879492,
-3.59243206163479));
#42074=CARTESIAN_POINT('Ctrl Pts',(-8.08019418646456,1.43691188026914,-3.64066439324238));
#42075=CARTESIAN_POINT('Ctrl Pts',(-8.04672214409242,2.43299215640587,-3.48167859570911));
#42076=CARTESIAN_POINT('Ctrl Pts',(-8.03110175186132,2.88378118790837,-3.31519900874102));
#42077=CARTESIAN_POINT('Ctrl Pts',(-7.99965634959557,3.69423168855652,-2.82298744252999));
#42078=CARTESIAN_POINT('Ctrl Pts',(-7.98421719987669,4.04210919775715,-2.50100896810475));
#42079=CARTESIAN_POINT('Ctrl Pts',(-7.95315659758425,4.59096715371532,-1.74186823207489));
#42080=CARTESIAN_POINT('Ctrl Pts',(-7.93786697424626,4.79058036633025,-1.31641162082662));
#42081=CARTESIAN_POINT('Ctrl Pts',(-7.90422322792772,5.03780997820345,-0.333276150020889));
#42082=CARTESIAN_POINT('Ctrl Pts',(-7.88857555087737,5.02614425340102,0.148461360209211));
#42083=CARTESIAN_POINT('Ctrl Pts',(-7.86075164923162,4.9008256457112,0.978580261358042));
#42084=CARTESIAN_POINT('Ctrl Pts',(-7.84585197180134,4.75227370220379,1.41101213498212));
#42085=CARTESIAN_POINT('Ctrl Pts',(-7.81602824355066,4.30310920504431,2.1889878650182));
#42086=CARTESIAN_POINT('Ctrl Pts',(-7.80112856612061,4.00288818883333,2.53385355868915));
#42087=CARTESIAN_POINT('Ctrl Pts',(-7.77330466447505,3.34664343612141,3.05744210708992));
#42088=CARTESIAN_POINT('Ctrl Pts',(-7.7576569874249,2.93527937670711,3.30841367623759));
#42089=CARTESIAN_POINT('Ctrl Pts',(-7.72401324110639,1.9602442776905,3.58587428719052));
#42090=CARTESIAN_POINT('Ctrl Pts',(-7.7087236177683,1.4919814378338,3.62573247975904));
#42091=CARTESIAN_POINT('Ctrl Pts',(-7.67766301547583,0.560117297405548,
3.52997791484458));
#42092=CARTESIAN_POINT('Ctrl Pts',(-7.6622238657569,0.107337004481931,3.38969639168412));
#42093=CARTESIAN_POINT('Ctrl Pts',(-7.63077846349124,-0.724155966216571,
2.93393145271847));
#42094=CARTESIAN_POINT('Ctrl Pts',(-7.61515807126026,-1.09372603349347,
2.62677649317388));
#42095=CARTESIAN_POINT('Ctrl Pts',(-7.58168602888828,-1.72945191106649,
1.84363856859722));
#42096=CARTESIAN_POINT('Ctrl Pts',(-7.56638936716971,-1.92167646430538,
1.41423121270979));
#42097=CARTESIAN_POINT('Ctrl Pts',(-7.53767793103207,-2.17128197185495,
0.584723013700023));
#42098=CARTESIAN_POINT('Ctrl Pts',(-7.52187420561931,-2.21995907262114,
0.101074923695193));
#42099=CARTESIAN_POINT('Ctrl Pts',(-7.49113775041247,-2.12413068178685,
-0.819773855556126));
#42100=CARTESIAN_POINT('Ctrl Pts',(-7.47623328771001,-1.99044759733927,
-1.25718605363888));
#42101=CARTESIAN_POINT('Ctrl Pts',(-7.44841551778689,-1.60461826958535,
-2.00259179169766));
#42102=CARTESIAN_POINT('Ctrl Pts',(-7.43276400900423,-1.33123456413401,
-2.39957165922484));
#42103=CARTESIAN_POINT('Ctrl Pts',(-7.39911665828806,-0.553823402944175,
-3.05035443589482));
#42104=CARTESIAN_POINT('Ctrl Pts',(-7.38383041992828,-0.142544241390186,
-3.27752189348148));
#42105=CARTESIAN_POINT('Ctrl Pts',(-7.35277369082752,0.747330816658265,
-3.56984723484916));
#42106=CARTESIAN_POINT('Ctrl Pts',(-7.33733117029458,1.21807259377297,-3.62633630936248));
#42107=CARTESIAN_POINT('Ctrl Pts',(-7.30588466746204,2.16314971101677,-3.5489877084657));
#42108=CARTESIAN_POINT('Ctrl Pts',(-7.29026661123315,2.62574158749036,-3.41912431062187));
#42109=CARTESIAN_POINT('Ctrl Pts',(-7.25679622765995,3.52542695680216,-2.96312899578099));
#42110=CARTESIAN_POINT('Ctrl Pts',(-7.2414984864169,3.87602558624035,-2.64936192882806));
#42111=CARTESIAN_POINT('Ctrl Pts',(-7.21277909859177,4.44213891078422,-1.99337880265077));
#42112=CARTESIAN_POINT('Ctrl Pts',(-7.19697625204333,4.68366136469929,-1.57156326080924));
#42113=CARTESIAN_POINT('Ctrl Pts',(-7.16623338948259,4.97151016120934,-0.691423320158281));
#42114=CARTESIAN_POINT('Ctrl Pts',(-7.15132477165723,5.0276356791207,-0.237365748009261));
#42115=CARTESIAN_POINT('Ctrl Pts',(-7.12351271462668,4.97897813573245,0.6003926843047));
#42116=CARTESIAN_POINT('Ctrl Pts',(-7.10785780798465,4.89110679903859,1.07444004263271));
#42117=CARTESIAN_POINT('Ctrl Pts',(-7.07420696594771,4.44623604957347,1.98558191396118));
#42118=CARTESIAN_POINT('Ctrl Pts',(-7.05892369366876,4.16324643751228,2.36052473298372));
#42119=CARTESIAN_POINT('Ctrl Pts',(-7.02787035537127,3.46977843988283,2.99000998636959));
#42120=CARTESIAN_POINT('Ctrl Pts',(-7.01242486744595,3.06284227260822,3.23348418370285));
#42121=CARTESIAN_POINT('Ctrl Pts',(-6.98097741354077,2.16822650117107,3.54790362030417));
#42122=CARTESIAN_POINT('Ctrl Pts',(-6.96536142053655,1.69292441485119,3.61776937546153));
#42123=CARTESIAN_POINT('Ctrl Pts',(-6.93189298349964,0.685561448299596,
3.56796020431103));
#42124=CARTESIAN_POINT('Ctrl Pts',(-6.91659441817572,0.237502785545008,
3.42431148426496));
#42125=CARTESIAN_POINT('Ctrl Pts',(-6.88786764570467,-0.546946900536641,
3.05577123496467));
#42126=CARTESIAN_POINT('Ctrl Pts',(-6.87206555359276,-0.93934740684421,
2.76895553999292));
#42127=CARTESIAN_POINT('Ctrl Pts',(-6.84131730068868,-1.56093761369266,
2.0823553476949));
#42128=CARTESIAN_POINT('Ctrl Pts',(-6.82640535038721,-1.79718657022345,
1.69044375960059));
#42129=CARTESIAN_POINT('Ctrl Pts',(-6.79859919994262,-2.09393240444934,
0.905683591417754));
#42130=CARTESIAN_POINT('Ctrl Pts',(-6.7829397978034,-2.20689620983523,0.436826228201021));
#42131=CARTESIAN_POINT('Ctrl Pts',(-6.74928211437852,-2.17173694839478,
-0.576725573751296));
#42132=CARTESIAN_POINT('Ctrl Pts',(-6.73400044723635,-2.06602617929488,
-1.0343766302434));
#42133=CARTESIAN_POINT('Ctrl Pts',(-6.70295271590285,-1.6891582731651,-1.89158780048352));
#42134=CARTESIAN_POINT('Ctrl Pts',(-6.68751045174163,-1.41674269123005,
-2.27963350176108));
#42135=CARTESIAN_POINT('Ctrl Pts',(-6.65606524728288,-0.727776491008708,
-2.93114612264656));
#42136=CARTESIAN_POINT('Ctrl Pts',(-6.64044873203163,-0.32211258271571,
-3.18857913776016));
#42137=CARTESIAN_POINT('Ctrl Pts',(-6.60798160501411,0.589872447884793,
-3.54264151700872));
#42138=CARTESIAN_POINT('Ctrl Pts',(-6.59343435231527,1.03254206764506,-3.59874068850377));
#42139=CARTESIAN_POINT('Ctrl Pts',(-6.58091840173488,1.40999774666754,-3.59814532547397));
#42140=CARTESIAN_POINT('Ctrl Pts',(-9.674889449625,-0.9664803087391,3.270944531304));
#42141=CARTESIAN_POINT('Ctrl Pts',(-9.647806116292,-1.708634081117,2.731738253352));
#42142=CARTESIAN_POINT('Ctrl Pts',(-9.593639449625,-2.808297225935,1.130720984389));
#42143=CARTESIAN_POINT('Ctrl Pts',(-9.512389449625,-2.580073583318,-1.776527932779));
#42144=CARTESIAN_POINT('Ctrl Pts',(-9.431139449625,-0.5727959484731,-3.891494677932));
#42145=CARTESIAN_POINT('Ctrl Pts',(-9.349889449625,2.318056769223,-4.272116567967));
#42146=CARTESIAN_POINT('Ctrl Pts',(-9.268639449625,4.804227628837,-2.748587901516));
#42147=CARTESIAN_POINT('Ctrl Pts',(-9.187389449625,5.777551391752,-4.35565146506E-7));
#42148=CARTESIAN_POINT('Ctrl Pts',(-9.106139449625,4.804225552094,2.748589643777));
#42149=CARTESIAN_POINT('Ctrl Pts',(-9.024889449625,2.318065076194,4.272110470055));
#42150=CARTESIAN_POINT('Ctrl Pts',(-8.943639449625,-0.5728270996155,3.89151732732));
#42151=CARTESIAN_POINT('Ctrl Pts',(-8.862389449625,-2.57995728572,1.776443433137));
#42152=CARTESIAN_POINT('Ctrl Pts',(-8.781139449625,-2.808731265186,-1.130405635211));
#42153=CARTESIAN_POINT('Ctrl Pts',(-8.699889449625,-1.157182649303,-3.533423784903));
#42154=CARTESIAN_POINT('Ctrl Pts',(-8.618639449625,1.638580009963,-4.361566413001));
#42155=CARTESIAN_POINT('Ctrl Pts',(-8.537389449625,4.332462712197,-3.245723662317));
#42156=CARTESIAN_POINT('Ctrl Pts',(-8.456139449625,5.723780178711,-0.6832356592843));
#42157=CARTESIAN_POINT('Ctrl Pts',(-8.374889449625,5.192410976774,2.183775995627));
#42158=CARTESIAN_POINT('Ctrl Pts',(-8.293639449625,2.975190651644,4.077461050748));
#42159=CARTESIAN_POINT('Ctrl Pts',(-8.212389449625,0.06035221086774,4.153788781534));
#42160=CARTESIAN_POINT('Ctrl Pts',(-8.131139449625,-2.252937308971,2.378739301925));
#42161=CARTESIAN_POINT('Ctrl Pts',(-8.049889449625,-2.933626084714,-0.4565334979991));
#42162=CARTESIAN_POINT('Ctrl Pts',(-7.968639449625,-1.678325629267,-3.088325629786));
#42163=CARTESIAN_POINT('Ctrl Pts',(-7.887389449625,0.9534664986228,-4.343626086017));
#42164=CARTESIAN_POINT('Ctrl Pts',(-7.806139449625,3.788739314919,-3.662937303239));
#42165=CARTESIAN_POINT('Ctrl Pts',(-7.724889449625,5.563788732938,-1.349647810754));
#42166=CARTESIAN_POINT('Ctrl Pts',(-7.643639449625,5.487461232137,1.5651907324));
#42167=CARTESIAN_POINT('Ctrl Pts',(-7.562389449625,3.593775318665,3.782410675374));
#42168=CARTESIAN_POINT('Ctrl Pts',(-7.481139449625,0.726766867171,4.313781303558));
#42169=CARTESIAN_POINT('Ctrl Pts',(-7.399889449625,-1.835733091177,2.922458514209));
#42170=CARTESIAN_POINT('Ctrl Pts',(-7.318639449625,-2.951531224017,0.2285956770673));
#42171=CARTESIAN_POINT('Ctrl Pts',(-7.237389449625,-2.123555111978,-2.567241119733));
#42172=CARTESIAN_POINT('Ctrl Pts',(-7.156139449625,0.2800844841049,-4.218513050568));
#42173=CARTESIAN_POINT('Ctrl Pts',(-7.101972782958,2.216437683334,-4.066685466031));
#42174=CARTESIAN_POINT('Ctrl Pts',(-7.074889449625,3.05448090411,-3.693564584614));
#42175=CARTESIAN_POINT('Ctrl Pts',(-9.581316447316,-0.8712160753873,3.139824562851));
#42176=CARTESIAN_POINT('Ctrl Pts',(-9.554233113983,-1.583619670625,2.622233053807));
#42177=CARTESIAN_POINT('Ctrl Pts',(-9.500066447316,-2.639201420765,1.08539459674));
#42178=CARTESIAN_POINT('Ctrl Pts',(-9.418816447316,-2.420126412902,-1.705313552873));
#42179=CARTESIAN_POINT('Ctrl Pts',(-9.337566447316,-0.4933130530206,-3.735499168218));
#42180=CARTESIAN_POINT('Ctrl Pts',(-9.256316447316,2.281656159615,-4.100863346074));
#42181=CARTESIAN_POINT('Ctrl Pts',(-9.175066447316,4.668165700744,-2.638407262411));
#42182=CARTESIAN_POINT('Ctrl Pts',(-9.093816447316,5.602472543663,-4.181049656672E-7));
#42183=CARTESIAN_POINT('Ctrl Pts',(-9.012566447316,4.66816370725,2.638408934831));
#42184=CARTESIAN_POINT('Ctrl Pts',(-8.931316447316,2.28166413359,4.100857492604));
#42185=CARTESIAN_POINT('Ctrl Pts',(-8.850066447316,-0.4933429554299,3.735520909677));
#42186=CARTESIAN_POINT('Ctrl Pts',(-8.768816447316,-2.420014777241,1.705232440507));
#42187=CARTESIAN_POINT('Ctrl Pts',(-8.687566447316,-2.639618061001,-1.085091888735));
#42188=CARTESIAN_POINT('Ctrl Pts',(-8.606316447316,-1.054273870273,-3.391782001995));
#42189=CARTESIAN_POINT('Ctrl Pts',(-8.525066447316,1.62941708977,-4.186727480392));
#42190=CARTESIAN_POINT('Ctrl Pts',(-8.443816447316,4.215312080335,-3.11561470445));
#42191=CARTESIAN_POINT('Ctrl Pts',(-8.362566447316,5.550856818033,-0.6558472895843));
#42192=CARTESIAN_POINT('Ctrl Pts',(-8.281316447316,5.040788225852,2.096236559566));
#42193=CARTESIAN_POINT('Ctrl Pts',(-8.200066447316,2.912447995233,3.914010842643));
#42194=CARTESIAN_POINT('Ctrl Pts',(-8.118816447316,0.1144545577098,3.987278879338));
#42195=CARTESIAN_POINT('Ctrl Pts',(-8.037566447316,-2.106103811857,2.283384513961));
#42196=CARTESIAN_POINT('Ctrl Pts',(-7.956316447316,-2.759506312963,-0.4382327725412));
#42197=CARTESIAN_POINT('Ctrl Pts',(-7.875066447316,-1.554526171585,-2.964526172083));
#42198=CARTESIAN_POINT('Ctrl Pts',(-7.793816447316,0.9717672242161,-4.169506314214));
#42199=CARTESIAN_POINT('Ctrl Pts',(-7.712566447316,3.693384526433,-3.516103806355));
#42200=CARTESIAN_POINT('Ctrl Pts',(-7.631316447316,5.39727883269,-1.295545463045));
#42201=CARTESIAN_POINT('Ctrl Pts',(-7.550066447316,5.324011016761,1.502448072752));
#42202=CARTESIAN_POINT('Ctrl Pts',(-7.468816447316,3.506235909742,3.630787936533));
#42203=CARTESIAN_POINT('Ctrl Pts',(-7.387566447316,0.7541551355947,4.140857897789));
#42204=CARTESIAN_POINT('Ctrl Pts',(-7.306316447316,-1.705623755341,2.805308050628));
#42205=CARTESIAN_POINT('Ctrl Pts',(-7.225066447316,-2.776693702003,0.2194321288388));
#42206=CARTESIAN_POINT('Ctrl Pts',(-7.143816447316,-1.981908064657,-2.464329996843));
#42207=CARTESIAN_POINT('Ctrl Pts',(-7.062566447316,0.325378583525,-4.049408593792));
#42208=CARTESIAN_POINT('Ctrl Pts',(-7.00839978065,2.184110603928,-3.903667210934));
#42209=CARTESIAN_POINT('Ctrl Pts',(-6.981316447316,2.988559797162,-3.545503354232));
#42210=CARTESIAN_POINT('Ctrl Pts',(-9.487743445008,-0.7759518420355,3.008704594398));
#42211=CARTESIAN_POINT('Ctrl Pts',(-9.460660111674,-1.458605260133,2.512727854262));
#42212=CARTESIAN_POINT('Ctrl Pts',(-9.406493445008,-2.470105615594,1.040068209092));
#42213=CARTESIAN_POINT('Ctrl Pts',(-9.325243445008,-2.260179242486,-1.634099172968));
#42214=CARTESIAN_POINT('Ctrl Pts',(-9.243993445008,-0.4138301575682,-3.579503658505));
#42215=CARTESIAN_POINT('Ctrl Pts',(-9.162743445008,2.245255550006,-3.929610124181));
#42216=CARTESIAN_POINT('Ctrl Pts',(-9.081493445008,4.532103772651,-2.528226623306));
#42217=CARTESIAN_POINT('Ctrl Pts',(-9.000243445008,5.427393695574,-4.006447743584E-7));
#42218=CARTESIAN_POINT('Ctrl Pts',(-8.918993445008,4.532101862406,2.528228225885));
#42219=CARTESIAN_POINT('Ctrl Pts',(-8.837743445008,2.245263190987,3.929604515154));
#42220=CARTESIAN_POINT('Ctrl Pts',(-8.756493445008,-0.4138588112444,3.579524492034));
#42221=CARTESIAN_POINT('Ctrl Pts',(-8.675243445008,-2.260072268762,1.634021447877));
#42222=CARTESIAN_POINT('Ctrl Pts',(-8.593993445008,-2.470504856815,-1.039778142259));
#42223=CARTESIAN_POINT('Ctrl Pts',(-8.512743445008,-0.9513650912439,-3.250140219087));
#42224=CARTESIAN_POINT('Ctrl Pts',(-8.431493445008,1.620254169577,-4.011888547782));
#42225=CARTESIAN_POINT('Ctrl Pts',(-8.350243445008,4.098161448473,-2.985505746582));
#42226=CARTESIAN_POINT('Ctrl Pts',(-8.268993445008,5.377933457354,-0.6284589198844));
#42227=CARTESIAN_POINT('Ctrl Pts',(-8.187743445008,4.88916547493,2.008697123506));
#42228=CARTESIAN_POINT('Ctrl Pts',(-8.106493445008,2.849705338822,3.750560634537));
#42229=CARTESIAN_POINT('Ctrl Pts',(-8.025243445008,0.1685569045517,3.820768977142));
#42230=CARTESIAN_POINT('Ctrl Pts',(-7.943993445008,-1.959270314743,2.188029725996));
#42231=CARTESIAN_POINT('Ctrl Pts',(-7.862743445008,-2.585386541213,-0.4199320470833));
#42232=CARTESIAN_POINT('Ctrl Pts',(-7.781493445008,-1.430726713904,-2.840726714381));
#42233=CARTESIAN_POINT('Ctrl Pts',(-7.700243445008,0.9900679498094,-3.995386542412));
#42234=CARTESIAN_POINT('Ctrl Pts',(-7.618993445008,3.598029737948,-3.369270309471));
#42235=CARTESIAN_POINT('Ctrl Pts',(-7.537743445008,5.230768932443,-1.241443115336));
#42236=CARTESIAN_POINT('Ctrl Pts',(-7.456493445008,5.160560801384,1.439705413104));
#42237=CARTESIAN_POINT('Ctrl Pts',(-7.375243445008,3.418696500819,3.479165197693));
#42238=CARTESIAN_POINT('Ctrl Pts',(-7.293993445008,0.7815434040185,3.96793449202));
#42239=CARTESIAN_POINT('Ctrl Pts',(-7.212743445008,-1.575514419506,2.688157587048));
#42240=CARTESIAN_POINT('Ctrl Pts',(-7.131493445008,-2.601856179989,0.2102685806102));
#42241=CARTESIAN_POINT('Ctrl Pts',(-7.050243445008,-1.840261017337,-2.361418873952));
#42242=CARTESIAN_POINT('Ctrl Pts',(-6.968993445008,0.3706726829451,-3.880304137017));
#42243=CARTESIAN_POINT('Ctrl Pts',(-6.914826778341,2.151783524521,-3.740648955836));
#42244=CARTESIAN_POINT('Ctrl Pts',(-6.887743445008,2.922638690214,-3.397442123851));
#42245=CARTESIAN_POINT('Ctrl Pts',(-9.394170442699,-0.6806876086837,2.877584625945));
#42246=CARTESIAN_POINT('Ctrl Pts',(-9.367087109366,-1.333590849641,2.403222654717));
#42247=CARTESIAN_POINT('Ctrl Pts',(-9.312920442699,-2.301009810423,0.9947418214436));
#42248=CARTESIAN_POINT('Ctrl Pts',(-9.231670442699,-2.10023207207,-1.562884793063));
#42249=CARTESIAN_POINT('Ctrl Pts',(-9.150420442699,-0.3343472621158,-3.423508148791));
#42250=CARTESIAN_POINT('Ctrl Pts',(-9.069170442699,2.208854940398,-3.758356902288));
#42251=CARTESIAN_POINT('Ctrl Pts',(-8.987920442699,4.396041844558,-2.418045984201));
#42252=CARTESIAN_POINT('Ctrl Pts',(-8.906670442699,5.252314847485,-3.831845932778E-7));
#42253=CARTESIAN_POINT('Ctrl Pts',(-8.825420442699,4.396040017561,2.418047516939));
#42254=CARTESIAN_POINT('Ctrl Pts',(-8.744170442699,2.208862248383,3.758351537704));
#42255=CARTESIAN_POINT('Ctrl Pts',(-8.662920442699,-0.3343746670588,3.423528074391));
#42256=CARTESIAN_POINT('Ctrl Pts',(-8.581670442699,-2.100129760283,1.562810455248));
#42257=CARTESIAN_POINT('Ctrl Pts',(-8.500420442699,-2.301391652629,-0.9944643957835));
#42258=CARTESIAN_POINT('Ctrl Pts',(-8.419170442699,-0.8484563122144,-3.108498436179));
#42259=CARTESIAN_POINT('Ctrl Pts',(-8.337920442699,1.611091249384,-3.837049615173));
#42260=CARTESIAN_POINT('Ctrl Pts',(-8.256670442699,3.981010816611,-2.855396788715));
#42261=CARTESIAN_POINT('Ctrl Pts',(-8.175420442699,5.205010096676,-0.6010705501845));
#42262=CARTESIAN_POINT('Ctrl Pts',(-8.094170442699,4.737542724007,1.921157687446));
#42263=CARTESIAN_POINT('Ctrl Pts',(-8.012920442699,2.786962682412,3.587110426432));
#42264=CARTESIAN_POINT('Ctrl Pts',(-7.931670442699,0.2226592513938,3.654259074947));
#42265=CARTESIAN_POINT('Ctrl Pts',(-7.850420442699,-1.812436817629,2.092674938032));
#42266=CARTESIAN_POINT('Ctrl Pts',(-7.769170442699,-2.411266769463,-0.4016313216255));
#42267=CARTESIAN_POINT('Ctrl Pts',(-7.687920442699,-1.306927256222,-2.716927256679));
#42268=CARTESIAN_POINT('Ctrl Pts',(-7.606670442699,1.008368675403,-3.821266770609));
#42269=CARTESIAN_POINT('Ctrl Pts',(-7.525420442699,3.502674949463,-3.222436812587));
#42270=CARTESIAN_POINT('Ctrl Pts',(-7.444170442699,5.064259032195,-1.187340767628));
#42271=CARTESIAN_POINT('Ctrl Pts',(-7.362920442699,4.997110586008,1.376962753456));
#42272=CARTESIAN_POINT('Ctrl Pts',(-7.281670442699,3.331157091895,3.327542458853));
#42273=CARTESIAN_POINT('Ctrl Pts',(-7.200420442699,0.8089316724422,3.795011086251));
#42274=CARTESIAN_POINT('Ctrl Pts',(-7.119170442699,-1.445405083671,2.571007123468));
#42275=CARTESIAN_POINT('Ctrl Pts',(-7.037920442699,-2.427018657974,0.2011050323817));
#42276=CARTESIAN_POINT('Ctrl Pts',(-6.956670442699,-1.698613970016,-2.258507751061));
#42277=CARTESIAN_POINT('Ctrl Pts',(-6.875420442699,0.4159667823653,-3.711199680242));
#42278=CARTESIAN_POINT('Ctrl Pts',(-6.821253776032,2.119456445115,-3.577630700739));
#42279=CARTESIAN_POINT('Ctrl Pts',(-6.794170442699,2.856717583266,-3.24938089347));
#42280=CARTESIAN_POINT('',(-6.86905988805729,1.40999999992759,-3.59999993640925));
#42281=CARTESIAN_POINT('Ctrl Pts',(-9.36908159826537,-1.70608638503483,
1.79907071129373));
#42282=CARTESIAN_POINT('Ctrl Pts',(-9.35656564768497,-1.89532982405453,
1.47248218597209));
#42283=CARTESIAN_POINT('Ctrl Pts',(-9.3420183949866,-2.06808132628875,1.06106946402822));
#42284=CARTESIAN_POINT('Ctrl Pts',(-9.30955126796911,-2.2174468266351,0.0942360700323995));
#42285=CARTESIAN_POINT('Ctrl Pts',(-9.29393475271798,-2.19733524992031,
-0.385795687504502));
#42286=CARTESIAN_POINT('Ctrl Pts',(-9.26248954825925,-1.97759186945788,
-1.30821422968742));
#42287=CARTESIAN_POINT('Ctrl Pts',(-9.24704728409788,-1.7777422252897,-1.73815589466842));
#42288=CARTESIAN_POINT('Ctrl Pts',(-9.2159995527642,-1.22380952851887,-2.4931386603676));
#42289=CARTESIAN_POINT('Ctrl Pts',(-9.2007178856219,-0.880327472077824,
-2.81351240010764));
#42290=CARTESIAN_POINT('Ctrl Pts',(-9.16706020219686,-0.0201454942556584,
-3.35073711466933));
#42291=CARTESIAN_POINT('Ctrl Pts',(-9.15140080005762,0.44237879573454,-3.48733627110526));
#42292=CARTESIAN_POINT('Ctrl Pts',(-9.12359464961302,1.27037395437227,-3.62272692428968));
#42293=CARTESIAN_POINT('Ctrl Pts',(-9.10868269931163,1.7279038239651,-3.61408512036349));
#42294=CARTESIAN_POINT('Ctrl Pts',(-9.07793444640764,2.63331213616281,-3.41907230663781));
#42295=CARTESIAN_POINT('Ctrl Pts',(-9.06213235429575,3.07790206736608,-3.22265134720342));
#42296=CARTESIAN_POINT('Ctrl Pts',(-9.03340558182475,3.78929212861789,-2.72756811571599));
#42297=CARTESIAN_POINT('Ctrl Pts',(-9.01810701650085,4.13772490077611,-2.41136229140776));
#42298=CARTESIAN_POINT('Ctrl Pts',(-8.98463857946408,4.6845423916094,-1.56386495711759));
#42299=CARTESIAN_POINT('Ctrl Pts',(-8.96902258646002,4.86168791594835,-1.11730839831426));
#42300=CARTESIAN_POINT('Ctrl Pts',(-8.93757513255501,5.0367005821264,-0.185338695322908));
#42301=CARTESIAN_POINT('Ctrl Pts',(-8.92212964462973,5.02931382570696,0.288815461922182));
#42302=CARTESIAN_POINT('Ctrl Pts',(-8.89107630633225,4.83089760378159,1.20411899127373));
#42303=CARTESIAN_POINT('Ctrl Pts',(-8.87579303405328,4.64768240357197,1.63666659383711));
#42304=CARTESIAN_POINT('Ctrl Pts',(-8.84214219201624,4.08104577128213,2.47750689993866));
#42305=CARTESIAN_POINT('Ctrl Pts',(-8.82648728537404,3.71444438472003,2.79062938894396));
#42306=CARTESIAN_POINT('Ctrl Pts',(-8.79867522834333,3.01325307179544,3.25164727376078));
#42307=CARTESIAN_POINT('Ctrl Pts',(-8.78376661051786,2.59196492057786,3.4300699355234));
#42308=CARTESIAN_POINT('Ctrl Pts',(-8.75302374795712,1.68581697483343,3.62085553562213));
#42309=CARTESIAN_POINT('Ctrl Pts',(-8.73722090140883,1.19975277292987,3.62259872586791));
#42310=CARTESIAN_POINT('Ctrl Pts',(-8.70850151358385,0.348598058934352,
3.46032176848038));
#42311=CARTESIAN_POINT('Ctrl Pts',(-8.69320377234091,-0.0984315066368902,
3.31357798233121));
#42312=CARTESIAN_POINT('Ctrl Pts',(-8.65973338876775,-0.943177717951456,
2.76242525451423));
#42313=CARTESIAN_POINT('Ctrl Pts',(-8.64411533253879,-1.28693865774261,
2.42674063682566));
#42314=CARTESIAN_POINT('Ctrl Pts',(-8.61266882970619,-1.82646306968818,
1.64695414520521));
#42315=CARTESIAN_POINT('Ctrl Pts',(-8.59722630917321,-2.01291298468063,
1.21103527034422));
#42316=CARTESIAN_POINT('Ctrl Pts',(-8.56616958007247,-2.20468934191018,
0.294218193195971));
#42317=CARTESIAN_POINT('Ctrl Pts',(-8.55088334171275,-2.21359613350388,
-0.175543737550325));
#42318=CARTESIAN_POINT('Ctrl Pts',(-8.51723599099668,-2.03870729715697,
-1.17419294066118));
#42319=CARTESIAN_POINT('Ctrl Pts',(-8.50158448221408,-1.83160449981305,
-1.60944010832624));
#42320=CARTESIAN_POINT('Ctrl Pts',(-8.47376671229103,-1.37897885840423,
-2.31628097671549));
#42321=CARTESIAN_POINT('Ctrl Pts',(-8.4588622495886,-1.06701032516302,-2.65076002294469));
#42322=CARTESIAN_POINT('Ctrl Pts',(-8.42812579438174,-0.317446084704319,
-3.19417423343644));
#42323=CARTESIAN_POINT('Ctrl Pts',(-8.41232206896895,0.125743998114912,
-3.39384267259265));
#42324=CARTESIAN_POINT('Ctrl Pts',(-8.38361063283124,0.968921924879503,
-3.59243206163479));
#42325=CARTESIAN_POINT('Ctrl Pts',(-8.36831397111268,1.43691188026915,-3.64066439324238));
#42326=CARTESIAN_POINT('Ctrl Pts',(-8.3348419287405,2.4329921564059,-3.48167859570911));
#42327=CARTESIAN_POINT('Ctrl Pts',(-8.31922153650926,2.88378118790839,-3.31519900874101));
#42328=CARTESIAN_POINT('Ctrl Pts',(-8.2877761342433,3.69423168855654,-2.82298744252997));
#42329=CARTESIAN_POINT('Ctrl Pts',(-8.27233698452426,4.04210919775717,-2.50100896810474));
#42330=CARTESIAN_POINT('Ctrl Pts',(-8.24127638223185,4.59096715371533,-1.74186823207487));
#42331=CARTESIAN_POINT('Ctrl Pts',(-8.22598675889404,4.79058036633025,-1.31641162082661));
#42332=CARTESIAN_POINT('Ctrl Pts',(-8.19234301257582,5.03780997820345,-0.333276150020885));
#42333=CARTESIAN_POINT('Ctrl Pts',(-8.17669533552577,5.02614425340102,0.148461360209209));
#42334=CARTESIAN_POINT('Ctrl Pts',(-8.1488714338802,4.9008256457112,0.97858026135804));
#42335=CARTESIAN_POINT('Ctrl Pts',(-8.13397175644994,4.75227370220379,1.41101213498212));
#42336=CARTESIAN_POINT('Ctrl Pts',(-8.10414802819902,4.3031092050443,2.1889878650182));
#42337=CARTESIAN_POINT('Ctrl Pts',(-8.08924835076851,4.00288818883332,2.53385355868917));
#42338=CARTESIAN_POINT('Ctrl Pts',(-8.0614244491227,3.34664343612139,3.05744210708993));
#42339=CARTESIAN_POINT('Ctrl Pts',(-8.0457767720724,2.93527937670709,3.3084136762376));
#42340=CARTESIAN_POINT('Ctrl Pts',(-8.01213302575411,1.96024427769048,3.58587428719052));
#42341=CARTESIAN_POINT('Ctrl Pts',(-7.99684340241638,1.49198143783378,3.62573247975904));
#42342=CARTESIAN_POINT('Ctrl Pts',(-7.96578280012404,0.560117297405531,
3.52997791484458));
#42343=CARTESIAN_POINT('Ctrl Pts',(-7.95034365040512,0.107337004481917,
3.38969639168411));
#42344=CARTESIAN_POINT('Ctrl Pts',(-7.91889824813912,-0.724155966216583,
2.93393145271846));
#42345=CARTESIAN_POINT('Ctrl Pts',(-7.90327785590776,-1.09372603349349,
2.62677649317387));
#42346=CARTESIAN_POINT('Ctrl Pts',(-7.8698058135354,-1.7294519110665,1.8436385685972));
#42347=CARTESIAN_POINT('Ctrl Pts',(-7.85450915181672,-1.9216764643054,1.41423121270976));
#42348=CARTESIAN_POINT('Ctrl Pts',(-7.82579771567903,-2.17128197185496,
0.584723013699983));
#42349=CARTESIAN_POINT('Ctrl Pts',(-7.80999399026637,-2.21995907262114,
0.101074923695152));
#42350=CARTESIAN_POINT('Ctrl Pts',(-7.77925753505961,-2.12413068178684,
-0.819773855556165));
#42351=CARTESIAN_POINT('Ctrl Pts',(-7.76435307235719,-1.99044759733926,
-1.25718605363892));
#42352=CARTESIAN_POINT('Ctrl Pts',(-7.73653530243412,-1.60461826958533,
-2.00259179169769));
#42353=CARTESIAN_POINT('Ctrl Pts',(-7.72088379365142,-1.33123456413399,
-2.39957165922486));
#42354=CARTESIAN_POINT('Ctrl Pts',(-7.68723644293545,-0.553823402944156,
-3.05035443589483));
#42355=CARTESIAN_POINT('Ctrl Pts',(-7.67195020457591,-0.142544241390169,
-3.27752189348149));
#42356=CARTESIAN_POINT('Ctrl Pts',(-7.64089347547534,0.747330816658283,
-3.56984723484916));
#42357=CARTESIAN_POINT('Ctrl Pts',(-7.62545095494251,1.21807259377298,-3.62633630936248));
#42358=CARTESIAN_POINT('Ctrl Pts',(-7.59400445210985,2.16314971101678,-3.5489877084657));
#42359=CARTESIAN_POINT('Ctrl Pts',(-7.57838639588073,2.62574158749038,-3.41912431062186));
#42360=CARTESIAN_POINT('Ctrl Pts',(-7.54491601230753,3.52542695680217,-2.96312899578098));
#42361=CARTESIAN_POINT('Ctrl Pts',(-7.52961827106464,3.87602558624036,-2.64936192882806));
#42362=CARTESIAN_POINT('Ctrl Pts',(-7.50089888323972,4.44213891078422,-1.99337880265076));
#42363=CARTESIAN_POINT('Ctrl Pts',(-7.48509603669147,4.68366136469929,-1.57156326080923));
#42364=CARTESIAN_POINT('Ctrl Pts',(-7.45435317413076,4.97151016120934,-0.691423320158279));
#42365=CARTESIAN_POINT('Ctrl Pts',(-7.43944455630529,5.0276356791207,-0.237365748009259));
#42366=CARTESIAN_POINT('Ctrl Pts',(-7.41163249927462,4.97897813573245,0.600392684304703));
#42367=CARTESIAN_POINT('Ctrl Pts',(-7.39597759263248,4.89110679903858,1.07444004263272));
#42368=CARTESIAN_POINT('Ctrl Pts',(-7.36232675059545,4.44623604957346,1.98558191396119));
#42369=CARTESIAN_POINT('Ctrl Pts',(-7.34704347831648,4.16324643751228,2.36052473298373));
#42370=CARTESIAN_POINT('Ctrl Pts',(-7.31599014001889,3.46977843988281,2.99000998636961));
#42371=CARTESIAN_POINT('Ctrl Pts',(-7.30054465209352,3.06284227260819,3.23348418370286));
#42372=CARTESIAN_POINT('Ctrl Pts',(-7.2690971981882,2.16822650117104,3.54790362030417));
#42373=CARTESIAN_POINT('Ctrl Pts',(-7.25348120518384,1.69292441485116,3.61776937546153));
#42374=CARTESIAN_POINT('Ctrl Pts',(-7.22001276814687,0.685561448299564,
3.56796020431102));
#42375=CARTESIAN_POINT('Ctrl Pts',(-7.20471420282298,0.237502785544977,
3.42431148426495));
#42376=CARTESIAN_POINT('Ctrl Pts',(-7.17598743035216,-0.546946900536664,
3.05577123496466));
#42377=CARTESIAN_POINT('Ctrl Pts',(-7.16018533824052,-0.939347406844226,
2.76895553999291));
#42378=CARTESIAN_POINT('Ctrl Pts',(-7.12943708533679,-1.56093761369267,
2.08235534769489));
#42379=CARTESIAN_POINT('Ctrl Pts',(-7.11452513503551,-1.79718657022345,
1.69044375960058));
#42380=CARTESIAN_POINT('Ctrl Pts',(-7.08671898459106,-2.09393240444935,
0.905683591417752));
#42381=CARTESIAN_POINT('Ctrl Pts',(-7.07105958245186,-2.20689620983523,
0.436826228201019));
#42382=CARTESIAN_POINT('Ctrl Pts',(-7.03740189902686,-2.17173694839478,
-0.5767255737513));
#42383=CARTESIAN_POINT('Ctrl Pts',(-7.02212023188454,-2.06602617929488,
-1.03437663024341));
#42384=CARTESIAN_POINT('Ctrl Pts',(-6.99107250055076,-1.68915827316509,
-1.89158780048353));
#42385=CARTESIAN_POINT('Ctrl Pts',(-6.97563023638929,-1.41674269123004,
-2.27963350176109));
#42386=CARTESIAN_POINT('Ctrl Pts',(-6.94418503193041,-0.727776491008685,
-2.93114612264658));
#42387=CARTESIAN_POINT('Ctrl Pts',(-6.92856851667922,-0.322112582715683,
-3.18857913776017));
#42388=CARTESIAN_POINT('Ctrl Pts',(-6.89610138755526,0.589872507054565,
-3.54264153998035));
#42389=CARTESIAN_POINT('Ctrl Pts',(-6.8815541332902,1.03254217835801,-3.59874070293085));
#42390=CARTESIAN_POINT('Ctrl Pts',(-6.86903818168747,1.40999788827261,-3.59814532525062));
#42391=CARTESIAN_POINT('',(-7.1,1.41,-4.));
#42392=CARTESIAN_POINT('Ctrl Pts',(-7.174889449625,-0.2344809041097,-3.693564584614));
#42393=CARTESIAN_POINT('Ctrl Pts',(-7.147806116292,0.6035623166656,-4.066685466031));
#42394=CARTESIAN_POINT('Ctrl Pts',(-7.093639449625,2.539915515895,-4.218513050568));
#42395=CARTESIAN_POINT('Ctrl Pts',(-7.012389449625,4.943555111978,-2.567241119733));
#42396=CARTESIAN_POINT('Ctrl Pts',(-6.931139449625,5.771531224017,0.2285956770673));
#42397=CARTESIAN_POINT('Ctrl Pts',(-6.849889449625,4.655733091177,2.922458514209));
#42398=CARTESIAN_POINT('Ctrl Pts',(-6.768639449625,2.093233132829,4.313781303558));
#42399=CARTESIAN_POINT('Ctrl Pts',(-6.687389449625,-0.7737753186654,3.782410675374));
#42400=CARTESIAN_POINT('Ctrl Pts',(-6.606139449625,-2.667461232137,1.5651907324));
#42401=CARTESIAN_POINT('Ctrl Pts',(-6.524889449625,-2.743788732938,-1.349647810754));
#42402=CARTESIAN_POINT('Ctrl Pts',(-6.443639449625,-0.9687393149189,-3.662937303239));
#42403=CARTESIAN_POINT('Ctrl Pts',(-6.362389449625,1.866533501377,-4.343626086017));
#42404=CARTESIAN_POINT('Ctrl Pts',(-6.281139449625,4.498325629267,-3.088325629786));
#42405=CARTESIAN_POINT('Ctrl Pts',(-6.199889449625,5.753626084714,-0.4565334979991));
#42406=CARTESIAN_POINT('Ctrl Pts',(-6.118639449625,5.072937308971,2.378739301925));
#42407=CARTESIAN_POINT('Ctrl Pts',(-6.037389449625,2.759647789132,4.153788781534));
#42408=CARTESIAN_POINT('Ctrl Pts',(-5.956139449625,-0.155190651644,4.077461050748));
#42409=CARTESIAN_POINT('Ctrl Pts',(-5.874889449625,-2.372410976774,2.183775995627));
#42410=CARTESIAN_POINT('Ctrl Pts',(-5.793639449625,-2.903780178711,-0.6832356592843));
#42411=CARTESIAN_POINT('Ctrl Pts',(-5.712389449625,-1.512462712197,-3.245723662317));
#42412=CARTESIAN_POINT('Ctrl Pts',(-5.631139449625,1.181419990037,-4.361566413001));
#42413=CARTESIAN_POINT('Ctrl Pts',(-5.549889449625,3.977182649303,-3.533423784903));
#42414=CARTESIAN_POINT('Ctrl Pts',(-5.468639449625,5.628731265186,-1.130405635211));
#42415=CARTESIAN_POINT('Ctrl Pts',(-5.387389449625,5.39995728572,1.776443433137));
#42416=CARTESIAN_POINT('Ctrl Pts',(-5.306139449625,3.392827099615,3.89151732732));
#42417=CARTESIAN_POINT('Ctrl Pts',(-5.224889449625,0.501934923806,4.272110470055));
#42418=CARTESIAN_POINT('Ctrl Pts',(-5.143639449625,-1.984225552094,2.748589643777));
#42419=CARTESIAN_POINT('Ctrl Pts',(-5.062389449625,-2.957551391752,-4.355651576082E-7));
#42420=CARTESIAN_POINT('Ctrl Pts',(-4.981139449625,-1.984227628837,-2.748587901516));
#42421=CARTESIAN_POINT('Ctrl Pts',(-4.899889449625,0.5019432307773,-4.272116567967));
#42422=CARTESIAN_POINT('Ctrl Pts',(-4.818639449625,3.392795948473,-3.891494677932));
#42423=CARTESIAN_POINT('Ctrl Pts',(-4.737389449625,5.400073583318,-1.776527932779));
#42424=CARTESIAN_POINT('Ctrl Pts',(-4.656139449625,5.628297225935,1.130720984389));
#42425=CARTESIAN_POINT('Ctrl Pts',(-4.601972782958,4.528634081117,2.731738253352));
#42426=CARTESIAN_POINT('Ctrl Pts',(-4.574889449625,3.786480308739,3.270944531304));
#42427=CARTESIAN_POINT('Ctrl Pts',(-7.081316447316,-0.1685597971619,-3.545503354232));
#42428=CARTESIAN_POINT('Ctrl Pts',(-7.054233113983,0.6358893960722,-3.903667210934));
#42429=CARTESIAN_POINT('Ctrl Pts',(-7.000066447316,2.494621416475,-4.049408593792));
#42430=CARTESIAN_POINT('Ctrl Pts',(-6.918816447316,4.801908064657,-2.464329996843));
#42431=CARTESIAN_POINT('Ctrl Pts',(-6.837566447316,5.596693702003,0.2194321288388));
#42432=CARTESIAN_POINT('Ctrl Pts',(-6.756316447316,4.525623755341,2.805308050628));
#42433=CARTESIAN_POINT('Ctrl Pts',(-6.675066447316,2.065844864405,4.140857897789));
#42434=CARTESIAN_POINT('Ctrl Pts',(-6.593816447316,-0.686235909742,3.630787936533));
#42435=CARTESIAN_POINT('Ctrl Pts',(-6.512566447316,-2.504011016761,1.502448072752));
#42436=CARTESIAN_POINT('Ctrl Pts',(-6.431316447316,-2.57727883269,-1.295545463045));
#42437=CARTESIAN_POINT('Ctrl Pts',(-6.350066447316,-0.8733845264335,-3.516103806355));
#42438=CARTESIAN_POINT('Ctrl Pts',(-6.268816447316,1.848232775784,-4.169506314214));
#42439=CARTESIAN_POINT('Ctrl Pts',(-6.187566447316,4.374526171585,-2.964526172083));
#42440=CARTESIAN_POINT('Ctrl Pts',(-6.106316447316,5.579506312963,-0.4382327725412));
#42441=CARTESIAN_POINT('Ctrl Pts',(-6.025066447316,4.926103811857,2.283384513961));
#42442=CARTESIAN_POINT('Ctrl Pts',(-5.943816447316,2.70554544229,3.987278879338));
#42443=CARTESIAN_POINT('Ctrl Pts',(-5.862566447316,-0.09244799523316,3.914010842643));
#42444=CARTESIAN_POINT('Ctrl Pts',(-5.781316447316,-2.220788225852,2.096236559566));
#42445=CARTESIAN_POINT('Ctrl Pts',(-5.700066447316,-2.730856818033,-0.6558472895844));
#42446=CARTESIAN_POINT('Ctrl Pts',(-5.618816447316,-1.395312080335,-3.11561470445));
#42447=CARTESIAN_POINT('Ctrl Pts',(-5.537566447316,1.19058291023,-4.186727480392));
#42448=CARTESIAN_POINT('Ctrl Pts',(-5.456316447316,3.874273870273,-3.391782001995));
#42449=CARTESIAN_POINT('Ctrl Pts',(-5.375066447316,5.459618061001,-1.085091888735));
#42450=CARTESIAN_POINT('Ctrl Pts',(-5.293816447316,5.240014777241,1.705232440507));
#42451=CARTESIAN_POINT('Ctrl Pts',(-5.212566447316,3.31334295543,3.735520909677));
#42452=CARTESIAN_POINT('Ctrl Pts',(-5.131316447316,0.5383358664096,4.100857492604));
#42453=CARTESIAN_POINT('Ctrl Pts',(-5.050066447316,-1.84816370725,2.638408934831));
#42454=CARTESIAN_POINT('Ctrl Pts',(-4.968816447316,-2.782472543663,-4.181049745989E-7));
#42455=CARTESIAN_POINT('Ctrl Pts',(-4.887566447316,-1.848165700744,-2.638407262411));
#42456=CARTESIAN_POINT('Ctrl Pts',(-4.806316447316,0.5383438403855,-4.100863346074));
#42457=CARTESIAN_POINT('Ctrl Pts',(-4.725066447316,3.313313053021,-3.735499168218));
#42458=CARTESIAN_POINT('Ctrl Pts',(-4.643816447316,5.240126412902,-1.705313552873));
#42459=CARTESIAN_POINT('Ctrl Pts',(-4.562566447316,5.459201420765,1.08539459674));
#42460=CARTESIAN_POINT('Ctrl Pts',(-4.50839978065,4.403619670625,2.622233053807));
#42461=CARTESIAN_POINT('Ctrl Pts',(-4.481316447316,3.691216075387,3.139824562851));
#42462=CARTESIAN_POINT('Ctrl Pts',(-6.987743445008,-0.1026386902142,-3.397442123851));
#42463=CARTESIAN_POINT('Ctrl Pts',(-6.960660111674,0.6682164754788,-3.740648955836));
#42464=CARTESIAN_POINT('Ctrl Pts',(-6.906493445008,2.449327317055,-3.880304137017));
#42465=CARTESIAN_POINT('Ctrl Pts',(-6.825243445008,4.660261017337,-2.361418873952));
#42466=CARTESIAN_POINT('Ctrl Pts',(-6.743993445008,5.421856179989,0.2102685806102));
#42467=CARTESIAN_POINT('Ctrl Pts',(-6.662743445008,4.395514419506,2.688157587048));
#42468=CARTESIAN_POINT('Ctrl Pts',(-6.581493445008,2.038456595982,3.96793449202));
#42469=CARTESIAN_POINT('Ctrl Pts',(-6.500243445008,-0.5986965008186,3.479165197693));
#42470=CARTESIAN_POINT('Ctrl Pts',(-6.418993445008,-2.340560801384,1.439705413104));
#42471=CARTESIAN_POINT('Ctrl Pts',(-6.337743445008,-2.410768932443,-1.241443115336));
#42472=CARTESIAN_POINT('Ctrl Pts',(-6.256493445008,-0.7780297379481,-3.369270309471));
#42473=CARTESIAN_POINT('Ctrl Pts',(-6.175243445008,1.829932050191,-3.995386542412));
#42474=CARTESIAN_POINT('Ctrl Pts',(-6.093993445008,4.250726713904,-2.840726714381));
#42475=CARTESIAN_POINT('Ctrl Pts',(-6.012743445008,5.405386541213,-0.4199320470834));
#42476=CARTESIAN_POINT('Ctrl Pts',(-5.931493445008,4.779270314743,2.188029725996));
#42477=CARTESIAN_POINT('Ctrl Pts',(-5.850243445008,2.651443095448,3.820768977142));
#42478=CARTESIAN_POINT('Ctrl Pts',(-5.768993445008,-0.02970533882237,3.750560634537));
#42479=CARTESIAN_POINT('Ctrl Pts',(-5.687743445008,-2.06916547493,2.008697123506));
#42480=CARTESIAN_POINT('Ctrl Pts',(-5.606493445008,-2.557933457354,-0.6284589198844));
#42481=CARTESIAN_POINT('Ctrl Pts',(-5.525243445008,-1.278161448473,-2.985505746582));
#42482=CARTESIAN_POINT('Ctrl Pts',(-5.443993445008,1.199745830423,-4.011888547782));
#42483=CARTESIAN_POINT('Ctrl Pts',(-5.362743445008,3.771365091244,-3.250140219087));
#42484=CARTESIAN_POINT('Ctrl Pts',(-5.281493445008,5.290504856815,-1.039778142259));
#42485=CARTESIAN_POINT('Ctrl Pts',(-5.200243445008,5.080072268762,1.634021447877));
#42486=CARTESIAN_POINT('Ctrl Pts',(-5.118993445008,3.233858811244,3.579524492034));
#42487=CARTESIAN_POINT('Ctrl Pts',(-5.037743445008,0.5747368090133,3.929604515154));
#42488=CARTESIAN_POINT('Ctrl Pts',(-4.956493445008,-1.712101862406,2.528228225885));
#42489=CARTESIAN_POINT('Ctrl Pts',(-4.875243445008,-2.607393695574,-4.00644791597E-7));
#42490=CARTESIAN_POINT('Ctrl Pts',(-4.793993445008,-1.712103772651,-2.528226623306));
#42491=CARTESIAN_POINT('Ctrl Pts',(-4.712743445008,0.5747444499936,-3.929610124181));
#42492=CARTESIAN_POINT('Ctrl Pts',(-4.631493445008,3.233830157568,-3.579503658505));
#42493=CARTESIAN_POINT('Ctrl Pts',(-4.550243445008,5.080179242486,-1.634099172968));
#42494=CARTESIAN_POINT('Ctrl Pts',(-4.468993445008,5.290105615594,1.040068209092));
#42495=CARTESIAN_POINT('Ctrl Pts',(-4.414826778341,4.278605260133,2.512727854262));
#42496=CARTESIAN_POINT('Ctrl Pts',(-4.387743445008,3.595951842036,3.008704594398));
#42497=CARTESIAN_POINT('Ctrl Pts',(-6.894170442699,-0.03671758326641,-3.24938089347));
#42498=CARTESIAN_POINT('Ctrl Pts',(-6.867087109366,0.7005435548854,-3.577630700739));
#42499=CARTESIAN_POINT('Ctrl Pts',(-6.812920442699,2.404033217635,-3.711199680242));
#42500=CARTESIAN_POINT('Ctrl Pts',(-6.731670442699,4.518613970016,-2.258507751061));
#42501=CARTESIAN_POINT('Ctrl Pts',(-6.650420442699,5.247018657974,0.2011050323816));
#42502=CARTESIAN_POINT('Ctrl Pts',(-6.569170442699,4.265405083671,2.571007123468));
#42503=CARTESIAN_POINT('Ctrl Pts',(-6.487920442699,2.011068327558,3.795011086251));
#42504=CARTESIAN_POINT('Ctrl Pts',(-6.406670442699,-0.5111570918951,3.327542458853));
#42505=CARTESIAN_POINT('Ctrl Pts',(-6.325420442699,-2.177110586008,1.376962753456));
#42506=CARTESIAN_POINT('Ctrl Pts',(-6.244170442699,-2.244259032195,-1.187340767628));
#42507=CARTESIAN_POINT('Ctrl Pts',(-6.162920442699,-0.6826749494628,-3.222436812587));
#42508=CARTESIAN_POINT('Ctrl Pts',(-6.081670442699,1.811631324597,-3.821266770609));
#42509=CARTESIAN_POINT('Ctrl Pts',(-6.000420442699,4.126927256222,-2.716927256679));
#42510=CARTESIAN_POINT('Ctrl Pts',(-5.919170442699,5.231266769463,-0.4016313216255));
#42511=CARTESIAN_POINT('Ctrl Pts',(-5.837920442699,4.632436817629,2.092674938032));
#42512=CARTESIAN_POINT('Ctrl Pts',(-5.756670442699,2.597340748606,3.654259074947));
#42513=CARTESIAN_POINT('Ctrl Pts',(-5.675420442699,0.03303731758842,3.587110426432));
#42514=CARTESIAN_POINT('Ctrl Pts',(-5.594170442699,-1.917542724007,1.921157687446));
#42515=CARTESIAN_POINT('Ctrl Pts',(-5.512920442699,-2.385010096676,-0.6010705501845));
#42516=CARTESIAN_POINT('Ctrl Pts',(-5.431670442699,-1.161010816611,-2.855396788715));
#42517=CARTESIAN_POINT('Ctrl Pts',(-5.350420442699,1.208908750616,-3.837049615173));
#42518=CARTESIAN_POINT('Ctrl Pts',(-5.269170442699,3.668456312214,-3.108498436179));
#42519=CARTESIAN_POINT('Ctrl Pts',(-5.187920442699,5.121391652629,-0.9944643957835));
#42520=CARTESIAN_POINT('Ctrl Pts',(-5.106670442699,4.920129760283,1.562810455248));
#42521=CARTESIAN_POINT('Ctrl Pts',(-5.025420442699,3.154374667059,3.423528074391));
#42522=CARTESIAN_POINT('Ctrl Pts',(-4.944170442699,0.6111377516169,3.758351537704));
#42523=CARTESIAN_POINT('Ctrl Pts',(-4.862920442699,-1.576040017561,2.418047516939));
#42524=CARTESIAN_POINT('Ctrl Pts',(-4.781670442699,-2.432314847485,-3.831846085989E-7));
#42525=CARTESIAN_POINT('Ctrl Pts',(-4.700420442699,-1.576041844558,-2.418045984201));
#42526=CARTESIAN_POINT('Ctrl Pts',(-4.619170442699,0.6111450596018,-3.758356902288));
#42527=CARTESIAN_POINT('Ctrl Pts',(-4.537920442699,3.154347262116,-3.423508148791));
#42528=CARTESIAN_POINT('Ctrl Pts',(-4.456670442699,4.92023207207,-1.562884793063));
#42529=CARTESIAN_POINT('Ctrl Pts',(-4.375420442699,5.121009810423,0.9947418214435));
#42530=CARTESIAN_POINT('Ctrl Pts',(-4.321253776032,4.153590849641,2.403222654717));
#42531=CARTESIAN_POINT('Ctrl Pts',(-4.294170442699,3.500687608684,2.877584625945));
#42532=CARTESIAN_POINT('',(-4.36903811233822,4.52608525564794,1.79907266111361));
#42533=CARTESIAN_POINT('Ctrl Pts',(-6.86908159826512,1.41000225333245,-3.59814532547397));
#42534=CARTESIAN_POINT('Ctrl Pts',(-6.85656564768471,1.78745793235516,-3.59874068850376));
#42535=CARTESIAN_POINT('Ctrl Pts',(-6.84201839498573,2.23012755211558,-3.54264151700861));
#42536=CARTESIAN_POINT('Ctrl Pts',(-6.80955126796814,3.14211258271628,-3.1885791377597));
#42537=CARTESIAN_POINT('Ctrl Pts',(-6.79393475271691,3.5477764910093,-2.93114612264598));
#42538=CARTESIAN_POINT('Ctrl Pts',(-6.7624895482582,4.23674269123054,-2.27963350176036));
#42539=CARTESIAN_POINT('Ctrl Pts',(-6.74704728409703,4.50915827316548,-1.89158780048281));
#42540=CARTESIAN_POINT('Ctrl Pts',(-6.71599955276356,4.88602617929508,-1.03437663024274));
#42541=CARTESIAN_POINT('Ctrl Pts',(-6.70071788562139,4.99173694839489,-0.576725573750675));
#42542=CARTESIAN_POINT('Ctrl Pts',(-6.66706020219651,5.02689620983516,0.436826228201624));
#42543=CARTESIAN_POINT('Ctrl Pts',(-6.65140080005729,4.91393240444917,0.90568359141837));
#42544=CARTESIAN_POINT('Ctrl Pts',(-6.62359464961269,4.61718657022314,1.69044375960114));
#42545=CARTESIAN_POINT('Ctrl Pts',(-6.60868269931122,4.38093761369227,2.08235534769542));
#42546=CARTESIAN_POINT('Ctrl Pts',(-6.57793444640711,3.75934740684366,2.76895553999336));
#42547=CARTESIAN_POINT('Ctrl Pts',(-6.56213235429517,3.36694690053603,3.05577123496503));
#42548=CARTESIAN_POINT('Ctrl Pts',(-6.53340558182412,2.58249721445423,3.4243114842652));
#42549=CARTESIAN_POINT('Ctrl Pts',(-6.51810701650023,2.13443855169954,3.56796020431119));
#42550=CARTESIAN_POINT('Ctrl Pts',(-6.48463857946336,1.12707558514785,3.61776937546146));
#42551=CARTESIAN_POINT('Ctrl Pts',(-6.46902258645918,0.651773498827994,
3.54790362030401));
#42552=CARTESIAN_POINT('Ctrl Pts',(-6.43757513255404,-0.24284227260902,
3.23348418370255));
#42553=CARTESIAN_POINT('Ctrl Pts',(-6.42212964462873,-0.649778439883527,
2.99000998636925));
#42554=CARTESIAN_POINT('Ctrl Pts',(-6.39107630633123,-1.3432464375128,2.3605247329833));
#42555=CARTESIAN_POINT('Ctrl Pts',(-6.37579303405225,-1.62623604957389,
1.98558191396071));
#42556=CARTESIAN_POINT('Ctrl Pts',(-6.34214219201528,-2.07110679903882,
1.07444004263209));
#42557=CARTESIAN_POINT('Ctrl Pts',(-6.32648728537324,-2.15897813573259,
0.600392684303986));
#42558=CARTESIAN_POINT('Ctrl Pts',(-6.29867522834268,-2.20763567912064,
-0.237365748009939));
#42559=CARTESIAN_POINT('Ctrl Pts',(-6.28376661051732,-2.15151016120919,
-0.691423320158909));
#42560=CARTESIAN_POINT('Ctrl Pts',(-6.25302374795656,-1.86366136469891,
-1.57156326080986));
#42561=CARTESIAN_POINT('Ctrl Pts',(-6.23722090140809,-1.62213891078368,
-1.99337880265141));
#42562=CARTESIAN_POINT('Ctrl Pts',(-6.20850151358295,-1.05602558623953,
-2.64936192882867));
#42563=CARTESIAN_POINT('Ctrl Pts',(-6.19320377233992,-0.705426956801188,
-2.96312899578155));
#42564=CARTESIAN_POINT('Ctrl Pts',(-6.15973338876674,0.194258412510738,
-3.41912431062218));
#42565=CARTESIAN_POINT('Ctrl Pts',(-6.14411533253787,0.656850288984262,
-3.54898770846589));
#42566=CARTESIAN_POINT('Ctrl Pts',(-6.11266882970534,1.60192740622801,-3.62633630936245));
#42567=CARTESIAN_POINT('Ctrl Pts',(-6.09722630917239,2.07266918334271,-3.56984723484898));
#42568=CARTESIAN_POINT('Ctrl Pts',(-6.06616958007161,2.96254424139103,-3.27752189348108));
#42569=CARTESIAN_POINT('Ctrl Pts',(-6.05088334171184,3.37382340294493,-3.05035443589433));
#42570=CARTESIAN_POINT('Ctrl Pts',(-6.01723599099568,4.1512345641346,-2.39957165922417));
#42571=CARTESIAN_POINT('Ctrl Pts',(-6.00158448221301,4.42461826958585,-2.0025917916969));
#42572=CARTESIAN_POINT('Ctrl Pts',(-5.9737667122899,4.81044759733959,-1.25718605363803));
#42573=CARTESIAN_POINT('Ctrl Pts',(-5.95886224958743,4.94413068178708,-0.819773855555199));
#42574=CARTESIAN_POINT('Ctrl Pts',(-5.92812579438059,5.0399590726211,0.101074923696212));
#42575=CARTESIAN_POINT('Ctrl Pts',(-5.91232206896784,4.99128197185478,0.584723013701021));
#42576=CARTESIAN_POINT('Ctrl Pts',(-5.8836106328302,4.74167646430498,1.41423121271077));
#42577=CARTESIAN_POINT('Ctrl Pts',(-5.86831397111165,4.54945191106594,1.84363856859817));
#42578=CARTESIAN_POINT('Ctrl Pts',(-5.83484192873968,3.91372603349253,2.62677649317481));
#42579=CARTESIAN_POINT('Ctrl Pts',(-5.81922153650868,3.54415596621539,2.93393145271936));
#42580=CARTESIAN_POINT('Ctrl Pts',(-5.78777613424304,2.7126629955164,3.38969639168488));
#42581=CARTESIAN_POINT('Ctrl Pts',(-5.77233698452416,2.25988270259248,3.52997791484526));
#42582=CARTESIAN_POINT('Ctrl Pts',(-5.74127638223186,1.32801856216453,3.62573247975942));
#42583=CARTESIAN_POINT('Ctrl Pts',(-5.72598675889398,0.859755722308294,
3.58587428719093));
#42584=CARTESIAN_POINT('Ctrl Pts',(-5.69234301257561,-0.115279376707324,
3.30841367623825));
#42585=CARTESIAN_POINT('Ctrl Pts',(-5.67669533552535,-0.526643436121224,
3.05744210709078));
#42586=CARTESIAN_POINT('Ctrl Pts',(-5.64887143387965,-1.18288818883317,
2.53385355868996));
#42587=CARTESIAN_POINT('Ctrl Pts',(-5.63397175644942,-1.48310920504433,
2.18898786501864));
#42588=CARTESIAN_POINT('Ctrl Pts',(-5.60414802819858,-1.932273702204,1.41101213498186));
#42589=CARTESIAN_POINT('Ctrl Pts',(-5.58924835076831,-2.08082564571144,
0.978580261357411));
#42590=CARTESIAN_POINT('Ctrl Pts',(-5.56142444912252,-2.20614425340107,
0.148461360208148));
#42591=CARTESIAN_POINT('Ctrl Pts',(-5.5457767720722,-2.21780997820335,-0.333276150021961));
#42592=CARTESIAN_POINT('Ctrl Pts',(-5.51213302575366,-1.97058036632984,
-1.31641162082767));
#42593=CARTESIAN_POINT('Ctrl Pts',(-5.49684340241566,-1.77096715371477,
-1.7418682320759));
#42594=CARTESIAN_POINT('Ctrl Pts',(-5.46578280012323,-1.22210919775633,
-2.50100896810563));
#42595=CARTESIAN_POINT('Ctrl Pts',(-5.45034365040435,-0.874231688555608,
-2.82298744253071));
#42596=CARTESIAN_POINT('Ctrl Pts',(-5.41889824813859,-0.0637811879073202,
-3.31519900874149));
#42597=CARTESIAN_POINT('Ctrl Pts',(-5.4032778559075,0.387007843595256,-3.48167859570946));
#42598=CARTESIAN_POINT('Ctrl Pts',(-5.36980581353536,1.38308811973198,-3.64066439324238));
#42599=CARTESIAN_POINT('Ctrl Pts',(-5.3545091518167,1.85107807512154,-3.59243206163464));
#42600=CARTESIAN_POINT('Ctrl Pts',(-5.3257977156791,2.69425600188595,-3.39384267259226));
#42601=CARTESIAN_POINT('Ctrl Pts',(-5.30999399026649,3.13744608470506,-3.19417423343593));
#42602=CARTESIAN_POINT('Ctrl Pts',(-5.27925753505974,3.88701032516358,-2.65076002294397));
#42603=CARTESIAN_POINT('Ctrl Pts',(-5.26435307235728,4.19897885840477,-2.31628097671465));
#42604=CARTESIAN_POINT('Ctrl Pts',(-5.23653530243416,4.65160449981346,-1.60944010832521));
#42605=CARTESIAN_POINT('Ctrl Pts',(-5.22088379365139,4.85870729715726,-1.17419294066014));
#42606=CARTESIAN_POINT('Ctrl Pts',(-5.18723644293534,5.0335961335039,-0.175543737549326));
#42607=CARTESIAN_POINT('Ctrl Pts',(-5.17195020457575,5.02468934191009,0.29421819319692));
#42608=CARTESIAN_POINT('Ctrl Pts',(-5.14089347547514,4.83291298468031,1.21103527034499));
#42609=CARTESIAN_POINT('Ctrl Pts',(-5.12545095494229,4.64646306968778,1.64695414520581));
#42610=CARTESIAN_POINT('Ctrl Pts',(-5.09400445210965,4.10693865774205,2.42674063682608));
#42611=CARTESIAN_POINT('Ctrl Pts',(-5.07838639588057,3.76317771795078,2.76242525451461));
#42612=CARTESIAN_POINT('Ctrl Pts',(-5.04491601230736,2.91843150663598,3.31357798233151));
#42613=CARTESIAN_POINT('Ctrl Pts',(-5.02961827106443,2.47140194106463,3.46032176848062));
#42614=CARTESIAN_POINT('Ctrl Pts',(-5.0008988832394,1.62024722706905,3.62259872586796));
#42615=CARTESIAN_POINT('Ctrl Pts',(-4.98509603669101,1.13418302516555,3.62085553562207));
#42616=CARTESIAN_POINT('Ctrl Pts',(-4.95435317413029,0.228035079421312,
3.43006993552313));
#42617=CARTESIAN_POINT('Ctrl Pts',(-4.93944455630491,-0.193253071796147,
3.25164727376046));
#42618=CARTESIAN_POINT('Ctrl Pts',(-4.91163249927437,-0.894444384720605,
2.79062938894352));
#42619=CARTESIAN_POINT('Ctrl Pts',(-4.89597759263239,-1.26104577128262,
2.47750689993816));
#42620=CARTESIAN_POINT('Ctrl Pts',(-4.86232675059547,-1.8276824035723,1.63666659383646));
#42621=CARTESIAN_POINT('Ctrl Pts',(-4.84704347831652,-2.01089760378185,
1.20411899127301));
#42622=CARTESIAN_POINT('Ctrl Pts',(-4.81599014001893,-2.20931382570703,
0.288815461921366));
#42623=CARTESIAN_POINT('Ctrl Pts',(-4.80054465209355,-2.21670058212636,
-0.185338695323713));
#42624=CARTESIAN_POINT('Ctrl Pts',(-4.76909719818808,-2.0416879159481,-1.11730839831502));
#42625=CARTESIAN_POINT('Ctrl Pts',(-4.75348120518357,-1.86454239160905,
-1.56386495711833));
#42626=CARTESIAN_POINT('Ctrl Pts',(-4.72001276814644,-1.31772490077557,
-2.41136229140834));
#42627=CARTESIAN_POINT('Ctrl Pts',(-4.70471420282251,-0.969292128617286,
-2.72756811571648));
#42628=CARTESIAN_POINT('Ctrl Pts',(-4.67598743035164,-0.25790206736538,
-3.22265134720376));
#42629=CARTESIAN_POINT('Ctrl Pts',(-4.66018533824,0.186687863837955,-3.41907230663808));
#42630=CARTESIAN_POINT('Ctrl Pts',(-4.6294370853362,1.09209617603565,-3.61408512036354));
#42631=CARTESIAN_POINT('Ctrl Pts',(-4.61452513503486,1.54962604562839,-3.62272692428965));
#42632=CARTESIAN_POINT('Ctrl Pts',(-4.58671898459036,2.37762120426606,-3.48733627110506));
#42633=CARTESIAN_POINT('Ctrl Pts',(-4.57105958245111,2.84014549425619,-3.35073711466903));
#42634=CARTESIAN_POINT('Ctrl Pts',(-4.53740189902619,3.70032747207835,-2.81351240010708));
#42635=CARTESIAN_POINT('Ctrl Pts',(-4.52212023188399,4.04380952851943,-2.49313866036687));
#42636=CARTESIAN_POINT('Ctrl Pts',(-4.49107250055042,4.59774222529018,-1.73815589466743));
#42637=CARTESIAN_POINT('Ctrl Pts',(-4.47563023638915,4.79759186945824,-1.30821422968639));
#42638=CARTESIAN_POINT('Ctrl Pts',(-4.44418503193031,5.01733524992042,-0.38579568750342));
#42639=CARTESIAN_POINT('Ctrl Pts',(-4.42856851667902,5.03744682663507,0.0942360700334575));
#42640=CARTESIAN_POINT('Ctrl Pts',(-4.39610133443088,4.88808107219921,1.06107110873269));
#42641=CARTESIAN_POINT('Ctrl Pts',(-4.38155405604991,4.71532880232278,1.47248441266071));
#42642=CARTESIAN_POINT('Ctrl Pts',(-4.3690381116678,4.52608525532423,1.79907266090034));
#42643=CARTESIAN_POINT('Ctrl Pts',(-4.60069824814697,4.87339643710536,1.99959286527304));
#42644=CARTESIAN_POINT('Ctrl Pts',(-4.56225271749423,4.81575785116069,1.96631521216219));
#42645=CARTESIAN_POINT('Ctrl Pts',(-4.52380718684145,4.75811926521517,1.93303755905287));
#42646=CARTESIAN_POINT('Ctrl Pts',(-4.44658714145964,4.64234887144461,1.86619749104525));
#42647=CARTESIAN_POINT('Ctrl Pts',(-4.40781262673061,4.58421706361958,1.83263507614692));
#42648=CARTESIAN_POINT('Ctrl Pts',(-4.36903811200149,4.5260852557937,1.79907266125016));
#42649=CARTESIAN_POINT('Ctrl Pts',(-4.60038478407041,4.87292780285437,1.99931896219052));
#42650=CARTESIAN_POINT('Ctrl Pts',(-4.6035703024737,4.92593446793067,1.90795956928389));
#42651=CARTESIAN_POINT('Ctrl Pts',(-4.60672386917096,4.97533475390575,1.81450692734378));
#42652=CARTESIAN_POINT('Ctrl Pts',(-4.61408610987978,5.08335468073265,1.58866596006262));
#42653=CARTESIAN_POINT('Ctrl Pts',(-4.61820792381689,5.13828760357301,1.45536284527102));
#42654=CARTESIAN_POINT('Ctrl Pts',(-4.62751113351263,5.24542152639251,1.14850112082971));
#42655=CARTESIAN_POINT('Ctrl Pts',(-4.63270616058839,5.29296121703815,0.974576465761229));
#42656=CARTESIAN_POINT('Ctrl Pts',(-4.6488842581937,5.40000279831522,0.442314977411726));
#42657=CARTESIAN_POINT('Ctrl Pts',(-4.66017405850537,5.4230197842342,0.0773920769223206));
#42658=CARTESIAN_POINT('Ctrl Pts',(-4.67632980023208,5.38624878581296,-0.448695553793838));
#42659=CARTESIAN_POINT('Ctrl Pts',(-4.68135338643631,5.36466139121163,-0.612897342153464));
#42660=CARTESIAN_POINT('Ctrl Pts',(-4.69224737003279,5.29454390370242,-0.972005719990289));
#42661=CARTESIAN_POINT('Ctrl Pts',(-4.69797243738255,5.24147084555266,-1.16480913145431));
#42662=CARTESIAN_POINT('Ctrl Pts',(-4.70781276117758,5.12471824454401,-1.4894595964008));
#42663=CARTESIAN_POINT('Ctrl Pts',(-4.71194275738303,5.06844846719185,-1.62241111450313));
#42664=CARTESIAN_POINT('Ctrl Pts',(-4.72745569362673,4.83664530764845,-2.09553888496919));
#42665=CARTESIAN_POINT('Ctrl Pts',(-4.73934447005763,4.61886330285552,-2.4143241259663));
#42666=CARTESIAN_POINT('Ctrl Pts',(-4.7563410268637,4.24570641361292,-2.82363794847257));
#42667=CARTESIAN_POINT('Ctrl Pts',(-4.76158384758496,4.12177941933755,-2.94337786218929));
#42668=CARTESIAN_POINT('Ctrl Pts',(-4.77264780630134,3.83937965718473,-3.18302488007073));
#42669=CARTESIAN_POINT('Ctrl Pts',(-4.77834885694988,3.67928048231338,-3.29947962163654));
#42670=CARTESIAN_POINT('Ctrl Pts',(-4.78809945679421,3.38876454575258,-3.47877623962825));
#42671=CARTESIAN_POINT('Ctrl Pts',(-4.79217579565211,3.26332005198182,-3.54705929676832));
#42672=CARTESIAN_POINT('Ctrl Pts',(-4.80867299637761,2.75596636334532,-3.78825845997545));
#42673=CARTESIAN_POINT('Ctrl Pts',(-4.82175168624108,2.34935327217074,-3.90791317220951));
#42674=CARTESIAN_POINT('Ctrl Pts',(-4.83955889519952,1.7728527316371,-3.98502389205297));
#42675=CARTESIAN_POINT('Ctrl Pts',(-4.84451582113769,1.60973684337904,-3.99690828055661));
#42676=CARTESIAN_POINT('Ctrl Pts',(-4.85484353222898,1.26258219512494,-4.00083450847173));
#42677=CARTESIAN_POINT('Ctrl Pts',(-4.8601103831318,1.07950933164658,-3.99015666742414));
#42678=CARTESIAN_POINT('Ctrl Pts',(-4.8694309966141,0.755751468539741,-3.94831972406825));
#42679=CARTESIAN_POINT('Ctrl Pts',(-4.87349818263631,0.615624898732014,
-3.92240616106197));
#42680=CARTESIAN_POINT('Ctrl Pts',(-4.88997937013341,0.0701586442008021,
-3.79040136171959));
#42681=CARTESIAN_POINT('Ctrl Pts',(-4.90305151960809,-0.320841553370625,
-3.6274226805427));
#42682=CARTESIAN_POINT('Ctrl Pts',(-4.92084575374689,-0.816921118602842,
-3.32458772652715));
#42683=CARTESIAN_POINT('Ctrl Pts',(-4.92579691850775,-0.950982573522889,
-3.23123973971505));
#42684=CARTESIAN_POINT('Ctrl Pts',(-4.93610604655926,-1.22270830914031,
-3.01614227416233));
#42685=CARTESIAN_POINT('Ctrl Pts',(-4.94136080897506,-1.35793532184405,
-2.89291433481441));
#42686=CARTESIAN_POINT('Ctrl Pts',(-4.95067147605834,-1.58298771247924,
-2.65693772910767));
#42687=CARTESIAN_POINT('Ctrl Pts',(-4.9547406724232,-1.6756334049896,-2.54856669999476));
#42688=CARTESIAN_POINT('Ctrl Pts',(-4.97122336166442,-2.01652107619069,
-2.10267894897076));
#42689=CARTESIAN_POINT('Ctrl Pts',(-4.98429462215974,-2.21783034751745,
-1.72998304527702));
#42690=CARTESIAN_POINT('Ctrl Pts',(-5.00208975083267,-2.41281820332782,
-1.18242790784559));
#42691=CARTESIAN_POINT('Ctrl Pts',(-5.00704233971896,-2.45827713873544,
-1.02547320963265));
#42692=CARTESIAN_POINT('Ctrl Pts',(-5.01735347034643,-2.53410514603836,
-0.687247815140309));
#42693=CARTESIAN_POINT('Ctrl Pts',(-5.02260884847203,-2.56165265704727,
-0.506362404759346));
#42694=CARTESIAN_POINT('Ctrl Pts',(-5.03191996922711,-2.58805099729946,
-0.181331217235873));
#42695=CARTESIAN_POINT('Ctrl Pts',(-5.03598902394775,-2.59185186661705,
-0.0388130227363775));
#42696=CARTESIAN_POINT('Ctrl Pts',(-5.05247169419802,-2.57617378243136,
0.522232472389581));
#42697=CARTESIAN_POINT('Ctrl Pts',(-5.06554311807892,-2.49808026283208,
0.938564511662007));
#42698=CARTESIAN_POINT('Ctrl Pts',(-5.08333835677935,-2.3050325751149,1.48681008555445));
#42699=CARTESIAN_POINT('Ctrl Pts',(-5.08829093116806,-2.2415881606383,1.63739542350894));
#42700=CARTESIAN_POINT('Ctrl Pts',(-5.09860344882482,-2.08764891710839,
1.94800992102914));
#42701=CARTESIAN_POINT('Ctrl Pts',(-5.10386010760204,-1.99519812734779,
2.10596059914832));
#42702=CARTESIAN_POINT('Ctrl Pts',(-5.11317255998373,-1.81113127679454,
2.3752064708769));
#42703=CARTESIAN_POINT('Ctrl Pts',(-5.117241671025,-1.72439197945323,2.48835510650853));
#42704=CARTESIAN_POINT('Ctrl Pts',(-5.13372236742965,-1.35916593970459,
2.91444128970349));
#42705=CARTESIAN_POINT('Ctrl Pts',(-5.14679144608301,-1.03652730430544,
3.18879932984976));
#42706=CARTESIAN_POINT('Ctrl Pts',(-5.16458502497042,-0.541536684159376,
3.49336223301086));
#42707=CARTESIAN_POINT('Ctrl Pts',(-5.16953807765692,-0.39745380021034,
3.57047257538952));
#42708=CARTESIAN_POINT('Ctrl Pts',(-5.17985296404238,-0.0822776288367675,
3.715026423268));
#42709=CARTESIAN_POINT('Ctrl Pts',(-5.18511137697027,0.0890299587085872,
3.7796172228988));
#42710=CARTESIAN_POINT('Ctrl Pts',(-5.1944260539882,0.401595391251225,3.87303712917641));
#42711=CARTESIAN_POINT('Ctrl Pts',(-5.19849564684741,0.540226854777863,
3.90638218415407));
#42712=CARTESIAN_POINT('Ctrl Pts',(-5.21497062076652,1.09200879209013,4.00761093973977));
#42713=CARTESIAN_POINT('Ctrl Pts',(-5.22803248743137,1.51517703941989,4.01779722385531));
#42714=CARTESIAN_POINT('Ctrl Pts',(-5.24582133764916,2.09137133000897,3.94307223682389));
#42715=CARTESIAN_POINT('Ctrl Pts',(-5.25077620067333,2.25192966344508,3.91233032534663));
#42716=CARTESIAN_POINT('Ctrl Pts',(-5.26110079628887,2.58815230117755,3.82627314298496));
#42717=CARTESIAN_POINT('Ctrl Pts',(-5.26636653046677,2.76217799178062,3.76857817963031));
#42718=CARTESIAN_POINT('Ctrl Pts',(-5.2756900115597,3.06414979897996,3.64432388388499));
#42719=CARTESIAN_POINT('Ctrl Pts',(-5.27976113441245,3.19290558586765,3.58295724120763));
#42720=CARTESIAN_POINT('Ctrl Pts',(-5.29621568984227,3.68474781087186,3.31465467918565));
#42721=CARTESIAN_POINT('Ctrl Pts',(-5.30925207780753,4.01942115211145,3.05680262026333));
#42722=CARTESIAN_POINT('Ctrl Pts',(-5.3270240666099,4.41995990930571,2.63671459348876));
#42723=CARTESIAN_POINT('Ctrl Pts',(-5.33198519886083,4.52555986500751,2.51167232241837));
#42724=CARTESIAN_POINT('Ctrl Pts',(-5.34234341881043,4.73343265160419,2.23238333634713));
#42725=CARTESIAN_POINT('Ctrl Pts',(-5.3476344989158,4.83284681560513,2.07726484198014));
#42726=CARTESIAN_POINT('Ctrl Pts',(-5.35698863604942,4.98973040992224,1.78965928054136));
#42727=CARTESIAN_POINT('Ctrl Pts',(-5.36106522943616,5.05118636144953,1.66076044044048));
#42728=CARTESIAN_POINT('Ctrl Pts',(-5.37744732649883,5.2633223778622,1.14499878322517));
#42729=CARTESIAN_POINT('Ctrl Pts',(-5.39039335278322,5.36069205985606,0.73682290711044));
#42730=CARTESIAN_POINT('Ctrl Pts',(-5.40810573856788,5.40831514934431,0.160415114133084));
#42731=CARTESIAN_POINT('Ctrl Pts',(-5.41308938382183,5.41191584677786,-0.00390323901843598));
#42732=CARTESIAN_POINT('Ctrl Pts',(-5.42421436439621,5.3970440644381,-0.37740627340514));
#42733=CARTESIAN_POINT('Ctrl Pts',(-5.43017430376117,5.37219769669584,-0.584878068079895));
#42734=CARTESIAN_POINT('Ctrl Pts',(-5.44059768696027,5.30003297783807,-0.94248047016988));
#42735=CARTESIAN_POINT('Ctrl Pts',(-5.44506936436755,5.2603688794165,-1.09244637138767));
#42736=CARTESIAN_POINT('Ctrl Pts',(-5.4575443025882,5.12911243891207,-1.49191504831283));
#42737=CARTESIAN_POINT('Ctrl Pts',(-5.46568414727179,5.02122485529483,-1.73539122055828));
#42738=CARTESIAN_POINT('Ctrl Pts',(-5.48339908952568,4.73802558627545,-2.23658981625679));
#42739=CARTESIAN_POINT('Ctrl Pts',(-5.49297899782281,4.55410700945141,-2.48980476118052));
#42740=CARTESIAN_POINT('Ctrl Pts',(-5.50643445553346,4.24478756921484,-2.82495907783755));
#42741=CARTESIAN_POINT('Ctrl Pts',(-5.51058694952351,4.14085454108225,-2.9257765305949));
#42742=CARTESIAN_POINT('Ctrl Pts',(-5.52093657132699,3.86715748668139,-3.1633391894806));
#42743=CARTESIAN_POINT('Ctrl Pts',(-5.52715592007245,3.69210444161323,-3.29142779376694));
#42744=CARTESIAN_POINT('Ctrl Pts',(-5.53887399793356,3.35785980814675,-3.49621692938352));
#42745=CARTESIAN_POINT('Ctrl Pts',(-5.5441982500115,3.20308442348093,-3.57763549592054));
#42746=CARTESIAN_POINT('Ctrl Pts',(-5.56135647719954,2.69271752671186,-3.80555207068678));
#42747=CARTESIAN_POINT('Ctrl Pts',(-5.57331646009684,2.31910384288624,-3.91268855134794));
#42748=CARTESIAN_POINT('Ctrl Pts',(-5.58875002182019,1.79863387109188,-3.98302727131656));
#42749=CARTESIAN_POINT('Ctrl Pts',(-5.59275676580047,1.65887923890933,-3.99432367499748));
#42750=CARTESIAN_POINT('Ctrl Pts',(-5.60250657021499,1.31753324769005,-4.00359563815722));
#42751=CARTESIAN_POINT('Ctrl Pts',(-5.60827100141685,1.11713568192516,-3.99361579889223));
#42752=CARTESIAN_POINT('Ctrl Pts',(-5.61936844413469,0.748214458404577,
-3.94700732189921));
#42753=CARTESIAN_POINT('Ctrl Pts',(-5.62456782955319,0.580248495540013,
-3.91474781102115));
#42754=CARTESIAN_POINT('Ctrl Pts',(-5.64202869109998,0.0290543765692642,
-3.77245075419703));
#42755=CARTESIAN_POINT('Ctrl Pts',(-5.65445023878742,-0.342633980042864,
-3.61593464317991));
#42756=CARTESIAN_POINT('Ctrl Pts',(-5.67025629988414,-0.801958619087569,
-3.33505824895108));
#42757=CARTESIAN_POINT('Ctrl Pts',(-5.67423327412791,-0.916739185197197,
-3.25616569249984));
#42758=CARTESIAN_POINT('Ctrl Pts',(-5.68383956709192,-1.18349584160813,
-3.05113704587091));
#42759=CARTESIAN_POINT('Ctrl Pts',(-5.68948992730527,-1.32989561326599,
-2.91994828187451));
#42760=CARTESIAN_POINT('Ctrl Pts',(-5.70043449629585,-1.58417587641841,
-2.65547498388635));
#42761=CARTESIAN_POINT('Ctrl Pts',(-5.70560480027989,-1.69404300947267,
-2.52556125762722));
#42762=CARTESIAN_POINT('Ctrl Pts',(-5.7231383602013,-2.03522283953223,-2.06675560043406));
#42763=CARTESIAN_POINT('Ctrl Pts',(-5.73567052056328,-2.22748273832145,
-1.70825689135514));
#42764=CARTESIAN_POINT('Ctrl Pts',(-5.75156599480494,-2.40844954261256,
-1.19782329208381));
#42765=CARTESIAN_POINT('Ctrl Pts',(-5.75553633797694,-2.44787629006441,
-1.06445733848564));
#42766=CARTESIAN_POINT('Ctrl Pts',(-5.76510922149235,-2.52574739702303,
-0.738350992429132));
#42767=CARTESIAN_POINT('Ctrl Pts',(-5.77073271771454,-2.55679954926609,
-0.545209132280826));
#42768=CARTESIAN_POINT('Ctrl Pts',(-5.78164143197985,-2.58798656491482,
-0.180822322261445));
#42769=CARTESIAN_POINT('Ctrl Pts',(-5.78680500296509,-2.59167201613416,
-0.0109269046440773));
#42770=CARTESIAN_POINT('Ctrl Pts',(-5.8043555217336,-2.5683175062015,0.560935398308547));
#42771=CARTESIAN_POINT('Ctrl Pts',(-5.81691346823071,-2.49203377848039,
0.961348119108141));
#42772=CARTESIAN_POINT('Ctrl Pts',(-5.83282970047609,-2.31113156818679,
1.47258554747236));
#42773=CARTESIAN_POINT('Ctrl Pts',(-5.83679844779872,-2.25784635991363,
1.60099011966924));
#42774=CARTESIAN_POINT('Ctrl Pts',(-5.84636369073377,-2.11322477722094,
1.90317348646012));
#42775=CARTESIAN_POINT('Ctrl Pts',(-5.85198112237257,-2.01591397093011,
2.07262645731367));
#42776=CARTESIAN_POINT('Ctrl Pts',(-5.86288169834542,-1.81100355903198,
2.37523014621238));
#42777=CARTESIAN_POINT('Ctrl Pts',(-5.86804370107018,-1.70698989363315,
2.50955392441075));
#42778=CARTESIAN_POINT('Ctrl Pts',(-5.88559858416176,-1.32890077945757,
2.93942774296589));
#42779=CARTESIAN_POINT('Ctrl Pts',(-5.89816297819076,-1.01748136516023,
3.20274123435002));
#42780=CARTESIAN_POINT('Ctrl Pts',(-5.91408450248805,-0.554989599631195,
3.48627930074549));
#42781=CARTESIAN_POINT('Ctrl Pts',(-5.91805294469507,-0.43277713688448,
3.55252544851183));
#42782=CARTESIAN_POINT('Ctrl Pts',(-5.92761567211628,-0.130291101233887,
3.6963027695397));
#42783=CARTESIAN_POINT('Ctrl Pts',(-5.93323089022474,0.0518993214266012,
3.76672268133318));
#42784=CARTESIAN_POINT('Ctrl Pts',(-5.9441288630142,0.401494391228572,3.87291892401509));
#42785=CARTESIAN_POINT('Ctrl Pts',(-5.94929068481812,0.566854576580979,
3.91185314358545));
#42786=CARTESIAN_POINT('Ctrl Pts',(-5.96684585399282,1.13122133112492,4.0080058126726));
#42787=CARTESIAN_POINT('Ctrl Pts',(-5.97941074223079,1.53896471436482,4.0166650742138));
#42788=CARTESIAN_POINT('Ctrl Pts',(-5.99533278553194,2.07684470530957,3.94596574783833));
#42789=CARTESIAN_POINT('Ctrl Pts',(-5.99930129158615,2.21351485643232,3.92053930061174));
#42790=CARTESIAN_POINT('Ctrl Pts',(-6.00886367698267,2.53906472412968,3.84192106855853));
#42791=CARTESIAN_POINT('Ctrl Pts',(-6.0144784660986,2.72495947040826,3.78199858149246));
#42792=CARTESIAN_POINT('Ctrl Pts',(-6.02537458446193,3.06342520767069,3.64455124343639));
#42793=CARTESIAN_POINT('Ctrl Pts',(-6.03053491878416,3.21639598830336,3.57077129989299));
#42794=CARTESIAN_POINT('Ctrl Pts',(-6.04808979702491,3.71550980607629,3.29036196952939));
#42795=CARTESIAN_POINT('Ctrl Pts',(-6.06065621085059,4.03787773741545,3.04047995927916));
#42796=CARTESIAN_POINT('Ctrl Pts',(-6.076577503432,4.41139051034082,2.64706678040645));
#42797=CARTESIAN_POINT('Ctrl Pts',(-6.08054420752007,4.50156629507322,2.54135041529522));
#42798=CARTESIAN_POINT('Ctrl Pts',(-6.09011473601431,4.70529165940308,2.27515594889692));
#42799=CARTESIAN_POINT('Ctrl Pts',(-6.09573957130656,4.81223518646438,2.11129130400017));
#42800=CARTESIAN_POINT('Ctrl Pts',(-6.10665168319297,4.98896997997358,1.79096739541931));
#42801=CARTESIAN_POINT('Ctrl Pts',(-6.11181736549454,5.06145478402435,1.63718324939772));
#42802=CARTESIAN_POINT('Ctrl Pts',(-6.12938479342604,5.27285389105025,1.10470664553907));
#42803=CARTESIAN_POINT('Ctrl Pts',(-6.14195794858033,5.36602121342009,0.707359995913639));
#42804=CARTESIAN_POINT('Ctrl Pts',(-6.15789451213981,5.40848143073685,0.166017902455362));
#42805=CARTESIAN_POINT('Ctrl Pts',(-6.16186945335005,5.41195385370929,0.026823199581638));
#42806=CARTESIAN_POINT('Ctrl Pts',(-6.17139040514569,5.40256970591803,-0.306399653629353));
#42807=CARTESIAN_POINT('Ctrl Pts',(-6.17695711370529,5.382795545833,-0.498933285560094));
#42808=CARTESIAN_POINT('Ctrl Pts',(-6.18779443377622,5.31932381804776,-0.856657734443659));
#42809=CARTESIAN_POINT('Ctrl Pts',(-6.19294824148474,5.27914226898062,-1.02143551381684));
#42810=CARTESIAN_POINT('Ctrl Pts',(-6.21045140434731,5.10960376729697,-1.56645372157515));
#42811=CARTESIAN_POINT('Ctrl Pts',(-6.22297077464372,4.93337268328259,-1.93258635133501));
#42812=CARTESIAN_POINT('Ctrl Pts',(-6.23883466678608,4.62820099619023,-2.3787079638203));
#42813=CARTESIAN_POINT('Ctrl Pts',(-6.2427868842605,4.54408161512812,-2.48868157881534));
#42814=CARTESIAN_POINT('Ctrl Pts',(-6.25247848709626,4.32366283402261,-2.74731254107122));
#42815=CARTESIAN_POINT('Ctrl Pts',(-6.25823857463207,4.18208549069023,-2.88963895180828));
#42816=CARTESIAN_POINT('Ctrl Pts',(-6.2692813387163,3.90172397801768,-3.13164072520095));
#42817=CARTESIAN_POINT('Ctrl Pts',(-6.2744275556656,3.76670573621986,-3.23398973321062));
#42818=CARTESIAN_POINT('Ctrl Pts',(-6.29060925724983,3.32709283935529,-3.52600566838254));
#42819=CARTESIAN_POINT('Ctrl Pts',(-6.30178238136156,3.00176773346185,-3.68511173604148));
#42820=CARTESIAN_POINT('Ctrl Pts',(-6.31774503108853,2.49257762064374,-3.85413806611805));
#42821=CARTESIAN_POINT('Ctrl Pts',(-6.32284351431939,2.32099062755695,-3.89853576151291));
#42822=CARTESIAN_POINT('Ctrl Pts',(-6.33202810551563,2.00558964524924,-3.95766919450422));
#42823=CARTESIAN_POINT('Ctrl Pts',(-6.33612306616013,1.86369523672523,-3.97632621268576));
#42824=CARTESIAN_POINT('Ctrl Pts',(-6.34339855690956,1.61715754079666,-3.99507587614472));
#42825=CARTESIAN_POINT('Ctrl Pts',(-6.34649196870305,1.51356084580697,-3.99886470380823));
#42826=CARTESIAN_POINT('Ctrl Pts',(-6.34961610278363,1.4099734843268,-3.9986428669731));
#42827=CARTESIAN_POINT('Ctrl Pts',(-6.655829557301,-0.03671758326641,-3.24938089347));
#42828=CARTESIAN_POINT('Ctrl Pts',(-6.628746223968,0.7005435548854,-3.577630700739));
#42829=CARTESIAN_POINT('Ctrl Pts',(-6.574579557301,2.404033217635,-3.711199680242));
#42830=CARTESIAN_POINT('Ctrl Pts',(-6.493329557301,4.518613970016,-2.258507751061));
#42831=CARTESIAN_POINT('Ctrl Pts',(-6.412079557301,5.247018657974,0.2011050323816));
#42832=CARTESIAN_POINT('Ctrl Pts',(-6.330829557301,4.265405083671,2.571007123468));
#42833=CARTESIAN_POINT('Ctrl Pts',(-6.249579557301,2.011068327558,3.795011086251));
#42834=CARTESIAN_POINT('Ctrl Pts',(-6.168329557301,-0.5111570918951,3.327542458853));
#42835=CARTESIAN_POINT('Ctrl Pts',(-6.087079557301,-2.177110586008,1.376962753456));
#42836=CARTESIAN_POINT('Ctrl Pts',(-6.005829557301,-2.244259032195,-1.187340767628));
#42837=CARTESIAN_POINT('Ctrl Pts',(-5.924579557301,-0.6826749494628,-3.222436812587));
#42838=CARTESIAN_POINT('Ctrl Pts',(-5.843329557301,1.811631324597,-3.821266770609));
#42839=CARTESIAN_POINT('Ctrl Pts',(-5.762079557301,4.126927256222,-2.716927256679));
#42840=CARTESIAN_POINT('Ctrl Pts',(-5.680829557301,5.231266769463,-0.4016313216255));
#42841=CARTESIAN_POINT('Ctrl Pts',(-5.599579557301,4.632436817629,2.092674938032));
#42842=CARTESIAN_POINT('Ctrl Pts',(-5.518329557301,2.597340748606,3.654259074947));
#42843=CARTESIAN_POINT('Ctrl Pts',(-5.437079557301,0.03303731758841,3.587110426432));
#42844=CARTESIAN_POINT('Ctrl Pts',(-5.355829557301,-1.917542724007,1.921157687446));
#42845=CARTESIAN_POINT('Ctrl Pts',(-5.274579557301,-2.385010096676,-0.6010705501845));
#42846=CARTESIAN_POINT('Ctrl Pts',(-5.193329557301,-1.161010816611,-2.855396788715));
#42847=CARTESIAN_POINT('Ctrl Pts',(-5.112079557301,1.208908750616,-3.837049615173));
#42848=CARTESIAN_POINT('Ctrl Pts',(-5.030829557301,3.668456312214,-3.108498436179));
#42849=CARTESIAN_POINT('Ctrl Pts',(-4.949579557301,5.121391652629,-0.9944643957835));
#42850=CARTESIAN_POINT('Ctrl Pts',(-4.868329557301,4.920129760283,1.562810455248));
#42851=CARTESIAN_POINT('Ctrl Pts',(-4.787079557301,3.154374667059,3.423528074391));
#42852=CARTESIAN_POINT('Ctrl Pts',(-4.705829557301,0.611137751617,3.758351537704));
#42853=CARTESIAN_POINT('Ctrl Pts',(-4.624579557301,-1.576040017561,2.418047516939));
#42854=CARTESIAN_POINT('Ctrl Pts',(-4.543329557301,-2.432314847485,-3.831846085989E-7));
#42855=CARTESIAN_POINT('Ctrl Pts',(-4.462079557301,-1.576041844558,-2.418045984201));
#42856=CARTESIAN_POINT('Ctrl Pts',(-4.380829557301,0.6111450596018,-3.758356902288));
#42857=CARTESIAN_POINT('Ctrl Pts',(-4.299579557301,3.154347262116,-3.423508148791));
#42858=CARTESIAN_POINT('Ctrl Pts',(-4.218329557301,4.92023207207,-1.562884793063));
#42859=CARTESIAN_POINT('Ctrl Pts',(-4.137079557301,5.121009810423,0.9947418214435));
#42860=CARTESIAN_POINT('Ctrl Pts',(-4.082912890634,4.153590849641,2.403222654717));
#42861=CARTESIAN_POINT('Ctrl Pts',(-4.055829557301,3.500687608684,2.877584625945));
#42862=CARTESIAN_POINT('Ctrl Pts',(-6.562256554992,-0.1026386902142,-3.397442123851));
#42863=CARTESIAN_POINT('Ctrl Pts',(-6.535173221659,0.6682164754788,-3.740648955836));
#42864=CARTESIAN_POINT('Ctrl Pts',(-6.481006554992,2.449327317055,-3.880304137017));
#42865=CARTESIAN_POINT('Ctrl Pts',(-6.399756554992,4.660261017337,-2.361418873952));
#42866=CARTESIAN_POINT('Ctrl Pts',(-6.318506554992,5.421856179989,0.2102685806102));
#42867=CARTESIAN_POINT('Ctrl Pts',(-6.237256554992,4.395514419506,2.688157587048));
#42868=CARTESIAN_POINT('Ctrl Pts',(-6.156006554992,2.038456595982,3.96793449202));
#42869=CARTESIAN_POINT('Ctrl Pts',(-6.074756554992,-0.5986965008186,3.479165197693));
#42870=CARTESIAN_POINT('Ctrl Pts',(-5.993506554992,-2.340560801384,1.439705413104));
#42871=CARTESIAN_POINT('Ctrl Pts',(-5.912256554992,-2.410768932443,-1.241443115336));
#42872=CARTESIAN_POINT('Ctrl Pts',(-5.831006554992,-0.7780297379481,-3.369270309471));
#42873=CARTESIAN_POINT('Ctrl Pts',(-5.749756554992,1.829932050191,-3.995386542412));
#42874=CARTESIAN_POINT('Ctrl Pts',(-5.668506554992,4.250726713904,-2.840726714381));
#42875=CARTESIAN_POINT('Ctrl Pts',(-5.587256554992,5.405386541213,-0.4199320470834));
#42876=CARTESIAN_POINT('Ctrl Pts',(-5.506006554992,4.779270314743,2.188029725996));
#42877=CARTESIAN_POINT('Ctrl Pts',(-5.424756554992,2.651443095448,3.820768977142));
#42878=CARTESIAN_POINT('Ctrl Pts',(-5.343506554992,-0.02970533882238,3.750560634537));
#42879=CARTESIAN_POINT('Ctrl Pts',(-5.262256554992,-2.06916547493,2.008697123506));
#42880=CARTESIAN_POINT('Ctrl Pts',(-5.181006554992,-2.557933457354,-0.6284589198844));
#42881=CARTESIAN_POINT('Ctrl Pts',(-5.099756554992,-1.278161448473,-2.985505746582));
#42882=CARTESIAN_POINT('Ctrl Pts',(-5.018506554992,1.199745830423,-4.011888547782));
#42883=CARTESIAN_POINT('Ctrl Pts',(-4.937256554992,3.771365091244,-3.250140219087));
#42884=CARTESIAN_POINT('Ctrl Pts',(-4.856006554992,5.290504856815,-1.039778142259));
#42885=CARTESIAN_POINT('Ctrl Pts',(-4.774756554992,5.080072268762,1.634021447877));
#42886=CARTESIAN_POINT('Ctrl Pts',(-4.693506554992,3.233858811244,3.579524492034));
#42887=CARTESIAN_POINT('Ctrl Pts',(-4.612256554992,0.5747368090133,3.929604515154));
#42888=CARTESIAN_POINT('Ctrl Pts',(-4.531006554992,-1.712101862406,2.528228225885));
#42889=CARTESIAN_POINT('Ctrl Pts',(-4.449756554992,-2.607393695574,-4.006447915689E-7));
#42890=CARTESIAN_POINT('Ctrl Pts',(-4.368506554992,-1.712103772651,-2.528226623306));
#42891=CARTESIAN_POINT('Ctrl Pts',(-4.287256554992,0.5747444499936,-3.929610124181));
#42892=CARTESIAN_POINT('Ctrl Pts',(-4.206006554992,3.233830157568,-3.579503658505));
#42893=CARTESIAN_POINT('Ctrl Pts',(-4.124756554992,5.080179242486,-1.634099172968));
#42894=CARTESIAN_POINT('Ctrl Pts',(-4.043506554992,5.290105615594,1.040068209092));
#42895=CARTESIAN_POINT('Ctrl Pts',(-3.989339888326,4.278605260133,2.512727854262));
#42896=CARTESIAN_POINT('Ctrl Pts',(-3.962256554992,3.595951842036,3.008704594398));
#42897=CARTESIAN_POINT('Ctrl Pts',(-6.468683552684,-0.1685597971619,-3.545503354232));
#42898=CARTESIAN_POINT('Ctrl Pts',(-6.44160021935,0.6358893960722,-3.903667210934));
#42899=CARTESIAN_POINT('Ctrl Pts',(-6.387433552684,2.494621416475,-4.049408593792));
#42900=CARTESIAN_POINT('Ctrl Pts',(-6.306183552684,4.801908064657,-2.464329996843));
#42901=CARTESIAN_POINT('Ctrl Pts',(-6.224933552684,5.596693702003,0.2194321288388));
#42902=CARTESIAN_POINT('Ctrl Pts',(-6.143683552684,4.525623755341,2.805308050628));
#42903=CARTESIAN_POINT('Ctrl Pts',(-6.062433552684,2.065844864405,4.140857897789));
#42904=CARTESIAN_POINT('Ctrl Pts',(-5.981183552684,-0.686235909742,3.630787936533));
#42905=CARTESIAN_POINT('Ctrl Pts',(-5.899933552684,-2.504011016761,1.502448072752));
#42906=CARTESIAN_POINT('Ctrl Pts',(-5.818683552684,-2.57727883269,-1.295545463045));
#42907=CARTESIAN_POINT('Ctrl Pts',(-5.737433552684,-0.8733845264335,-3.516103806355));
#42908=CARTESIAN_POINT('Ctrl Pts',(-5.656183552684,1.848232775784,-4.169506314214));
#42909=CARTESIAN_POINT('Ctrl Pts',(-5.574933552684,4.374526171585,-2.964526172083));
#42910=CARTESIAN_POINT('Ctrl Pts',(-5.493683552684,5.579506312963,-0.4382327725412));
#42911=CARTESIAN_POINT('Ctrl Pts',(-5.412433552684,4.926103811857,2.283384513961));
#42912=CARTESIAN_POINT('Ctrl Pts',(-5.331183552684,2.70554544229,3.987278879338));
#42913=CARTESIAN_POINT('Ctrl Pts',(-5.249933552684,-0.09244799523316,3.914010842643));
#42914=CARTESIAN_POINT('Ctrl Pts',(-5.168683552684,-2.220788225852,2.096236559566));
#42915=CARTESIAN_POINT('Ctrl Pts',(-5.087433552684,-2.730856818033,-0.6558472895844));
#42916=CARTESIAN_POINT('Ctrl Pts',(-5.006183552684,-1.395312080335,-3.11561470445));
#42917=CARTESIAN_POINT('Ctrl Pts',(-4.924933552684,1.19058291023,-4.186727480392));
#42918=CARTESIAN_POINT('Ctrl Pts',(-4.843683552684,3.874273870273,-3.391782001995));
#42919=CARTESIAN_POINT('Ctrl Pts',(-4.762433552684,5.459618061001,-1.085091888735));
#42920=CARTESIAN_POINT('Ctrl Pts',(-4.681183552684,5.240014777241,1.705232440507));
#42921=CARTESIAN_POINT('Ctrl Pts',(-4.599933552684,3.31334295543,3.735520909677));
#42922=CARTESIAN_POINT('Ctrl Pts',(-4.518683552684,0.5383358664096,4.100857492604));
#42923=CARTESIAN_POINT('Ctrl Pts',(-4.437433552684,-1.84816370725,2.638408934831));
#42924=CARTESIAN_POINT('Ctrl Pts',(-4.356183552684,-2.782472543663,-4.181049747422E-7));
#42925=CARTESIAN_POINT('Ctrl Pts',(-4.274933552684,-1.848165700744,-2.638407262411));
#42926=CARTESIAN_POINT('Ctrl Pts',(-4.193683552684,0.5383438403855,-4.100863346074));
#42927=CARTESIAN_POINT('Ctrl Pts',(-4.112433552684,3.313313053021,-3.735499168218));
#42928=CARTESIAN_POINT('Ctrl Pts',(-4.031183552684,5.240126412902,-1.705313552873));
#42929=CARTESIAN_POINT('Ctrl Pts',(-3.949933552684,5.459201420765,1.08539459674));
#42930=CARTESIAN_POINT('Ctrl Pts',(-3.895766886017,4.403619670625,2.622233053807));
#42931=CARTESIAN_POINT('Ctrl Pts',(-3.868683552684,3.691216075387,3.139824562851));
#42932=CARTESIAN_POINT('Ctrl Pts',(-6.375110550375,-0.2344809041097,-3.693564584614));
#42933=CARTESIAN_POINT('Ctrl Pts',(-6.348027217042,0.6035623166656,-4.066685466031));
#42934=CARTESIAN_POINT('Ctrl Pts',(-6.293860550375,2.539915515895,-4.218513050568));
#42935=CARTESIAN_POINT('Ctrl Pts',(-6.212610550375,4.943555111978,-2.567241119733));
#42936=CARTESIAN_POINT('Ctrl Pts',(-6.131360550375,5.771531224017,0.2285956770673));
#42937=CARTESIAN_POINT('Ctrl Pts',(-6.050110550375,4.655733091177,2.922458514209));
#42938=CARTESIAN_POINT('Ctrl Pts',(-5.968860550375,2.093233132829,4.313781303558));
#42939=CARTESIAN_POINT('Ctrl Pts',(-5.887610550375,-0.7737753186654,3.782410675374));
#42940=CARTESIAN_POINT('Ctrl Pts',(-5.806360550375,-2.667461232137,1.5651907324));
#42941=CARTESIAN_POINT('Ctrl Pts',(-5.725110550375,-2.743788732938,-1.349647810754));
#42942=CARTESIAN_POINT('Ctrl Pts',(-5.643860550375,-0.9687393149189,-3.662937303239));
#42943=CARTESIAN_POINT('Ctrl Pts',(-5.562610550375,1.866533501377,-4.343626086017));
#42944=CARTESIAN_POINT('Ctrl Pts',(-5.481360550375,4.498325629267,-3.088325629786));
#42945=CARTESIAN_POINT('Ctrl Pts',(-5.400110550375,5.753626084714,-0.4565334979991));
#42946=CARTESIAN_POINT('Ctrl Pts',(-5.318860550375,5.072937308971,2.378739301925));
#42947=CARTESIAN_POINT('Ctrl Pts',(-5.237610550375,2.759647789132,4.153788781534));
#42948=CARTESIAN_POINT('Ctrl Pts',(-5.156360550375,-0.155190651644,4.077461050748));
#42949=CARTESIAN_POINT('Ctrl Pts',(-5.075110550375,-2.372410976774,2.183775995627));
#42950=CARTESIAN_POINT('Ctrl Pts',(-4.993860550375,-2.903780178711,-0.6832356592843));
#42951=CARTESIAN_POINT('Ctrl Pts',(-4.912610550375,-1.512462712197,-3.245723662317));
#42952=CARTESIAN_POINT('Ctrl Pts',(-4.831360550375,1.181419990037,-4.361566413001));
#42953=CARTESIAN_POINT('Ctrl Pts',(-4.750110550375,3.977182649303,-3.533423784903));
#42954=CARTESIAN_POINT('Ctrl Pts',(-4.668860550375,5.628731265186,-1.130405635211));
#42955=CARTESIAN_POINT('Ctrl Pts',(-4.587610550375,5.39995728572,1.776443433137));
#42956=CARTESIAN_POINT('Ctrl Pts',(-4.506360550375,3.392827099615,3.89151732732));
#42957=CARTESIAN_POINT('Ctrl Pts',(-4.425110550375,0.501934923806,4.272110470055));
#42958=CARTESIAN_POINT('Ctrl Pts',(-4.343860550375,-1.984225552094,2.748589643777));
#42959=CARTESIAN_POINT('Ctrl Pts',(-4.262610550375,-2.957551391752,-4.355651578303E-7));
#42960=CARTESIAN_POINT('Ctrl Pts',(-4.181360550375,-1.984227628837,-2.748587901516));
#42961=CARTESIAN_POINT('Ctrl Pts',(-4.100110550375,0.5019432307773,-4.272116567967));
#42962=CARTESIAN_POINT('Ctrl Pts',(-4.018860550375,3.392795948473,-3.891494677932));
#42963=CARTESIAN_POINT('Ctrl Pts',(-3.937610550375,5.400073583318,-1.776527932779));
#42964=CARTESIAN_POINT('Ctrl Pts',(-3.856360550375,5.628297225935,1.130720984389));
#42965=CARTESIAN_POINT('Ctrl Pts',(-3.802193883708,4.528634081117,2.731738253352));
#42966=CARTESIAN_POINT('Ctrl Pts',(-3.775110550375,3.786480308739,3.270944531304));
#42967=CARTESIAN_POINT('',(-4.08091832637295,4.52608525559028,1.79907266118024));
#42968=CARTESIAN_POINT('Ctrl Pts',(-4.0809183266954,4.52608525577217,1.79907266123773));
#42969=CARTESIAN_POINT('Ctrl Pts',(-4.04214744347317,4.58421161914435,1.83263193277767));
#42970=CARTESIAN_POINT('Ctrl Pts',(-4.00337656025091,4.64233798251616,1.86619120431821));
#42971=CARTESIAN_POINT('Ctrl Pts',(-3.92599972798394,4.75834343545228,1.93316698379834));
#42972=CARTESIAN_POINT('Ctrl Pts',(-3.88739377893924,4.81622252501658,1.96658349173795));
#42973=CARTESIAN_POINT('Ctrl Pts',(-3.84878782989446,4.8741016145805,1.99999999967813));
#42974=CARTESIAN_POINT('Ctrl Pts',(-6.58096181831254,1.41000211172738,-3.59814532525062));
#42975=CARTESIAN_POINT('Ctrl Pts',(-6.56844586670982,1.78745782164221,-3.59874070293084));
#42976=CARTESIAN_POINT('Ctrl Pts',(-6.55389861244537,2.23012749294581,-3.54264153998024));
#42977=CARTESIAN_POINT('Ctrl Pts',(-6.52143148332145,3.14211258271626,-3.18857913775972));
#42978=CARTESIAN_POINT('Ctrl Pts',(-6.50581496807022,3.54777649100928,-2.93114612264599));
#42979=CARTESIAN_POINT('Ctrl Pts',(-6.47436976361129,4.23674269123053,-2.27963350176037));
#42980=CARTESIAN_POINT('Ctrl Pts',(-6.45892749944977,4.50915827316548,-1.89158780048282));
#42981=CARTESIAN_POINT('Ctrl Pts',(-6.42787976811596,4.88602617929508,-1.03437663024274));
#42982=CARTESIAN_POINT('Ctrl Pts',(-6.41259810097365,4.99173694839489,-0.576725573750677));
#42983=CARTESIAN_POINT('Ctrl Pts',(-6.37894041754866,5.02689620983516,0.436826228201623));
#42984=CARTESIAN_POINT('Ctrl Pts',(-6.36328101540946,4.91393240444917,0.905683591418369));
#42985=CARTESIAN_POINT('Ctrl Pts',(-6.33547486496501,4.61718657022314,1.69044375960113));
#42986=CARTESIAN_POINT('Ctrl Pts',(-6.32056291466375,4.38093761369228,2.08235534769541));
#42987=CARTESIAN_POINT('Ctrl Pts',(-6.28981466176003,3.75934740684368,2.76895553999334));
#42988=CARTESIAN_POINT('Ctrl Pts',(-6.27401256964841,3.36694690053605,3.05577123496502));
#42989=CARTESIAN_POINT('Ctrl Pts',(-6.24528579717759,2.58249721445425,3.4243114842652));
#42990=CARTESIAN_POINT('Ctrl Pts',(-6.22998723185367,2.13443855169956,3.56796020431119));
#42991=CARTESIAN_POINT('Ctrl Pts',(-6.19651879481664,1.12707558514787,3.61776937546146));
#42992=CARTESIAN_POINT('Ctrl Pts',(-6.18090280181225,0.651773498828013,
3.54790362030401));
#42993=CARTESIAN_POINT('Ctrl Pts',(-6.1494553479069,-0.242842272609004,
3.23348418370255));
#42994=CARTESIAN_POINT('Ctrl Pts',(-6.13400985998153,-0.649778439883511,
2.99000998636926));
#42995=CARTESIAN_POINT('Ctrl Pts',(-6.10295652168396,-1.34324643751278,
2.36052473298331));
#42996=CARTESIAN_POINT('Ctrl Pts',(-6.08767324940502,-1.62623604957388,
1.98558191396073));
#42997=CARTESIAN_POINT('Ctrl Pts',(-6.05402240736802,-2.07110679903882,
1.0744400426321));
#42998=CARTESIAN_POINT('Ctrl Pts',(-6.03836750072588,-2.15897813573258,
0.600392684303999));
#42999=CARTESIAN_POINT('Ctrl Pts',(-6.01055544369523,-2.20763567912064,
-0.237365748009926));
#43000=CARTESIAN_POINT('Ctrl Pts',(-5.99564682586976,-2.1515101612092,-0.691423320158894));
#43001=CARTESIAN_POINT('Ctrl Pts',(-5.96490396330907,-1.86366136469892,
-1.57156326080984));
#43002=CARTESIAN_POINT('Ctrl Pts',(-5.94910111676084,-1.62213891078369,
-1.99337880265138));
#43003=CARTESIAN_POINT('Ctrl Pts',(-5.92038172893592,-1.05602558623955,
-2.64936192882865));
#43004=CARTESIAN_POINT('Ctrl Pts',(-5.90508398769301,-0.705426956801211,
-2.96312899578154));
#43005=CARTESIAN_POINT('Ctrl Pts',(-5.87161360411978,0.194258412510714,
-3.41912431062218));
#43006=CARTESIAN_POINT('Ctrl Pts',(-5.85599554789065,0.656850288984242,
-3.54898770846588));
#43007=CARTESIAN_POINT('Ctrl Pts',(-5.82454904505799,1.60192740622799,-3.62633630936245));
#43008=CARTESIAN_POINT('Ctrl Pts',(-5.80910652452517,2.07266918334268,-3.56984723484898));
#43009=CARTESIAN_POINT('Ctrl Pts',(-5.77804979542462,2.962544241391,-3.2775218934811));
#43010=CARTESIAN_POINT('Ctrl Pts',(-5.76276355706507,3.3738234029449,-3.05035443589435));
#43011=CARTESIAN_POINT('Ctrl Pts',(-5.7291162063491,4.15123456413457,-2.3995716592242));
#43012=CARTESIAN_POINT('Ctrl Pts',(-5.71346469756639,4.42461826958582,-2.00259179169693));
#43013=CARTESIAN_POINT('Ctrl Pts',(-5.68564692764332,4.81044759733957,-1.25718605363807));
#43014=CARTESIAN_POINT('Ctrl Pts',(-5.6707424649409,4.94413068178707,-0.819773855555241));
#43015=CARTESIAN_POINT('Ctrl Pts',(-5.64000600973413,5.0399590726211,0.101074923696168));
#43016=CARTESIAN_POINT('Ctrl Pts',(-5.62420228432147,4.99128197185479,0.584723013700979));
#43017=CARTESIAN_POINT('Ctrl Pts',(-5.59549084818378,4.74167646430499,1.41423121271074));
#43018=CARTESIAN_POINT('Ctrl Pts',(-5.58019418646508,4.54945191106595,1.84363856859814));
#43019=CARTESIAN_POINT('Ctrl Pts',(-5.5467221440927,3.91372603349255,2.6267764931748));
#43020=CARTESIAN_POINT('Ctrl Pts',(-5.53110175186135,3.5441559662154,2.93393145271935));
#43021=CARTESIAN_POINT('Ctrl Pts',(-5.49965634959531,2.71266299551641,3.38969639168488));
#43022=CARTESIAN_POINT('Ctrl Pts',(-5.4842171998763,2.25988270259248,3.52997791484526));
#43023=CARTESIAN_POINT('Ctrl Pts',(-5.45315659758382,1.32801856216453,3.62573247975942));
#43024=CARTESIAN_POINT('Ctrl Pts',(-5.43786697424592,0.859755722308295,
3.58587428719093));
#43025=CARTESIAN_POINT('Ctrl Pts',(-5.40422322792756,-0.115279376707325,
3.30841367623825));
#43026=CARTESIAN_POINT('Ctrl Pts',(-5.38857555087741,-0.526643436121224,
3.05744210709078));
#43027=CARTESIAN_POINT('Ctrl Pts',(-5.36075164923175,-1.18288818883317,
2.53385355868996));
#43028=CARTESIAN_POINT('Ctrl Pts',(-5.34585197180141,-1.48310920504433,
2.18898786501864));
#43029=CARTESIAN_POINT('Ctrl Pts',(-5.31602824355059,-1.932273702204,1.41101213498186));
#43030=CARTESIAN_POINT('Ctrl Pts',(-5.30112856612032,-2.08082564571144,
0.978580261357411));
#43031=CARTESIAN_POINT('Ctrl Pts',(-5.27330466447475,-2.20614425340107,
0.148461360208153));
#43032=CARTESIAN_POINT('Ctrl Pts',(-5.25765698742468,-2.21780997820335,
-0.33327615002195));
#43033=CARTESIAN_POINT('Ctrl Pts',(-5.22401324110646,-1.97058036632985,
-1.31641162082765));
#43034=CARTESIAN_POINT('Ctrl Pts',(-5.20872361776865,-1.77096715371478,
-1.74186823207588));
#43035=CARTESIAN_POINT('Ctrl Pts',(-5.17766301547623,-1.22210919775635,
-2.5010089681056));
#43036=CARTESIAN_POINT('Ctrl Pts',(-5.16222386575719,-0.874231688555634,
-2.82298744253069));
#43037=CARTESIAN_POINT('Ctrl Pts',(-5.13077846349123,-0.0637811879073495,
-3.31519900874147));
#43038=CARTESIAN_POINT('Ctrl Pts',(-5.11515807126,0.387007843595224,-3.48167859570945));
#43039=CARTESIAN_POINT('Ctrl Pts',(-5.08168602888781,1.38308811973195,-3.64066439324238));
#43040=CARTESIAN_POINT('Ctrl Pts',(-5.06638936716926,1.85107807512151,-3.59243206163465));
#43041=CARTESIAN_POINT('Ctrl Pts',(-5.03767793103155,2.69425600188593,-3.39384267259227));
#43042=CARTESIAN_POINT('Ctrl Pts',(-5.02187420561876,3.13744608470504,-3.19417423343594));
#43043=CARTESIAN_POINT('Ctrl Pts',(-4.9911377504119,3.88701032516357,-2.65076002294398));
#43044=CARTESIAN_POINT('Ctrl Pts',(-4.97623328770948,4.19897885840476,-2.31628097671466));
#43045=CARTESIAN_POINT('Ctrl Pts',(-4.94841551778642,4.65160449981345,-1.60944010832522));
#43046=CARTESIAN_POINT('Ctrl Pts',(-4.93276400900382,4.85870729715726,-1.17419294066014));
#43047=CARTESIAN_POINT('Ctrl Pts',(-4.89911665828775,5.0335961335039,-0.175543737549332));
#43048=CARTESIAN_POINT('Ctrl Pts',(-4.88383041992803,5.02468934191009,0.294218193196915));
#43049=CARTESIAN_POINT('Ctrl Pts',(-4.85277369082731,4.83291298468031,1.21103527034498));
#43050=CARTESIAN_POINT('Ctrl Pts',(-4.83733117029437,4.64646306968778,1.6469541452058));
#43051=CARTESIAN_POINT('Ctrl Pts',(-4.80588466746181,4.10693865774205,2.42674063682608));
#43052=CARTESIAN_POINT('Ctrl Pts',(-4.79026661123289,3.76317771795078,2.7624252545146));
#43053=CARTESIAN_POINT('Ctrl Pts',(-4.7567962276597,2.91843150663598,3.3135779823315));
#43054=CARTESIAN_POINT('Ctrl Pts',(-4.74149848641669,2.47140194106464,3.46032176848061));
#43055=CARTESIAN_POINT('Ctrl Pts',(-4.71277909859167,1.62024722706906,3.62259872586796));
#43056=CARTESIAN_POINT('Ctrl Pts',(-4.69697625204335,1.13418302516555,3.62085553562207));
#43057=CARTESIAN_POINT('Ctrl Pts',(-4.6662333894826,0.228035079421316,3.43006993552313));
#43058=CARTESIAN_POINT('Ctrl Pts',(-4.65132477165713,-0.193253071796144,
3.25164727376046));
#43059=CARTESIAN_POINT('Ctrl Pts',(-4.62351271462644,-0.8944443847206,2.79062938894352));
#43060=CARTESIAN_POINT('Ctrl Pts',(-4.60785780798426,-1.26104577128261,
2.47750689993816));
#43061=CARTESIAN_POINT('Ctrl Pts',(-4.57420696594723,-1.8276824035723,1.63666659383647));
#43062=CARTESIAN_POINT('Ctrl Pts',(-4.55892369366826,-2.01089760378185,
1.20411899127301));
#43063=CARTESIAN_POINT('Ctrl Pts',(-4.52787035537078,-2.20931382570703,
0.288815461921373));
#43064=CARTESIAN_POINT('Ctrl Pts',(-4.51242486744549,-2.21670058212636,
-0.185338695323704));
#43065=CARTESIAN_POINT('Ctrl Pts',(-4.48097741354048,-2.04168791594811,
-1.11730839831501));
#43066=CARTESIAN_POINT('Ctrl Pts',(-4.46536142053643,-1.86454239160906,
-1.56386495711831));
#43067=CARTESIAN_POINT('Ctrl Pts',(-4.43189298349968,-1.31772490077559,
-2.41136229140832));
#43068=CARTESIAN_POINT('Ctrl Pts',(-4.4165944181758,-0.969292128617316,
-2.72756811571645));
#43069=CARTESIAN_POINT('Ctrl Pts',(-4.38786764570481,-0.257902067365425,
-3.22265134720374));
#43070=CARTESIAN_POINT('Ctrl Pts',(-4.3720655535929,0.186687863837912,-3.41907230663807));
#43071=CARTESIAN_POINT('Ctrl Pts',(-4.34131730068888,1.09209617603561,-3.61408512036354));
#43072=CARTESIAN_POINT('Ctrl Pts',(-4.32640535038746,1.54962604562836,-3.62272692428965));
#43073=CARTESIAN_POINT('Ctrl Pts',(-4.29859919994289,2.37762120426604,-3.48733627110506));
#43074=CARTESIAN_POINT('Ctrl Pts',(-4.28293979780371,2.84014549425617,-3.35073711466903));
#43075=CARTESIAN_POINT('Ctrl Pts',(-4.24928211437871,3.70032747207834,-2.81351240010709));
#43076=CARTESIAN_POINT('Ctrl Pts',(-4.2340004472364,4.04380952851942,-2.49313866036689));
#43077=CARTESIAN_POINT('Ctrl Pts',(-4.20295271590267,4.59774222529018,-1.73815589466744));
#43078=CARTESIAN_POINT('Ctrl Pts',(-4.18751045174126,4.79759186945824,-1.3082142296864));
#43079=CARTESIAN_POINT('Ctrl Pts',(-4.1560652472825,5.01733524992041,-0.385795687503433));
#43080=CARTESIAN_POINT('Ctrl Pts',(-4.14044873203137,5.03744682663507,0.0942360700334427));
#43081=CARTESIAN_POINT('Ctrl Pts',(-4.10798155174798,4.88808108123792,1.0610710502257));
#43082=CARTESIAN_POINT('Ctrl Pts',(-4.09343427343297,4.71532883305283,1.4724843596549));
#43083=CARTESIAN_POINT('Ctrl Pts',(-4.08091832701493,4.52608525525901,1.79907266101289));
#43084=CARTESIAN_POINT('Ctrl Pts',(-6.968838791574,-0.05425191507289,-3.288763647513));
#43085=CARTESIAN_POINT('Ctrl Pts',(-6.941755458241,0.6919448865242,-3.62099186847));
#43086=CARTESIAN_POINT('Ctrl Pts',(-6.887588791574,2.41608097904,-3.756179714594));
#43087=CARTESIAN_POINT('Ctrl Pts',(-6.806338791574,4.556290617787,-2.28588104406));
#43088=CARTESIAN_POINT('Ctrl Pts',(-6.725088791574,5.293523628312,0.2035424413179));
#43089=CARTESIAN_POINT('Ctrl Pts',(-6.643838791574,4.300012819665,2.602167933636));
#43090=CARTESIAN_POINT('Ctrl Pts',(-6.562588791574,2.018353323341,3.841006921488));
#43091=CARTESIAN_POINT('Ctrl Pts',(-6.481338791574,-0.5344416681603,3.367872537265));
#43092=CARTESIAN_POINT('Ctrl Pts',(-6.400088791574,-2.2205866507,1.393651651195));
#43093=CARTESIAN_POINT('Ctrl Pts',(-6.318838791574,-2.288548941379,-1.201731431865));
#43094=CARTESIAN_POINT('Ctrl Pts',(-6.237588791574,-0.7080383357597,-3.261493002233));
#43095=CARTESIAN_POINT('Ctrl Pts',(-6.156338791574,1.816499128093,-3.867580826823));
#43096=CARTESIAN_POINT('Ctrl Pts',(-6.075088791574,4.159856629968,-2.74985663043));
#43097=CARTESIAN_POINT('Ctrl Pts',(-5.993838791574,5.277580825662,-0.4064991250853));
#43098=CARTESIAN_POINT('Ctrl Pts',(-5.912588791574,4.671493007336,2.11803832419));
#43099=CARTESIAN_POINT('Ctrl Pts',(-5.831338791574,2.611731412613,3.698548984649));
#43100=CARTESIAN_POINT('Ctrl Pts',(-5.750088791574,0.01634842071054,3.630586489191));
#43101=CARTESIAN_POINT('Ctrl Pts',(-5.668838791574,-1.957872805634,1.944442270929));
#43102=CARTESIAN_POINT('Ctrl Pts',(-5.587588791574,-2.43100591992,-0.6083555729063));
#43103=CARTESIAN_POINT('Ctrl Pts',(-5.506338791574,-1.19217167154,-2.890004424173));
#43104=CARTESIAN_POINT('Ctrl Pts',(-5.425088791574,1.20647150873,-3.883554960714));
#43105=CARTESIAN_POINT('Ctrl Pts',(-5.343838791574,3.695828981771,-3.146173683671));
#43106=CARTESIAN_POINT('Ctrl Pts',(-5.262588791574,5.166374013702,-1.006517383103));
#43107=CARTESIAN_POINT('Ctrl Pts',(-5.181338791574,4.962672811265,1.581751841867));
#43108=CARTESIAN_POINT('Ctrl Pts',(-5.100088791574,3.175516626319,3.465021506074));
#43109=CARTESIAN_POINT('Ctrl Pts',(-5.018838791574,0.6014554778319,3.803903056307));
#43110=CARTESIAN_POINT('Ctrl Pts',(-4.937588791574,-1.612231059311,2.44735444455));
#43111=CARTESIAN_POINT('Ctrl Pts',(-4.856338791574,-2.47888400806,-3.87828836268E-7));
#43112=CARTESIAN_POINT('Ctrl Pts',(-4.775088791574,-1.61223290845,-2.447352893234));
#43113=CARTESIAN_POINT('Ctrl Pts',(-4.693838791574,0.6014628743901,-3.80390848591));
#43114=CARTESIAN_POINT('Ctrl Pts',(-4.612588791574,3.175488889226,-3.465001338974));
#43115=CARTESIAN_POINT('Ctrl Pts',(-4.531338791574,4.962776363079,-1.581827080662));
#43116=CARTESIAN_POINT('Ctrl Pts',(-4.450088791574,5.165987543538,1.006798171184));
#43117=CARTESIAN_POINT('Ctrl Pts',(-4.395922124908,4.186843388254,2.432349903822));
#43118=CARTESIAN_POINT('Ctrl Pts',(-4.368838791574,3.526026908253,2.91246117975));
#43119=CARTESIAN_POINT('Ctrl Pts',(-6.839612930525,-0.05425191507289,-3.288763647513));
#43120=CARTESIAN_POINT('Ctrl Pts',(-6.812529597191,0.6919448865242,-3.62099186847));
#43121=CARTESIAN_POINT('Ctrl Pts',(-6.758362930525,2.41608097904,-3.756179714594));
#43122=CARTESIAN_POINT('Ctrl Pts',(-6.677112930525,4.556290617787,-2.28588104406));
#43123=CARTESIAN_POINT('Ctrl Pts',(-6.595862930525,5.293523628312,0.2035424413179));
#43124=CARTESIAN_POINT('Ctrl Pts',(-6.514612930525,4.300012819665,2.602167933636));
#43125=CARTESIAN_POINT('Ctrl Pts',(-6.433362930525,2.018353323341,3.841006921488));
#43126=CARTESIAN_POINT('Ctrl Pts',(-6.352112930525,-0.5344416681603,3.367872537265));
#43127=CARTESIAN_POINT('Ctrl Pts',(-6.270862930525,-2.2205866507,1.393651651195));
#43128=CARTESIAN_POINT('Ctrl Pts',(-6.189612930525,-2.288548941379,-1.201731431865));
#43129=CARTESIAN_POINT('Ctrl Pts',(-6.108362930525,-0.7080383357597,-3.261493002233));
#43130=CARTESIAN_POINT('Ctrl Pts',(-6.027112930525,1.816499128093,-3.867580826823));
#43131=CARTESIAN_POINT('Ctrl Pts',(-5.945862930525,4.159856629968,-2.74985663043));
#43132=CARTESIAN_POINT('Ctrl Pts',(-5.864612930525,5.277580825662,-0.4064991250853));
#43133=CARTESIAN_POINT('Ctrl Pts',(-5.783362930525,4.671493007336,2.11803832419));
#43134=CARTESIAN_POINT('Ctrl Pts',(-5.702112930525,2.611731412613,3.698548984649));
#43135=CARTESIAN_POINT('Ctrl Pts',(-5.620862930525,0.01634842071054,3.630586489191));
#43136=CARTESIAN_POINT('Ctrl Pts',(-5.539612930525,-1.957872805634,1.944442270929));
#43137=CARTESIAN_POINT('Ctrl Pts',(-5.458362930525,-2.43100591992,-0.6083555729063));
#43138=CARTESIAN_POINT('Ctrl Pts',(-5.377112930525,-1.19217167154,-2.890004424173));
#43139=CARTESIAN_POINT('Ctrl Pts',(-5.295862930525,1.20647150873,-3.883554960714));
#43140=CARTESIAN_POINT('Ctrl Pts',(-5.214612930525,3.695828981771,-3.146173683671));
#43141=CARTESIAN_POINT('Ctrl Pts',(-5.133362930525,5.166374013702,-1.006517383103));
#43142=CARTESIAN_POINT('Ctrl Pts',(-5.052112930525,4.962672811265,1.581751841867));
#43143=CARTESIAN_POINT('Ctrl Pts',(-4.970862930525,3.175516626319,3.465021506074));
#43144=CARTESIAN_POINT('Ctrl Pts',(-4.889612930525,0.6014554778319,3.803903056307));
#43145=CARTESIAN_POINT('Ctrl Pts',(-4.808362930525,-1.612231059311,2.44735444455));
#43146=CARTESIAN_POINT('Ctrl Pts',(-4.727112930525,-2.47888400806,-3.87828836268E-7));
#43147=CARTESIAN_POINT('Ctrl Pts',(-4.645862930525,-1.61223290845,-2.447352893234));
#43148=CARTESIAN_POINT('Ctrl Pts',(-4.564612930525,0.6014628743901,-3.80390848591));
#43149=CARTESIAN_POINT('Ctrl Pts',(-4.483362930525,3.175488889226,-3.465001338974));
#43150=CARTESIAN_POINT('Ctrl Pts',(-4.402112930525,4.962776363079,-1.581827080662));
#43151=CARTESIAN_POINT('Ctrl Pts',(-4.320862930525,5.165987543538,1.006798171184));
#43152=CARTESIAN_POINT('Ctrl Pts',(-4.266696263858,4.186843388254,2.432349903822));
#43153=CARTESIAN_POINT('Ctrl Pts',(-4.239612930525,3.526026908253,2.91246117975));
#43154=CARTESIAN_POINT('Ctrl Pts',(-6.710387069475,-0.05425191507289,-3.288763647513));
#43155=CARTESIAN_POINT('Ctrl Pts',(-6.683303736142,0.6919448865242,-3.62099186847));
#43156=CARTESIAN_POINT('Ctrl Pts',(-6.629137069475,2.41608097904,-3.756179714594));
#43157=CARTESIAN_POINT('Ctrl Pts',(-6.547887069475,4.556290617787,-2.28588104406));
#43158=CARTESIAN_POINT('Ctrl Pts',(-6.466637069475,5.293523628312,0.2035424413179));
#43159=CARTESIAN_POINT('Ctrl Pts',(-6.385387069475,4.300012819665,2.602167933636));
#43160=CARTESIAN_POINT('Ctrl Pts',(-6.304137069475,2.018353323341,3.841006921488));
#43161=CARTESIAN_POINT('Ctrl Pts',(-6.222887069475,-0.5344416681603,3.367872537265));
#43162=CARTESIAN_POINT('Ctrl Pts',(-6.141637069475,-2.2205866507,1.393651651195));
#43163=CARTESIAN_POINT('Ctrl Pts',(-6.060387069475,-2.288548941379,-1.201731431865));
#43164=CARTESIAN_POINT('Ctrl Pts',(-5.979137069475,-0.7080383357597,-3.261493002233));
#43165=CARTESIAN_POINT('Ctrl Pts',(-5.897887069475,1.816499128093,-3.867580826823));
#43166=CARTESIAN_POINT('Ctrl Pts',(-5.816637069475,4.159856629968,-2.74985663043));
#43167=CARTESIAN_POINT('Ctrl Pts',(-5.735387069475,5.277580825662,-0.4064991250853));
#43168=CARTESIAN_POINT('Ctrl Pts',(-5.654137069475,4.671493007336,2.11803832419));
#43169=CARTESIAN_POINT('Ctrl Pts',(-5.572887069475,2.611731412613,3.698548984649));
#43170=CARTESIAN_POINT('Ctrl Pts',(-5.491637069475,0.01634842071054,3.630586489191));
#43171=CARTESIAN_POINT('Ctrl Pts',(-5.410387069475,-1.957872805634,1.944442270929));
#43172=CARTESIAN_POINT('Ctrl Pts',(-5.329137069475,-2.43100591992,-0.6083555729063));
#43173=CARTESIAN_POINT('Ctrl Pts',(-5.247887069475,-1.19217167154,-2.890004424173));
#43174=CARTESIAN_POINT('Ctrl Pts',(-5.166637069475,1.20647150873,-3.883554960714));
#43175=CARTESIAN_POINT('Ctrl Pts',(-5.085387069475,3.695828981771,-3.146173683671));
#43176=CARTESIAN_POINT('Ctrl Pts',(-5.004137069475,5.166374013702,-1.006517383103));
#43177=CARTESIAN_POINT('Ctrl Pts',(-4.922887069475,4.962672811265,1.581751841867));
#43178=CARTESIAN_POINT('Ctrl Pts',(-4.841637069475,3.175516626319,3.465021506074));
#43179=CARTESIAN_POINT('Ctrl Pts',(-4.760387069475,0.6014554778319,3.803903056307));
#43180=CARTESIAN_POINT('Ctrl Pts',(-4.679137069475,-1.612231059311,2.44735444455));
#43181=CARTESIAN_POINT('Ctrl Pts',(-4.597887069475,-2.47888400806,-3.87828836268E-7));
#43182=CARTESIAN_POINT('Ctrl Pts',(-4.516637069475,-1.61223290845,-2.447352893234));
#43183=CARTESIAN_POINT('Ctrl Pts',(-4.435387069475,0.6014628743901,-3.80390848591));
#43184=CARTESIAN_POINT('Ctrl Pts',(-4.354137069475,3.175488889226,-3.465001338974));
#43185=CARTESIAN_POINT('Ctrl Pts',(-4.272887069475,4.962776363079,-1.581827080662));
#43186=CARTESIAN_POINT('Ctrl Pts',(-4.191637069475,5.165987543538,1.006798171184));
#43187=CARTESIAN_POINT('Ctrl Pts',(-4.137470402809,4.186843388254,2.432349903822));
#43188=CARTESIAN_POINT('Ctrl Pts',(-4.110387069475,3.526026908253,2.91246117975));
#43189=CARTESIAN_POINT('Ctrl Pts',(-6.581161208426,-0.05425191507289,-3.288763647513));
#43190=CARTESIAN_POINT('Ctrl Pts',(-6.554077875092,0.6919448865242,-3.62099186847));
#43191=CARTESIAN_POINT('Ctrl Pts',(-6.499911208426,2.41608097904,-3.756179714594));
#43192=CARTESIAN_POINT('Ctrl Pts',(-6.418661208426,4.556290617787,-2.28588104406));
#43193=CARTESIAN_POINT('Ctrl Pts',(-6.337411208426,5.293523628312,0.2035424413179));
#43194=CARTESIAN_POINT('Ctrl Pts',(-6.256161208426,4.300012819665,2.602167933636));
#43195=CARTESIAN_POINT('Ctrl Pts',(-6.174911208426,2.018353323341,3.841006921488));
#43196=CARTESIAN_POINT('Ctrl Pts',(-6.093661208426,-0.5344416681603,3.367872537265));
#43197=CARTESIAN_POINT('Ctrl Pts',(-6.012411208426,-2.2205866507,1.393651651195));
#43198=CARTESIAN_POINT('Ctrl Pts',(-5.931161208426,-2.288548941379,-1.201731431865));
#43199=CARTESIAN_POINT('Ctrl Pts',(-5.849911208426,-0.7080383357597,-3.261493002233));
#43200=CARTESIAN_POINT('Ctrl Pts',(-5.768661208426,1.816499128093,-3.867580826823));
#43201=CARTESIAN_POINT('Ctrl Pts',(-5.687411208426,4.159856629968,-2.74985663043));
#43202=CARTESIAN_POINT('Ctrl Pts',(-5.606161208426,5.277580825662,-0.4064991250853));
#43203=CARTESIAN_POINT('Ctrl Pts',(-5.524911208426,4.671493007336,2.11803832419));
#43204=CARTESIAN_POINT('Ctrl Pts',(-5.443661208426,2.611731412613,3.698548984649));
#43205=CARTESIAN_POINT('Ctrl Pts',(-5.362411208426,0.01634842071054,3.630586489191));
#43206=CARTESIAN_POINT('Ctrl Pts',(-5.281161208426,-1.957872805634,1.944442270929));
#43207=CARTESIAN_POINT('Ctrl Pts',(-5.199911208426,-2.43100591992,-0.6083555729063));
#43208=CARTESIAN_POINT('Ctrl Pts',(-5.118661208426,-1.19217167154,-2.890004424173));
#43209=CARTESIAN_POINT('Ctrl Pts',(-5.037411208426,1.20647150873,-3.883554960714));
#43210=CARTESIAN_POINT('Ctrl Pts',(-4.956161208426,3.695828981771,-3.146173683671));
#43211=CARTESIAN_POINT('Ctrl Pts',(-4.874911208426,5.166374013702,-1.006517383103));
#43212=CARTESIAN_POINT('Ctrl Pts',(-4.793661208426,4.962672811265,1.581751841867));
#43213=CARTESIAN_POINT('Ctrl Pts',(-4.712411208426,3.175516626319,3.465021506074));
#43214=CARTESIAN_POINT('Ctrl Pts',(-4.631161208426,0.6014554778319,3.803903056307));
#43215=CARTESIAN_POINT('Ctrl Pts',(-4.549911208426,-1.612231059311,2.44735444455));
#43216=CARTESIAN_POINT('Ctrl Pts',(-4.468661208426,-2.47888400806,-3.87828836268E-7));
#43217=CARTESIAN_POINT('Ctrl Pts',(-4.387411208426,-1.61223290845,-2.447352893234));
#43218=CARTESIAN_POINT('Ctrl Pts',(-4.306161208426,0.6014628743901,-3.80390848591));
#43219=CARTESIAN_POINT('Ctrl Pts',(-4.224911208426,3.175488889226,-3.465001338974));
#43220=CARTESIAN_POINT('Ctrl Pts',(-4.143661208426,4.962776363079,-1.581827080662));
#43221=CARTESIAN_POINT('Ctrl Pts',(-4.062411208426,5.165987543538,1.006798171184));
#43222=CARTESIAN_POINT('Ctrl Pts',(-4.008244541759,4.186843388254,2.432349903822));
#43223=CARTESIAN_POINT('Ctrl Pts',(-3.981161208426,3.526026908253,2.91246117975));
#43224=CARTESIAN_POINT('',(-6.869059892324,1.41,-3.6));
#43225=CARTESIAN_POINT('Ctrl Pts',(-4.36903811233822,4.52608525529002,1.79907266095937));
#43226=CARTESIAN_POINT('Ctrl Pts',(-4.32102540822548,4.52608525529002,1.79907266095937));
#43227=CARTESIAN_POINT('Ctrl Pts',(-4.27301270411274,4.52608525529002,1.79907266095937));
#43228=CARTESIAN_POINT('Ctrl Pts',(-4.17697277545765,4.52608525529002,1.79907266095937));
#43229=CARTESIAN_POINT('Ctrl Pts',(-4.1289455509153,4.52608525529002,1.79907266095937));
#43230=CARTESIAN_POINT('Ctrl Pts',(-4.08091832637295,4.52608525529002,1.79907266095937));
#43231=CARTESIAN_POINT('Ctrl Pts',(-9.468838791574,-0.7060269082529,2.91246117975));
#43232=CARTESIAN_POINT('Ctrl Pts',(-9.441755458241,-1.366843388254,2.432349903822));
#43233=CARTESIAN_POINT('Ctrl Pts',(-9.387588791574,-2.345987543538,1.006798171184));
#43234=CARTESIAN_POINT('Ctrl Pts',(-9.306338791574,-2.142776363079,-1.581827080662));
#43235=CARTESIAN_POINT('Ctrl Pts',(-9.225088791574,-0.3554888892263,-3.465001338974));
#43236=CARTESIAN_POINT('Ctrl Pts',(-9.143838791574,2.21853712561,-3.80390848591));
#43237=CARTESIAN_POINT('Ctrl Pts',(-9.062588791574,4.43223290845,-2.447352893234));
#43238=CARTESIAN_POINT('Ctrl Pts',(-8.981338791574,5.29888400806,-3.878288208359E-7));
#43239=CARTESIAN_POINT('Ctrl Pts',(-8.900088791574,4.432231059311,2.44735444455));
#43240=CARTESIAN_POINT('Ctrl Pts',(-8.818838791574,2.218544522168,3.803903056307));
#43241=CARTESIAN_POINT('Ctrl Pts',(-8.737588791574,-0.3555166263194,3.465021506074));
#43242=CARTESIAN_POINT('Ctrl Pts',(-8.656338791574,-2.142672811265,1.581751841867));
#43243=CARTESIAN_POINT('Ctrl Pts',(-8.575088791574,-2.346374013702,-1.006517383103));
#43244=CARTESIAN_POINT('Ctrl Pts',(-8.493838791574,-0.8758289817713,-3.146173683671));
#43245=CARTESIAN_POINT('Ctrl Pts',(-8.412588791574,1.61352849127,-3.883554960714));
#43246=CARTESIAN_POINT('Ctrl Pts',(-8.331338791574,4.01217167154,-2.890004424173));
#43247=CARTESIAN_POINT('Ctrl Pts',(-8.250088791574,5.25100591992,-0.6083555729063));
#43248=CARTESIAN_POINT('Ctrl Pts',(-8.168838791574,4.777872805634,1.944442270929));
#43249=CARTESIAN_POINT('Ctrl Pts',(-8.087588791574,2.803651579289,3.63058648919));
#43250=CARTESIAN_POINT('Ctrl Pts',(-8.006338791574,0.208268587387,3.698548984649));
#43251=CARTESIAN_POINT('Ctrl Pts',(-7.925088791574,-1.851493007336,2.11803832419));
#43252=CARTESIAN_POINT('Ctrl Pts',(-7.843838791574,-2.457580825662,-0.4064991250853));
#43253=CARTESIAN_POINT('Ctrl Pts',(-7.762588791574,-1.339856629968,-2.74985663043));
#43254=CARTESIAN_POINT('Ctrl Pts',(-7.681338791574,1.003500871907,-3.867580826823));
#43255=CARTESIAN_POINT('Ctrl Pts',(-7.600088791574,3.52803833576,-3.261493002233));
#43256=CARTESIAN_POINT('Ctrl Pts',(-7.518838791574,5.108548941379,-1.201731431865));
#43257=CARTESIAN_POINT('Ctrl Pts',(-7.437588791574,5.0405866507,1.393651651195));
#43258=CARTESIAN_POINT('Ctrl Pts',(-7.356338791574,3.35444166816,3.367872537265));
#43259=CARTESIAN_POINT('Ctrl Pts',(-7.275088791574,0.8016466766589,3.841006921488));
#43260=CARTESIAN_POINT('Ctrl Pts',(-7.193838791574,-1.480012819665,2.602167933636));
#43261=CARTESIAN_POINT('Ctrl Pts',(-7.112588791574,-2.473523628312,0.203542441318));
#43262=CARTESIAN_POINT('Ctrl Pts',(-7.031338791574,-1.736290617787,-2.28588104406));
#43263=CARTESIAN_POINT('Ctrl Pts',(-6.950088791574,0.4039190209595,-3.756179714594));
#43264=CARTESIAN_POINT('Ctrl Pts',(-6.895922124908,2.128055113476,-3.62099186847));
#43265=CARTESIAN_POINT('Ctrl Pts',(-6.868838791574,2.874251915073,-3.288763647513));
#43266=CARTESIAN_POINT('Ctrl Pts',(-9.339612930525,-0.7060269082529,2.91246117975));
#43267=CARTESIAN_POINT('Ctrl Pts',(-9.312529597191,-1.366843388254,2.432349903822));
#43268=CARTESIAN_POINT('Ctrl Pts',(-9.258362930525,-2.345987543538,1.006798171184));
#43269=CARTESIAN_POINT('Ctrl Pts',(-9.177112930525,-2.142776363079,-1.581827080662));
#43270=CARTESIAN_POINT('Ctrl Pts',(-9.095862930525,-0.3554888892263,-3.465001338974));
#43271=CARTESIAN_POINT('Ctrl Pts',(-9.014612930525,2.21853712561,-3.80390848591));
#43272=CARTESIAN_POINT('Ctrl Pts',(-8.933362930525,4.43223290845,-2.447352893234));
#43273=CARTESIAN_POINT('Ctrl Pts',(-8.852112930525,5.29888400806,-3.878288208359E-7));
#43274=CARTESIAN_POINT('Ctrl Pts',(-8.770862930525,4.432231059311,2.44735444455));
#43275=CARTESIAN_POINT('Ctrl Pts',(-8.689612930525,2.218544522168,3.803903056307));
#43276=CARTESIAN_POINT('Ctrl Pts',(-8.608362930525,-0.3555166263194,3.465021506074));
#43277=CARTESIAN_POINT('Ctrl Pts',(-8.527112930525,-2.142672811265,1.581751841867));
#43278=CARTESIAN_POINT('Ctrl Pts',(-8.445862930525,-2.346374013702,-1.006517383103));
#43279=CARTESIAN_POINT('Ctrl Pts',(-8.364612930525,-0.8758289817713,-3.146173683671));
#43280=CARTESIAN_POINT('Ctrl Pts',(-8.283362930525,1.61352849127,-3.883554960714));
#43281=CARTESIAN_POINT('Ctrl Pts',(-8.202112930525,4.01217167154,-2.890004424173));
#43282=CARTESIAN_POINT('Ctrl Pts',(-8.120862930525,5.25100591992,-0.6083555729063));
#43283=CARTESIAN_POINT('Ctrl Pts',(-8.039612930525,4.777872805634,1.944442270929));
#43284=CARTESIAN_POINT('Ctrl Pts',(-7.958362930525,2.803651579289,3.63058648919));
#43285=CARTESIAN_POINT('Ctrl Pts',(-7.877112930525,0.208268587387,3.698548984649));
#43286=CARTESIAN_POINT('Ctrl Pts',(-7.795862930525,-1.851493007336,2.11803832419));
#43287=CARTESIAN_POINT('Ctrl Pts',(-7.714612930525,-2.457580825662,-0.4064991250853));
#43288=CARTESIAN_POINT('Ctrl Pts',(-7.633362930525,-1.339856629968,-2.74985663043));
#43289=CARTESIAN_POINT('Ctrl Pts',(-7.552112930525,1.003500871907,-3.867580826823));
#43290=CARTESIAN_POINT('Ctrl Pts',(-7.470862930525,3.52803833576,-3.261493002233));
#43291=CARTESIAN_POINT('Ctrl Pts',(-7.389612930525,5.108548941379,-1.201731431865));
#43292=CARTESIAN_POINT('Ctrl Pts',(-7.308362930525,5.0405866507,1.393651651195));
#43293=CARTESIAN_POINT('Ctrl Pts',(-7.227112930525,3.35444166816,3.367872537265));
#43294=CARTESIAN_POINT('Ctrl Pts',(-7.145862930525,0.8016466766589,3.841006921488));
#43295=CARTESIAN_POINT('Ctrl Pts',(-7.064612930525,-1.480012819665,2.602167933636));
#43296=CARTESIAN_POINT('Ctrl Pts',(-6.983362930525,-2.473523628312,0.203542441318));
#43297=CARTESIAN_POINT('Ctrl Pts',(-6.902112930525,-1.736290617787,-2.28588104406));
#43298=CARTESIAN_POINT('Ctrl Pts',(-6.820862930525,0.4039190209595,-3.756179714594));
#43299=CARTESIAN_POINT('Ctrl Pts',(-6.766696263858,2.128055113476,-3.62099186847));
#43300=CARTESIAN_POINT('Ctrl Pts',(-6.739612930525,2.874251915073,-3.288763647513));
#43301=CARTESIAN_POINT('Ctrl Pts',(-9.210387069475,-0.7060269082529,2.91246117975));
#43302=CARTESIAN_POINT('Ctrl Pts',(-9.183303736142,-1.366843388254,2.432349903822));
#43303=CARTESIAN_POINT('Ctrl Pts',(-9.129137069475,-2.345987543538,1.006798171184));
#43304=CARTESIAN_POINT('Ctrl Pts',(-9.047887069475,-2.142776363079,-1.581827080662));
#43305=CARTESIAN_POINT('Ctrl Pts',(-8.966637069475,-0.3554888892263,-3.465001338974));
#43306=CARTESIAN_POINT('Ctrl Pts',(-8.885387069475,2.21853712561,-3.80390848591));
#43307=CARTESIAN_POINT('Ctrl Pts',(-8.804137069475,4.43223290845,-2.447352893234));
#43308=CARTESIAN_POINT('Ctrl Pts',(-8.722887069475,5.29888400806,-3.878288207249E-7));
#43309=CARTESIAN_POINT('Ctrl Pts',(-8.641637069475,4.432231059311,2.44735444455));
#43310=CARTESIAN_POINT('Ctrl Pts',(-8.560387069475,2.218544522168,3.803903056307));
#43311=CARTESIAN_POINT('Ctrl Pts',(-8.479137069475,-0.3555166263194,3.465021506074));
#43312=CARTESIAN_POINT('Ctrl Pts',(-8.397887069475,-2.142672811265,1.581751841867));
#43313=CARTESIAN_POINT('Ctrl Pts',(-8.316637069475,-2.346374013702,-1.006517383103));
#43314=CARTESIAN_POINT('Ctrl Pts',(-8.235387069475,-0.8758289817713,-3.146173683671));
#43315=CARTESIAN_POINT('Ctrl Pts',(-8.154137069475,1.61352849127,-3.883554960714));
#43316=CARTESIAN_POINT('Ctrl Pts',(-8.072887069475,4.01217167154,-2.890004424173));
#43317=CARTESIAN_POINT('Ctrl Pts',(-7.991637069475,5.25100591992,-0.6083555729063));
#43318=CARTESIAN_POINT('Ctrl Pts',(-7.910387069475,4.777872805634,1.944442270929));
#43319=CARTESIAN_POINT('Ctrl Pts',(-7.829137069475,2.803651579289,3.63058648919));
#43320=CARTESIAN_POINT('Ctrl Pts',(-7.747887069475,0.208268587387,3.698548984649));
#43321=CARTESIAN_POINT('Ctrl Pts',(-7.666637069475,-1.851493007336,2.11803832419));
#43322=CARTESIAN_POINT('Ctrl Pts',(-7.585387069475,-2.457580825662,-0.4064991250853));
#43323=CARTESIAN_POINT('Ctrl Pts',(-7.504137069475,-1.339856629968,-2.74985663043));
#43324=CARTESIAN_POINT('Ctrl Pts',(-7.422887069475,1.003500871907,-3.867580826823));
#43325=CARTESIAN_POINT('Ctrl Pts',(-7.341637069475,3.52803833576,-3.261493002233));
#43326=CARTESIAN_POINT('Ctrl Pts',(-7.260387069475,5.108548941379,-1.201731431865));
#43327=CARTESIAN_POINT('Ctrl Pts',(-7.179137069475,5.0405866507,1.393651651195));
#43328=CARTESIAN_POINT('Ctrl Pts',(-7.097887069475,3.35444166816,3.367872537265));
#43329=CARTESIAN_POINT('Ctrl Pts',(-7.016637069475,0.8016466766589,3.841006921488));
#43330=CARTESIAN_POINT('Ctrl Pts',(-6.935387069475,-1.480012819665,2.602167933636));
#43331=CARTESIAN_POINT('Ctrl Pts',(-6.854137069475,-2.473523628312,0.203542441318));
#43332=CARTESIAN_POINT('Ctrl Pts',(-6.772887069475,-1.736290617787,-2.28588104406));
#43333=CARTESIAN_POINT('Ctrl Pts',(-6.691637069475,0.4039190209595,-3.756179714594));
#43334=CARTESIAN_POINT('Ctrl Pts',(-6.637470402809,2.128055113476,-3.62099186847));
#43335=CARTESIAN_POINT('Ctrl Pts',(-6.610387069475,2.874251915073,-3.288763647513));
#43336=CARTESIAN_POINT('Ctrl Pts',(-9.081161208426,-0.7060269082529,2.91246117975));
#43337=CARTESIAN_POINT('Ctrl Pts',(-9.054077875092,-1.366843388254,2.432349903822));
#43338=CARTESIAN_POINT('Ctrl Pts',(-8.999911208426,-2.345987543538,1.006798171184));
#43339=CARTESIAN_POINT('Ctrl Pts',(-8.918661208426,-2.142776363079,-1.581827080662));
#43340=CARTESIAN_POINT('Ctrl Pts',(-8.837411208426,-0.3554888892263,-3.465001338974));
#43341=CARTESIAN_POINT('Ctrl Pts',(-8.756161208426,2.21853712561,-3.80390848591));
#43342=CARTESIAN_POINT('Ctrl Pts',(-8.674911208426,4.43223290845,-2.447352893234));
#43343=CARTESIAN_POINT('Ctrl Pts',(-8.593661208426,5.29888400806,-3.878288207249E-7));
#43344=CARTESIAN_POINT('Ctrl Pts',(-8.512411208426,4.432231059311,2.44735444455));
#43345=CARTESIAN_POINT('Ctrl Pts',(-8.431161208426,2.218544522168,3.803903056307));
#43346=CARTESIAN_POINT('Ctrl Pts',(-8.349911208426,-0.3555166263194,3.465021506074));
#43347=CARTESIAN_POINT('Ctrl Pts',(-8.268661208426,-2.142672811265,1.581751841867));
#43348=CARTESIAN_POINT('Ctrl Pts',(-8.187411208426,-2.346374013702,-1.006517383103));
#43349=CARTESIAN_POINT('Ctrl Pts',(-8.106161208426,-0.8758289817713,-3.146173683671));
#43350=CARTESIAN_POINT('Ctrl Pts',(-8.024911208426,1.61352849127,-3.883554960714));
#43351=CARTESIAN_POINT('Ctrl Pts',(-7.943661208426,4.01217167154,-2.890004424173));
#43352=CARTESIAN_POINT('Ctrl Pts',(-7.862411208426,5.25100591992,-0.6083555729063));
#43353=CARTESIAN_POINT('Ctrl Pts',(-7.781161208426,4.777872805634,1.944442270929));
#43354=CARTESIAN_POINT('Ctrl Pts',(-7.699911208426,2.803651579289,3.63058648919));
#43355=CARTESIAN_POINT('Ctrl Pts',(-7.618661208426,0.208268587387,3.698548984649));
#43356=CARTESIAN_POINT('Ctrl Pts',(-7.537411208426,-1.851493007336,2.11803832419));
#43357=CARTESIAN_POINT('Ctrl Pts',(-7.456161208426,-2.457580825662,-0.4064991250853));
#43358=CARTESIAN_POINT('Ctrl Pts',(-7.374911208426,-1.339856629968,-2.74985663043));
#43359=CARTESIAN_POINT('Ctrl Pts',(-7.293661208426,1.003500871907,-3.867580826823));
#43360=CARTESIAN_POINT('Ctrl Pts',(-7.212411208426,3.52803833576,-3.261493002233));
#43361=CARTESIAN_POINT('Ctrl Pts',(-7.131161208426,5.108548941379,-1.201731431865));
#43362=CARTESIAN_POINT('Ctrl Pts',(-7.049911208426,5.0405866507,1.393651651195));
#43363=CARTESIAN_POINT('Ctrl Pts',(-6.968661208426,3.35444166816,3.367872537265));
#43364=CARTESIAN_POINT('Ctrl Pts',(-6.887411208426,0.8016466766589,3.841006921488));
#43365=CARTESIAN_POINT('Ctrl Pts',(-6.806161208426,-1.480012819665,2.602167933636));
#43366=CARTESIAN_POINT('Ctrl Pts',(-6.724911208426,-2.473523628312,0.203542441318));
#43367=CARTESIAN_POINT('Ctrl Pts',(-6.643661208426,-1.736290617787,-2.28588104406));
#43368=CARTESIAN_POINT('Ctrl Pts',(-6.562411208426,0.4039190209595,-3.756179714594));
#43369=CARTESIAN_POINT('Ctrl Pts',(-6.508244541759,2.128055113476,-3.62099186847));
#43370=CARTESIAN_POINT('Ctrl Pts',(-6.481161208426,2.874251915073,-3.288763647513));
#43371=CARTESIAN_POINT('Origin',(-4.6,4.874101615138,2.));
#43372=CARTESIAN_POINT('Origin',(-3.1,0.,0.));
#43373=CARTESIAN_POINT('',(-3.1,1.41,-6.));
#43374=CARTESIAN_POINT('Origin',(-3.1,1.41,0.));
#43375=CARTESIAN_POINT('Origin',(5.25,1.41,0.));
#43376=CARTESIAN_POINT('',(4.25,1.41,-6.));
#43377=CARTESIAN_POINT('',(5.25,1.41,-6.));
#43378=CARTESIAN_POINT('Origin',(4.25,1.41,0.));
#43379=CARTESIAN_POINT('',(0.,5.68,-4.215103794689));
#43380=CARTESIAN_POINT('',(1.63085988542761E-16,5.68,4.21510379468881));
#43381=CARTESIAN_POINT('Ctrl Pts',(0.,5.68,-4.21510379468881));
#43382=CARTESIAN_POINT('Ctrl Pts',(-0.266706680138663,5.68,-4.21510379468881));
#43383=CARTESIAN_POINT('Ctrl Pts',(-0.552196963605974,5.71567698479767,
-4.17989549259779));
#43384=CARTESIAN_POINT('Ctrl Pts',(-1.08458290107335,5.85511893191279,-4.03129022106372));
#43385=CARTESIAN_POINT('Ctrl Pts',(-1.33144862194443,5.95819559552318,-3.9171419061609));
#43386=CARTESIAN_POINT('Ctrl Pts',(-1.81218560208282,6.21764548689165,-3.59767135677579));
#43387=CARTESIAN_POINT('Ctrl Pts',(-2.03213201249546,6.38798517315582,-3.36454771509492));
#43388=CARTESIAN_POINT('Ctrl Pts',(-2.38147333747754,6.71484535620929,-2.82119365553778));
#43389=CARTESIAN_POINT('Ctrl Pts',(-2.51052533147875,6.871296113951,-2.51070089780968));
#43390=CARTESIAN_POINT('Ctrl Pts',(-2.79703133737243,7.26257643241256,-1.50498437334144));
#43391=CARTESIAN_POINT('Ctrl Pts',(-2.86057686489981,7.41,-0.73226230454066));
#43392=CARTESIAN_POINT('Ctrl Pts',(-2.86057686489981,7.41,0.));
#43393=CARTESIAN_POINT('Ctrl Pts',(-2.86057686489981,7.41,0.732262304540659));
#43394=CARTESIAN_POINT('Ctrl Pts',(-2.79703133737243,7.26257643241256,1.50498437334144));
#43395=CARTESIAN_POINT('Ctrl Pts',(-2.51052533147875,6.871296113951,2.51070089780968));
#43396=CARTESIAN_POINT('Ctrl Pts',(-2.38147333747754,6.71484535620929,2.82119365553778));
#43397=CARTESIAN_POINT('Ctrl Pts',(-2.03213201249546,6.38798517315582,3.36454771509492));
#43398=CARTESIAN_POINT('Ctrl Pts',(-1.81218560208282,6.21764548689165,3.59767135677579));
#43399=CARTESIAN_POINT('Ctrl Pts',(-1.33144862194443,5.95819559552318,3.9171419061609));
#43400=CARTESIAN_POINT('Ctrl Pts',(-1.08458290107335,5.85511893191279,4.03129022106372));
#43401=CARTESIAN_POINT('Ctrl Pts',(-0.552196963605975,5.71567698479767,
4.17989549259779));
#43402=CARTESIAN_POINT('Ctrl Pts',(-0.266706680138664,5.68,4.21510379468881));
#43403=CARTESIAN_POINT('Ctrl Pts',(-1.38777878078145E-16,5.68,4.21510379468881));
#43404=CARTESIAN_POINT('Ctrl Pts',(-6.93889390390723E-17,5.68,4.21510379468881));
#43405=CARTESIAN_POINT('Ctrl Pts',(0.266706680138664,5.68,4.21510379468881));
#43406=CARTESIAN_POINT('Ctrl Pts',(0.552196963605975,5.71567698479767,4.17989549259779));
#43407=CARTESIAN_POINT('Ctrl Pts',(1.08458290107335,5.85511893191279,4.03129022106372));
#43408=CARTESIAN_POINT('Ctrl Pts',(1.33144862194444,5.95819559552317,3.9171419061609));
#43409=CARTESIAN_POINT('Ctrl Pts',(1.81218560208282,6.21764548689165,3.59767135677579));
#43410=CARTESIAN_POINT('Ctrl Pts',(2.03213201249546,6.38798517315582,3.36454771509492));
#43411=CARTESIAN_POINT('Ctrl Pts',(2.38147333747754,6.71484535620929,2.82119365553778));
#43412=CARTESIAN_POINT('Ctrl Pts',(2.51052533147875,6.871296113951,2.51070089780968));
#43413=CARTESIAN_POINT('Ctrl Pts',(2.79703133737243,7.26257643241256,1.50498437334144));
#43414=CARTESIAN_POINT('Ctrl Pts',(2.86057686489981,7.41,0.73226230454066));
#43415=CARTESIAN_POINT('Ctrl Pts',(2.86057686489981,7.41,-0.73226230454066));
#43416=CARTESIAN_POINT('Ctrl Pts',(2.79703133737243,7.26257643241256,-1.50498437334144));
#43417=CARTESIAN_POINT('Ctrl Pts',(2.51052533147875,6.871296113951,-2.51070089780968));
#43418=CARTESIAN_POINT('Ctrl Pts',(2.38147333747754,6.71484535620929,-2.82119365553778));
#43419=CARTESIAN_POINT('Ctrl Pts',(2.03213201249546,6.38798517315582,-3.36454771509492));
#43420=CARTESIAN_POINT('Ctrl Pts',(1.81218560208282,6.21764548689165,-3.59767135677579));
#43421=CARTESIAN_POINT('Ctrl Pts',(1.33144862194444,5.95819559552317,-3.9171419061609));
#43422=CARTESIAN_POINT('Ctrl Pts',(1.08458290107335,5.85511893191279,-4.03129022106372));
#43423=CARTESIAN_POINT('Ctrl Pts',(0.552196963605975,5.71567698479767,-4.17989549259779));
#43424=CARTESIAN_POINT('Ctrl Pts',(0.266706680138664,5.68,-4.21510379468881));
#43425=CARTESIAN_POINT('Ctrl Pts',(0.,5.68,-4.21510379468881));
#43426=CARTESIAN_POINT('Origin',(4.25,0.,0.));
#43427=CARTESIAN_POINT('',(4.25,1.41,-6.75));
#43428=CARTESIAN_POINT('Origin',(4.25,1.41,0.));
#43429=CARTESIAN_POINT('Origin',(5.25,1.41,0.));
#43430=CARTESIAN_POINT('',(5.25,1.41,-6.75));
#43431=CARTESIAN_POINT('',(5.25,1.41,-6.75));
#43432=CARTESIAN_POINT('Origin',(5.25,1.41,0.));
#43433=CARTESIAN_POINT('Origin',(5.25,0.,0.));
#43434=CARTESIAN_POINT('',(5.24999993301406,7.94670116372702,-7.968642341825));
#43435=CARTESIAN_POINT('',(5.25000007836621,3.63834712397532,-7.50000017632907));
#43436=CARTESIAN_POINT('Ctrl Pts',(5.24999986926046,7.94670116372703,-7.96864234182499));
#43437=CARTESIAN_POINT('Ctrl Pts',(5.24999985979781,7.92042912898641,-7.98057901186823));
#43438=CARTESIAN_POINT('Ctrl Pts',(5.2500000454706,7.89428766094108,-7.99255496414018));
#43439=CARTESIAN_POINT('Ctrl Pts',(5.25000000000006,7.86827447145648,-8.00454117392044));
#43440=CARTESIAN_POINT('Ctrl Pts',(5.24999995731924,7.84385724015657,-8.01579200714822));
#43441=CARTESIAN_POINT('Ctrl Pts',(5.24999970997981,7.81955306918205,-8.0270518445332));
#43442=CARTESIAN_POINT('Ctrl Pts',(5.24999970836727,7.79536070220373,-8.03829312390875));
#43443=CARTESIAN_POINT('Ctrl Pts',(5.24999970656126,7.7682658959929,-8.05088305719287));
#43444=CARTESIAN_POINT('Ctrl Pts',(5.25000003233846,7.74131186309921,-8.06344951879706));
#43445=CARTESIAN_POINT('Ctrl Pts',(5.24999999999984,7.71444580188881,-8.07597690415732));
#43446=CARTESIAN_POINT('Ctrl Pts',(5.24999997270226,7.69176770109085,-8.08655148394815));
#43447=CARTESIAN_POINT('Ctrl Pts',(5.24999969135857,7.66915232604687,-8.09709825967747));
#43448=CARTESIAN_POINT('Ctrl Pts',(5.24999967895586,7.64656997550749,-8.1076038634778));
#43449=CARTESIAN_POINT('Ctrl Pts',(5.24999966354061,7.61850250221676,-8.12066121787298));
#43450=CARTESIAN_POINT('Ctrl Pts',(5.25000012887595,7.59048603449503,-8.13365525534816));
#43451=CARTESIAN_POINT('Ctrl Pts',(5.24999999999693,7.56249376377644,-8.14653794192863));
#43452=CARTESIAN_POINT('Ctrl Pts',(5.24999990234171,7.54128324084016,-8.15629951225435));
#43453=CARTESIAN_POINT('Ctrl Pts',(5.24999945605478,7.52008655804911,-8.16599720495859));
#43454=CARTESIAN_POINT('Ctrl Pts',(5.24999939312249,7.49889424963558,-8.17560645841391));
#43455=CARTESIAN_POINT('Ctrl Pts',(5.24999930603519,7.46956779655631,-8.18890398670037));
#43456=CARTESIAN_POINT('Ctrl Pts',(5.2500001189999,7.44024985607557,-8.20203300835797));
#43457=CARTESIAN_POINT('Ctrl Pts',(5.25000000000006,7.41093053450868,-8.21490731595539));
#43458=CARTESIAN_POINT('Ctrl Pts',(5.249999919518,7.39110126998961,-8.22361447687202));
#43459=CARTESIAN_POINT('Ctrl Pts',(5.24999935941906,7.37127128205611,-8.2322052130014));
#43460=CARTESIAN_POINT('Ctrl Pts',(5.24999921825673,7.35144050969113,-8.24065001429036));
#43461=CARTESIAN_POINT('Ctrl Pts',(5.24999899999811,7.32077909392119,-8.25370697236793));
#43462=CARTESIAN_POINT('Ctrl Pts',(5.25000009769284,7.29011544054891,-8.2664142201975));
#43463=CARTESIAN_POINT('Ctrl Pts',(5.24999999999859,7.25926186112955,-8.27871443681296));
#43464=CARTESIAN_POINT('Ctrl Pts',(5.24999994108235,7.24065506580565,-8.28613229941791));
#43465=CARTESIAN_POINT('Ctrl Pts',(5.24999934539331,7.22197913505664,-8.29340201010748));
#43466=CARTESIAN_POINT('Ctrl Pts',(5.24999915223788,7.20319642441607,-8.30050607557604));
#43467=CARTESIAN_POINT('Ctrl Pts',(5.24999884945851,7.17375372543655,-8.311642000796));
#43468=CARTESIAN_POINT('Ctrl Pts',(5.24999986612592,7.14404673713778,-8.32236961302399));
#43469=CARTESIAN_POINT('Ctrl Pts',(5.25000000790818,7.11368476804691,-8.33262088189463));
#43470=CARTESIAN_POINT('Ctrl Pts',(5.25000002226541,7.11061023868215,-8.33365895116722));
#43471=CARTESIAN_POINT('Ctrl Pts',(5.25000002173508,7.10752899840853,-8.33469209178922));
#43472=CARTESIAN_POINT('Ctrl Pts',(5.24999999999137,7.10444064568076,-8.33572020146925));
#43473=CARTESIAN_POINT('Ctrl Pts',(5.24999987233545,7.08630912824145,-8.34175616634638));
#43474=CARTESIAN_POINT('Ctrl Pts',(5.24999909769908,7.06793226520206,-8.34761949565941));
#43475=CARTESIAN_POINT('Ctrl Pts',(5.24999869097741,7.04923006893192,-8.35328916894757));
#43476=CARTESIAN_POINT('Ctrl Pts',(5.2499981544592,7.02455946657296,-8.36076819724869));
#43477=CARTESIAN_POINT('Ctrl Pts',(5.24999833662105,6.9993222943843,-8.36790723392353));
#43478=CARTESIAN_POINT('Ctrl Pts',(5.24999902610826,6.97331790178632,-8.37455580386236));
#43479=CARTESIAN_POINT('Ctrl Pts',(5.2499993431706,6.96135971981733,-8.37761316460872));
#43480=CARTESIAN_POINT('Ctrl Pts',(5.2499997293887,6.94923965184436,-8.38056625895871));
#43481=CARTESIAN_POINT('Ctrl Pts',(5.24999999992171,6.93694040179796,-8.38339734176588));
#43482=CARTESIAN_POINT('Ctrl Pts',(5.25000041319619,6.91815169250354,-8.38772219016327));
#43483=CARTESIAN_POINT('Ctrl Pts',(5.25000053414591,6.89894432415434,-8.39176277132838));
#43484=CARTESIAN_POINT('Ctrl Pts',(5.25000026927922,6.87924414025345,-8.39546034664865));
#43485=CARTESIAN_POINT('Ctrl Pts',(5.24999994432396,6.85507470427821,-8.39999676673572));
#43486=CARTESIAN_POINT('Ctrl Pts',(5.24999885106252,6.83018347199435,-8.4040151695677));
#43487=CARTESIAN_POINT('Ctrl Pts',(5.24999821940173,6.80454227883525,-8.40730778596991));
#43488=CARTESIAN_POINT('Ctrl Pts',(5.24999773730235,6.78497227616416,-8.40982079351158));
#43489=CARTESIAN_POINT('Ctrl Pts',(5.24999748527141,6.76496617478289,-8.41191057336018));
#43490=CARTESIAN_POINT('Ctrl Pts',(5.24999999607386,6.74453137954786,-8.41347976073673));
#43491=CARTESIAN_POINT('Ctrl Pts',(5.25000244927413,6.72456539410548,-8.4150129482219));
#43492=CARTESIAN_POINT('Ctrl Pts',(5.25000757949653,6.70419049199182,-8.41604885591512));
#43493=CARTESIAN_POINT('Ctrl Pts',(5.25001115564682,6.68341009717958,-8.41649761277241));
#43494=CARTESIAN_POINT('Ctrl Pts',(5.25001634209877,6.65327251609463,-8.41714843997256));
#43495=CARTESIAN_POINT('Ctrl Pts',(5.25001736124167,6.62227681778639,-8.41658575378721));
#43496=CARTESIAN_POINT('Ctrl Pts',(5.25001258721293,6.59061762597165,-8.41468583292122));
#43497=CARTESIAN_POINT('Ctrl Pts',(5.25000925802606,6.56853996969574,-8.4133609159721));
#43498=CARTESIAN_POINT('Ctrl Pts',(5.25000338360853,6.54614003683157,-8.41138640934763));
#43499=CARTESIAN_POINT('Ctrl Pts',(5.24999999458578,6.52347485149968,-8.40873179385859));
#43500=CARTESIAN_POINT('Ctrl Pts',(5.24999696928664,6.50324218541125,-8.40636208242688));
#43501=CARTESIAN_POINT('Ctrl Pts',(5.24999616463599,6.48279758957839,-8.40345058898327));
#43502=CARTESIAN_POINT('Ctrl Pts',(5.24999607720379,6.46220567247638,-8.39999184752192));
#43503=CARTESIAN_POINT('Ctrl Pts',(5.24999595356056,6.43308537815003,-8.39510062885324));
#43504=CARTESIAN_POINT('Ctrl Pts',(5.24999734419153,6.40362599126612,-8.38909780036147));
#43505=CARTESIAN_POINT('Ctrl Pts',(5.2499986539087,6.37396006149583,-8.38210528187685));
#43506=CARTESIAN_POINT('Ctrl Pts',(5.24999989231947,6.34590926717141,-8.37549346490901));
#43507=CARTESIAN_POINT('Ctrl Pts',(5.25000136507078,6.31767342551847,-8.36799762707938));
#43508=CARTESIAN_POINT('Ctrl Pts',(5.25000022613449,6.28931191598885,-8.35972094746712));
#43509=CARTESIAN_POINT('Ctrl Pts',(5.25000016055573,6.28767888988593,-8.35924438489776));
#43510=CARTESIAN_POINT('Ctrl Pts',(5.25000008515903,6.28604543293954,-8.35876523173905));
#43511=CARTESIAN_POINT('Ctrl Pts',(5.24999999892296,6.28441155129405,-8.35828350689833));
#43512=CARTESIAN_POINT('Ctrl Pts',(5.24999899277608,6.26534847426058,-8.35266305221421));
#43513=CARTESIAN_POINT('Ctrl Pts',(5.24999656259104,6.24622792118924,-8.34669240771587));
#43514=CARTESIAN_POINT('Ctrl Pts',(5.2499944902779,6.22707173109384,-8.34041729961635));
#43515=CARTESIAN_POINT('Ctrl Pts',(5.24998960195341,6.18188470255591,-8.32561511362009));
#43516=CARTESIAN_POINT('Ctrl Pts',(5.249989597612,6.13651203359492,-8.30906928328382));
#43517=CARTESIAN_POINT('Ctrl Pts',(5.24999486284137,6.09091967408837,-8.29121673089798));
#43518=CARTESIAN_POINT('Ctrl Pts',(5.24999686514397,6.07358145499244,-8.28442762263429));
#43519=CARTESIAN_POINT('Ctrl Pts',(5.24999919861929,6.05621110809025,-8.27744938914288));
#43520=CARTESIAN_POINT('Ctrl Pts',(5.24999999958938,6.03880643800309,-8.2703055376079));
#43521=CARTESIAN_POINT('Ctrl Pts',(5.25000079658244,6.0214881870133,-8.26319715731128));
#43522=CARTESIAN_POINT('Ctrl Pts',(5.25000001560539,6.00413601494501,-8.25592473803094));
#43523=CARTESIAN_POINT('Ctrl Pts',(5.24999898541405,5.98674097435617,-8.24850965134291));
#43524=CARTESIAN_POINT('Ctrl Pts',(5.2499964517624,5.94395962734543,-8.23027299388325));
#43525=CARTESIAN_POINT('Ctrl Pts',(5.24999411548082,5.90094906844815,-8.21118434813899));
#43526=CARTESIAN_POINT('Ctrl Pts',(5.24999628257442,5.85773628457346,-8.19153407956133));
#43527=CARTESIAN_POINT('Ctrl Pts',(5.24999744061961,5.83464436243185,-8.18103342601924));
#43528=CARTESIAN_POINT('Ctrl Pts',(5.24999948052378,5.81149511755054,-8.1703729347153));
#43529=CARTESIAN_POINT('Ctrl Pts',(5.2499999999919,5.78829678611397,-8.15960055110763));
#43530=CARTESIAN_POINT('Ctrl Pts',(5.25000034546962,5.77286849277986,-8.15243626454413));
#43531=CARTESIAN_POINT('Ctrl Pts',(5.24999995290227,5.75741859124791,-8.14522255069958));
#43532=CARTESIAN_POINT('Ctrl Pts',(5.24999940442921,5.74194736020579,-8.13797052346545));
#43533=CARTESIAN_POINT('Ctrl Pts',(5.24999775717843,5.69548200164799,-8.11619022396715));
#43534=CARTESIAN_POINT('Ctrl Pts',(5.24999615656465,5.64883593126901,-8.09407626703666));
#43535=CARTESIAN_POINT('Ctrl Pts',(5.24999770219945,5.60220799517453,-8.07196864924727));
#43536=CARTESIAN_POINT('Ctrl Pts',(5.24999845313466,5.57955415791413,-8.06122782695136));
#43537=CARTESIAN_POINT('Ctrl Pts',(5.24999964840422,5.55690524771809,-8.05048886902695));
#43538=CARTESIAN_POINT('Ctrl Pts',(5.24999999999646,5.5342879683987,-8.03979216915111));
#43539=CARTESIAN_POINT('Ctrl Pts',(5.25000020599498,5.52103646411359,-8.03352495361915));
#43540=CARTESIAN_POINT('Ctrl Pts',(5.25000009968989,5.50779587343064,-8.02727225737731));
#43541=CARTESIAN_POINT('Ctrl Pts',(5.24999989787751,5.49457103649227,-8.02104089797295));
#43542=CARTESIAN_POINT('Ctrl Pts',(5.24999902774336,5.43755083513988,-7.99417377139956));
#43543=CARTESIAN_POINT('Ctrl Pts',(5.24999833607258,5.38082137601284,-7.96771614392102));
#43544=CARTESIAN_POINT('Ctrl Pts',(5.24999941548658,5.32413575082117,-7.94183310567151));
#43545=CARTESIAN_POINT('Ctrl Pts',(5.24999968327137,5.31007298348315,-7.93541195138993));
#43546=CARTESIAN_POINT('Ctrl Pts',(5.24999994395975,5.29601313071909,-7.92902622523739));
#43547=CARTESIAN_POINT('Ctrl Pts',(5.24999999998534,5.28195281698071,-7.92267859721573));
#43548=CARTESIAN_POINT('Ctrl Pts',(5.25000004390683,5.27093017428062,-7.9177023472559));
#43549=CARTESIAN_POINT('Ctrl Pts',(5.24999995980601,5.25990725211983,-7.91274951373632));
#43550=CARTESIAN_POINT('Ctrl Pts',(5.24999982929753,5.24888230738315,-7.90782095774229));
#43551=CARTESIAN_POINT('Ctrl Pts',(5.2499993030909,5.20443003061332,-7.887949154268));
#43552=CARTESIAN_POINT('Ctrl Pts',(5.24999849170788,5.15993871607658,-7.86848537238923));
#43553=CARTESIAN_POINT('Ctrl Pts',(5.24999892117554,5.11486500000911,-7.84930144838585));
#43554=CARTESIAN_POINT('Ctrl Pts',(5.24999919587201,5.08603491199674,-7.83703101085165));
#43555=CARTESIAN_POINT('Ctrl Pts',(5.24999986607924,5.05696627771669,-7.8248756934888));
#43556=CARTESIAN_POINT('Ctrl Pts',(5.24999999999432,5.02751255560357,-7.81281258125108));
#43557=CARTESIAN_POINT('Ctrl Pts',(5.25000004186963,5.01830236391083,-7.80904044081688));
#43558=CARTESIAN_POINT('Ctrl Pts',(5.2500000224096,5.00905448794408,-7.80527739227639));
#43559=CARTESIAN_POINT('Ctrl Pts',(5.24999997176832,4.99976434331729,-7.80152284206514));
#43560=CARTESIAN_POINT('Ctrl Pts',(5.24999975764146,4.9604827571553,-7.78564745007203));
#43561=CARTESIAN_POINT('Ctrl Pts',(5.2499991504668,4.92044535873102,-7.76992996410811));
#43562=CARTESIAN_POINT('Ctrl Pts',(5.24999920773422,4.87931378761042,-7.75436286495623));
#43563=CARTESIAN_POINT('Ctrl Pts',(5.24999926490981,4.83824817735725,-7.73882073006745));
#43564=CARTESIAN_POINT('Ctrl Pts',(5.25000006250811,4.79609208646318,-7.72342743327411));
#43565=CARTESIAN_POINT('Ctrl Pts',(5.249999999991,4.75249331950356,-7.7082247363706));
#43566=CARTESIAN_POINT('Ctrl Pts',(5.24999998891567,4.74476950044821,-7.70553147488123));
#43567=CARTESIAN_POINT('Ctrl Pts',(5.24999994182541,4.73700036006587,-7.70284434575642));
#43568=CARTESIAN_POINT('Ctrl Pts',(5.24999987261493,4.72918391457014,-7.7001637385431));
#43569=CARTESIAN_POINT('Ctrl Pts',(5.24999946999015,4.68371255323638,-7.68456958398051));
#43570=CARTESIAN_POINT('Ctrl Pts',(5.24999850571767,4.63664612843812,-7.66919091579023));
#43571=CARTESIAN_POINT('Ctrl Pts',(5.2499985244879,4.58787344246801,-7.65423058086207));
#43572=CARTESIAN_POINT('Ctrl Pts',(5.24999854325813,4.53910075649789,-7.63927024593392));
#43573=CARTESIAN_POINT('Ctrl Pts',(5.24999969153135,4.48862171261842,-7.62472744726044));
#43574=CARTESIAN_POINT('Ctrl Pts',(5.24999999999003,4.43632478576696,-7.61086130246294));
#43575=CARTESIAN_POINT('Ctrl Pts',(5.25000003518208,4.43035823099177,-7.60927931442968));
#43576=CARTESIAN_POINT('Ctrl Pts',(5.25000005411519,4.42436801418822,-7.60770620227508));
#43577=CARTESIAN_POINT('Ctrl Pts',(5.25000006066451,4.41835398312687,-7.60614239344774));
#43578=CARTESIAN_POINT('Ctrl Pts',(5.25000010971638,4.37331122899801,-7.59443007340888));
#43579=CARTESIAN_POINT('Ctrl Pts',(5.24999955774809,4.32693296153263,-7.5832489428317));
#43580=CARTESIAN_POINT('Ctrl Pts',(5.24999945792033,4.27908779984327,-7.57278693404784));
#43581=CARTESIAN_POINT('Ctrl Pts',(5.24999936403813,4.23409220879664,-7.56294802344239));
#43582=CARTESIAN_POINT('Ctrl Pts',(5.24999971534387,4.18779916246661,-7.55374493379632));
#43583=CARTESIAN_POINT('Ctrl Pts',(5.24999998994999,4.14010088266014,-7.54537978049226));
#43584=CARTESIAN_POINT('Ctrl Pts',(5.2500001263197,4.11641386353316,-7.54122563600073));
#43585=CARTESIAN_POINT('Ctrl Pts',(5.25000021765403,4.09238032773424,-7.53727888386729));
#43586=CARTESIAN_POINT('Ctrl Pts',(5.2499999999999,4.06798733192949,-7.53356914073385));
#43587=CARTESIAN_POINT('Ctrl Pts',(5.24999996894701,4.06450716288216,-7.53303986858828));
#43588=CARTESIAN_POINT('Ctrl Pts',(5.24999993132666,4.06101967736794,-7.53251542663155));
#43589=CARTESIAN_POINT('Ctrl Pts',(5.24999988805877,4.05752485198541,-7.53199590138679));
#43590=CARTESIAN_POINT('Ctrl Pts',(5.24999929308391,4.00946766391712,-7.5248519329017));
#43591=CARTESIAN_POINT('Ctrl Pts',(5.24999772967613,3.96003396915788,-7.51863731311267));
#43592=CARTESIAN_POINT('Ctrl Pts',(5.24999701437125,3.9092284710242,-7.51362111328977));
#43593=CARTESIAN_POINT('Ctrl Pts',(5.24999633485654,3.86096501835613,-7.50885589827132));
#43594=CARTESIAN_POINT('Ctrl Pts',(5.24999647268159,3.81146348065842,-7.50517209025358));
#43595=CARTESIAN_POINT('Ctrl Pts',(5.24999744301681,3.76075092647382,-7.50284022076318));
#43596=CARTESIAN_POINT('Ctrl Pts',(5.2499982094219,3.72069635688742,-7.50099842773439));
#43597=CARTESIAN_POINT('Ctrl Pts',(5.24999948018792,3.67988668822894,-7.50000070445283));
#43598=CARTESIAN_POINT('Ctrl Pts',(5.25000017632343,3.63834712397696,-7.50000017632941));
#43599=CARTESIAN_POINT('',(5.25,10.41979065301,-7.968642341825));
#43600=CARTESIAN_POINT('',(5.25,10.41979065301,-7.968642341825));
#43601=CARTESIAN_POINT('',(5.24999999999988,10.4571163879047,-7.96641903838753));
#43602=CARTESIAN_POINT('Ctrl Pts',(5.24999999999953,10.45711625936,-7.966419053641));
#43603=CARTESIAN_POINT('Ctrl Pts',(5.24999999999953,10.45297744471,-7.96691054287));
#43604=CARTESIAN_POINT('Ctrl Pts',(5.24999999999955,10.448836167275,-7.9673236221365));
#43605=CARTESIAN_POINT('Ctrl Pts',(5.24999999999956,10.4446918747092,-7.96765338841725));
#43606=CARTESIAN_POINT('Ctrl Pts',(5.24999999999957,10.4405475821433,-7.967983154698));
#43607=CARTESIAN_POINT('Ctrl Pts',(5.24999999999957,10.4364002744467,-7.968229607993));
#43608=CARTESIAN_POINT('Ctrl Pts',(5.24999999999958,10.4322500589158,-7.9683944361125));
#43609=CARTESIAN_POINT('Ctrl Pts',(5.24999999999958,10.428099843385,-7.96855926423199));
#43610=CARTESIAN_POINT('Ctrl Pts',(5.24999999999958,10.42394672002,-7.968642467176));
#43611=CARTESIAN_POINT('Ctrl Pts',(5.24999999999958,10.41979065301,-7.968642341825));
#43612=CARTESIAN_POINT('',(5.24999999999997,12.1609694417917,-7.72257626142715));
#43613=CARTESIAN_POINT('Ctrl Pts',(5.25,12.1609694417906,-7.72257626142175));
#43614=CARTESIAN_POINT('Ctrl Pts',(5.25,12.0834979181545,-7.73841082136219));
#43615=CARTESIAN_POINT('Ctrl Pts',(5.25,11.9234509679755,-7.76813457545424));
#43616=CARTESIAN_POINT('Ctrl Pts',(5.25,11.67408343811,-7.808462753035));
#43617=CARTESIAN_POINT('Ctrl Pts',(5.25,11.39910660014,-7.848332324994));
#43618=CARTESIAN_POINT('Ctrl Pts',(5.25,11.09804785384,-7.888268548859));
#43619=CARTESIAN_POINT('Ctrl Pts',(5.25,10.7798535275883,-7.9278253552661));
#43620=CARTESIAN_POINT('Ctrl Pts',(5.25,10.5655600593217,-7.95355186396394));
#43621=CARTESIAN_POINT('Ctrl Pts',(5.25,10.4571163879049,-7.96641903838876));
#43622=CARTESIAN_POINT('',(5.25,12.4099999863643,-7.6583523942248));
#43623=CARTESIAN_POINT('Ctrl Pts',(5.25,12.4099999860592,-7.65835239311871));
#43624=CARTESIAN_POINT('Ctrl Pts',(5.25,12.3926880098894,-7.66312722015755));
#43625=CARTESIAN_POINT('Ctrl Pts',(5.25,12.3587824122134,-7.6725047316683));
#43626=CARTESIAN_POINT('Ctrl Pts',(5.25,12.31026017487,-7.68580697919));
#43627=CARTESIAN_POINT('Ctrl Pts',(5.25,12.26332802492,-7.698354350369));
#43628=CARTESIAN_POINT('Ctrl Pts',(5.25,12.21488327627,-7.710652709337));
#43629=CARTESIAN_POINT('Ctrl Pts',(5.25,12.1793923623,-7.718809498598));
#43630=CARTESIAN_POINT('Ctrl Pts',(5.25,12.16096980378,-7.722576187434));
#43631=CARTESIAN_POINT('',(5.25,12.40999999936,7.5));
#43632=CARTESIAN_POINT('',(5.25,12.40999999936,7.5));
#43633=CARTESIAN_POINT('',(5.25,1.41,7.5));
#43634=CARTESIAN_POINT('',(5.25,1.41,7.5));
#43635=CARTESIAN_POINT('',(5.25,0.04746907580983,7.375195555416));
#43636=CARTESIAN_POINT('Origin',(5.25,1.41,0.));
#43637=CARTESIAN_POINT('',(5.25,-0.975037109157,7.551196560962));
#43638=CARTESIAN_POINT('Origin',(5.25,-0.2250371090282,8.850234666499));
#43639=CARTESIAN_POINT('',(5.25,-5.118174593052,9.943238102513));
#43640=CARTESIAN_POINT('',(5.25,-5.118174593052,9.943238102513));
#43641=CARTESIAN_POINT('',(5.25,-8.533238102513,6.528174593052));
#43642=CARTESIAN_POINT('Origin',(5.25,-6.368174593052,7.778174593052));
#43643=CARTESIAN_POINT('',(5.25,-6.141196560822,2.385037109028));
#43644=CARTESIAN_POINT('',(5.25,-6.141196560967,2.385037109161));
#43645=CARTESIAN_POINT('',(5.25,-5.965195555416,1.36253092419));
#43646=CARTESIAN_POINT('Origin',(5.25,-7.440234666499,1.635037109028));
#43647=CARTESIAN_POINT('',(5.25,1.41,-7.5));
#43648=CARTESIAN_POINT('Origin',(5.25,1.41,0.));
#43649=CARTESIAN_POINT('',(5.250000058775,3.638347091316,-7.500000176329));
#43650=CARTESIAN_POINT('',(5.25,-6.368174593052,9.028174593052));
#43651=CARTESIAN_POINT('Origin',(5.25,-6.368174593052,7.778174593052));
#43652=CARTESIAN_POINT('Origin',(5.25,-6.368174593052,7.778174593052));
#43653=CARTESIAN_POINT('',(2.75,-6.368174593052,9.028174593052));
#43654=CARTESIAN_POINT('Origin',(2.75,-6.368174593052,7.778174593052));
#43655=CARTESIAN_POINT('',(5.25,-6.368174593052,9.028174593052));
#43656=CARTESIAN_POINT('Origin',(2.75,0.,0.));
#43657=CARTESIAN_POINT('',(2.75,-5.118174593052,9.943238102513));
#43658=CARTESIAN_POINT('',(2.75000000024287,-2.18603093399766,8.25036791856334));
#43659=CARTESIAN_POINT('',(2.75,-5.118174593052,9.943238102513));
#43660=CARTESIAN_POINT('',(2.74999999998423,-6.84036777526504,3.59603441391076));
#43661=CARTESIAN_POINT('Origin',(2.75,1.41,0.));
#43662=CARTESIAN_POINT('',(2.75,-8.533238102513,6.528174593052));
#43663=CARTESIAN_POINT('',(2.749999999978,-6.840370038804,3.596038711084));
#43664=CARTESIAN_POINT('Origin',(2.75,-6.368174593052,7.778174593052));
#43665=CARTESIAN_POINT('Origin',(3.25,-5.196644207287,9.988542555415));
#43666=CARTESIAN_POINT('',(3.25,-4.868174593052,10.37625080441));
#43667=CARTESIAN_POINT('Origin',(3.25,-5.118174593052,9.943238102513));
#43668=CARTESIAN_POINT('',(3.25,-0.7250371090282,7.984209262715));
#43669=CARTESIAN_POINT('',(3.25,-0.7250371090282,7.984209262715));
#43670=CARTESIAN_POINT('Ctrl Pts',(2.75000000080443,-2.18603081191096,8.25036913644901));
#43671=CARTESIAN_POINT('Ctrl Pts',(2.75000000143807,-2.18599696924301,8.2503657438976));
#43672=CARTESIAN_POINT('Ctrl Pts',(2.75000000265658,-2.18596312714159,8.25036235117153));
#43673=CARTESIAN_POINT('Ctrl Pts',(2.75000000445985,-2.18592928560675,8.25035895827084));
#43674=CARTESIAN_POINT('Ctrl Pts',(2.75000203206361,-2.14787778318541,8.24654397264854));
#43675=CARTESIAN_POINT('Ctrl Pts',(2.75074081561521,-2.11054605849314,8.24250971552603));
#43676=CARTESIAN_POINT('Ctrl Pts',(2.75208237772229,-2.07396390256443,8.23830837253815));
#43677=CARTESIAN_POINT('Ctrl Pts',(2.75351653681867,-2.03485678153477,8.23381704542679));
#43678=CARTESIAN_POINT('Ctrl Pts',(2.75563957979403,-1.99660590053698,8.22913468870886));
#43679=CARTESIAN_POINT('Ctrl Pts',(2.75832257441735,-1.9592033183985,8.22430523024947));
#43680=CARTESIAN_POINT('Ctrl Pts',(2.75919641252517,-1.94702148198355,8.22273229946338));
#43681=CARTESIAN_POINT('Ctrl Pts',(2.76012990642584,-1.93492932457007,8.22114362203655));
#43682=CARTESIAN_POINT('Ctrl Pts',(2.76111931513426,-1.92292575588343,8.21954032745987));
#43683=CARTESIAN_POINT('Ctrl Pts',(2.76180768008298,-1.91457446902568,8.21842486144499));
#43684=CARTESIAN_POINT('Ctrl Pts',(2.76252312304503,-1.90626632766312,8.21730248881821));
#43685=CARTESIAN_POINT('Ctrl Pts',(2.76326437045243,-1.89800218029635,8.2161738191947));
#43686=CARTESIAN_POINT('Ctrl Pts',(2.76730004426291,-1.85300856175418,8.21002885005913));
#43687=CARTESIAN_POINT('Ctrl Pts',(2.77209848480575,-1.80932259995566,8.20369889117441));
#43688=CARTESIAN_POINT('Ctrl Pts',(2.77749540077863,-1.76700707275716,8.19727271673768));
#43689=CARTESIAN_POINT('Ctrl Pts',(2.78100267390783,-1.73950764303895,8.19309656334957));
#43690=CARTESIAN_POINT('Ctrl Pts',(2.78476326022402,-1.71258601065174,8.188879337019));
#43691=CARTESIAN_POINT('Ctrl Pts',(2.78873776548973,-1.68625022687806,8.18464108598879));
#43692=CARTESIAN_POINT('Ctrl Pts',(2.79098335513103,-1.6713705477019,8.18224648037767));
#43693=CARTESIAN_POINT('Ctrl Pts',(2.79329729900393,-1.65667891831125,8.17984575545618));
#43694=CARTESIAN_POINT('Ctrl Pts',(2.79567328788736,-1.64217445308732,8.17744174943354));
#43695=CARTESIAN_POINT('Ctrl Pts',(2.80255749831722,-1.60014909199633,8.17047636190586));
#43696=CARTESIAN_POINT('Ctrl Pts',(2.80996108154947,-1.5596983374674,8.16348535455907));
#43697=CARTESIAN_POINT('Ctrl Pts',(2.81777158248429,-1.52080586459298,8.15653879339027));
#43698=CARTESIAN_POINT('Ctrl Pts',(2.82072673602345,-1.50609064596347,8.15391051704867));
#43699=CARTESIAN_POINT('Ctrl Pts',(2.82374036182381,-1.49159805648715,8.15128834736281));
#43700=CARTESIAN_POINT('Ctrl Pts',(2.8268071518979,-1.4773257415543,8.14867521058651));
#43701=CARTESIAN_POINT('Ctrl Pts',(2.83100504743873,-1.45778945580721,8.1450982865207));
#43702=CARTESIAN_POINT('Ctrl Pts',(2.83530229236517,-1.43866881913031,8.14153963541655));
#43703=CARTESIAN_POINT('Ctrl Pts',(2.83968716971298,-1.41995266321184,8.13800479351629));
#43704=CARTESIAN_POINT('Ctrl Pts',(2.84875078533761,-1.38126605244481,8.13069821553552));
#43705=CARTESIAN_POINT('Ctrl Pts',(2.85818770414255,-1.34431059448287,8.12349512669871));
#43706=CARTESIAN_POINT('Ctrl Pts',(2.86793215029481,-1.30901006276093,8.11644243981932));
#43707=CARTESIAN_POINT('Ctrl Pts',(2.8691616724745,-1.30455595772217,8.11555255497526));
#43708=CARTESIAN_POINT('Ctrl Pts',(2.87039611681958,-1.30012814775789,8.11466503148957));
#43709=CARTESIAN_POINT('Ctrl Pts',(2.87163537382243,-1.29572643767609,8.11377993626792));
#43710=CARTESIAN_POINT('Ctrl Pts',(2.87795924690619,-1.27326470790997,8.10926333492064));
#43711=CARTESIAN_POINT('Ctrl Pts',(2.884407574416,-1.25148815620034,8.10481226298927));
#43712=CARTESIAN_POINT('Ctrl Pts',(2.89096401354338,-1.2303795899674,8.1004364144946));
#43713=CARTESIAN_POINT('Ctrl Pts',(2.90080152733586,-1.1987075485709,8.09387073622263));
#43714=CARTESIAN_POINT('Ctrl Pts',(2.91088218359936,-1.16854172400716,8.08747545772209));
#43715=CARTESIAN_POINT('Ctrl Pts',(2.92117058635112,-1.13986277581381,8.08128868142044));
#43716=CARTESIAN_POINT('Ctrl Pts',(2.92974409568673,-1.1159640972722,8.07613313049));
#43717=CARTESIAN_POINT('Ctrl Pts',(2.93846080868979,-1.0931011345692,8.07112280556824));
#43718=CARTESIAN_POINT('Ctrl Pts',(2.94729604479062,-1.07126537440902,8.0662759237153));
#43719=CARTESIAN_POINT('Ctrl Pts',(2.95612955847588,-1.04943387109639,8.06142998675445));
#43720=CARTESIAN_POINT('Ctrl Pts',(2.96508155460103,-1.02862989400395,8.05674762477974));
#43721=CARTESIAN_POINT('Ctrl Pts',(2.97413022110453,-1.00887086876362,8.0522521809041));
#43722=CARTESIAN_POINT('Ctrl Pts',(2.98499562424733,-0.985144745708707,
8.04685416894336));
#43723=CARTESIAN_POINT('Ctrl Pts',(2.99599912932157,-0.962923457993005,
8.04172374290186));
#43724=CARTESIAN_POINT('Ctrl Pts',(3.0071077955465,-0.942199653336915,8.03688739802855));
#43725=CARTESIAN_POINT('Ctrl Pts',(3.0145034433413,-0.928402681036047,8.03366757824343));
#43726=CARTESIAN_POINT('Ctrl Pts',(3.02194572611609,-0.915268968712097,
8.03057785708498));
#43727=CARTESIAN_POINT('Ctrl Pts',(3.02942256884002,-0.902808977924984,
8.02762852891565));
#43728=CARTESIAN_POINT('Ctrl Pts',(3.04183447358211,-0.882124816916487,
8.02273250774167));
#43729=CARTESIAN_POINT('Ctrl Pts',(3.05434262452836,-0.863287067001056,
8.0182183319781));
#43730=CARTESIAN_POINT('Ctrl Pts',(3.06691280320266,-0.846284631151253,
8.01411257827712));
#43731=CARTESIAN_POINT('Ctrl Pts',(3.06760370501054,-0.845350116696736,
8.01388691142479));
#43732=CARTESIAN_POINT('Ctrl Pts',(3.06829479751297,-0.844421135571319,
8.01366247350665));
#43733=CARTESIAN_POINT('Ctrl Pts',(3.06898607616024,-0.843497682288813,
8.01343926730765));
#43734=CARTESIAN_POINT('Ctrl Pts',(3.07467411818084,-0.83589923975678,8.01160266170126));
#43735=CARTESIAN_POINT('Ctrl Pts',(3.0803746756442,-0.8286752304301,8.00984951854266));
#43736=CARTESIAN_POINT('Ctrl Pts',(3.08608187232844,-0.821827182093947,
8.00818252582984));
#43737=CARTESIAN_POINT('Ctrl Pts',(3.09708026754574,-0.808630240366617,
8.00497004767386));
#43738=CARTESIAN_POINT('Ctrl Pts',(3.10810885215689,-0.796817347737043,
8.00207175608596));
#43739=CARTESIAN_POINT('Ctrl Pts',(3.11909757641733,-0.786412036999781,
7.99950664885367));
#43740=CARTESIAN_POINT('Ctrl Pts',(3.12331828887664,-0.782415410673481,
7.99852140436139));
#43741=CARTESIAN_POINT('Ctrl Pts',(3.1275331906934,-0.778625917010289,7.99758515267624));
#43742=CARTESIAN_POINT('Ctrl Pts',(3.13173857046868,-0.77504297073421,7.99669838060771));
#43743=CARTESIAN_POINT('Ctrl Pts',(3.13551881815513,-0.771822233227817,
7.9959012544884));
#43744=CARTESIAN_POINT('Ctrl Pts',(3.13929136238273,-0.768768372415048,
7.99514410309805));
#43745=CARTESIAN_POINT('Ctrl Pts',(3.14305240612772,-0.765879628621723,
7.99442685358692));
#43746=CARTESIAN_POINT('Ctrl Pts',(3.15459054621756,-0.757017532663539,
7.99222647361269));
#43747=CARTESIAN_POINT('Ctrl Pts',(3.16602850201771,-0.749717434211676,
7.99040763809797));
#43748=CARTESIAN_POINT('Ctrl Pts',(3.1772685852345,-0.743883488159329,7.98894871026817));
#43749=CARTESIAN_POINT('Ctrl Pts',(3.18253941430561,-0.741147767092236,
7.98826457305409));
#43750=CARTESIAN_POINT('Ctrl Pts',(3.18776708152223,-0.73873377593749,7.98765940185426));
#43751=CARTESIAN_POINT('Ctrl Pts',(3.19294333485885,-0.736628319017608,
7.98713004868365));
#43752=CARTESIAN_POINT('Ctrl Pts',(3.1947510034279,-0.73589304428315,7.98694518619215));
#43753=CARTESIAN_POINT('Ctrl Pts',(3.19655241119166,-0.73519537838123,7.98676956462907));
#43754=CARTESIAN_POINT('Ctrl Pts',(3.19834710830016,-0.73453439781842,7.98660294139632));
#43755=CARTESIAN_POINT('Ctrl Pts',(3.20862886183901,-0.730747664553751,
7.98564836304162));
#43756=CARTESIAN_POINT('Ctrl Pts',(3.21869184518773,-0.728185401026915,
7.985002609133));
#43757=CARTESIAN_POINT('Ctrl Pts',(3.2285270849327,-0.726682175030561,7.98462380996472));
#43758=CARTESIAN_POINT('Ctrl Pts',(3.23580778908085,-0.725569386320671,
7.98434339741277));
#43759=CARTESIAN_POINT('Ctrl Pts',(3.24296430279622,-0.725037924549703,
7.98420952256945));
#43760=CARTESIAN_POINT('Ctrl Pts',(3.25,-0.725037109028451,7.98420926271457));
#43761=CARTESIAN_POINT('Ctrl Pts',(2.748031232229,-2.249001700534,8.299984818872));
#43762=CARTESIAN_POINT('Ctrl Pts',(2.748165300609,-2.234652803614,8.298726087963));
#43763=CARTESIAN_POINT('Ctrl Pts',(2.750023861624,-2.124930155855,8.288701163509));
#43764=CARTESIAN_POINT('Ctrl Pts',(2.764346989763,-1.927188444858,8.26530476129));
#43765=CARTESIAN_POINT('Ctrl Pts',(2.803313967766,-1.669542337486,8.224590429631));
#43766=CARTESIAN_POINT('Ctrl Pts',(2.852280936191,-1.44708336687,8.182172690363));
#43767=CARTESIAN_POINT('Ctrl Pts',(2.906900085727,-1.25819520666,8.141037625298));
#43768=CARTESIAN_POINT('Ctrl Pts',(2.964682486012,-1.101023410635,8.103166220994));
#43769=CARTESIAN_POINT('Ctrl Pts',(3.024021001282,-0.9744663407883,8.070107631206));
#43770=CARTESIAN_POINT('Ctrl Pts',(3.083563542553,-0.8781689679159,8.043241583061));
#43771=CARTESIAN_POINT('Ctrl Pts',(3.141847763167,-0.8121044008003,8.023815916094));
#43772=CARTESIAN_POINT('Ctrl Pts',(3.197244721767,-0.7752791571759,8.012580732793));
#43773=CARTESIAN_POINT('Ctrl Pts',(3.240232902369,-0.7659855665842,8.009696653886));
#43774=CARTESIAN_POINT('Ctrl Pts',(3.264295855207,-0.7681844468823,8.010377190337));
#43775=CARTESIAN_POINT('Ctrl Pts',(3.271420796559,-0.76950533233,8.010782594487));
#43776=CARTESIAN_POINT('Ctrl Pts',(2.792765104092,-1.991224869763,7.723406537252));
#43777=CARTESIAN_POINT('Ctrl Pts',(2.788537105428,-1.978678815405,7.721010757773));
#43778=CARTESIAN_POINT('Ctrl Pts',(2.756791097347,-1.881958605473,7.703051902518));
#43779=CARTESIAN_POINT('Ctrl Pts',(2.707875130552,-1.697202037034,7.675957994411));
#43780=CARTESIAN_POINT('Ctrl Pts',(2.667269448356,-1.433978002984,7.651213835617));
#43781=CARTESIAN_POINT('Ctrl Pts',(2.655188267488,-1.188072643789,7.63769259235));
#43782=CARTESIAN_POINT('Ctrl Pts',(2.669252075638,-0.9625884713048,7.63275022109));
#43783=CARTESIAN_POINT('Ctrl Pts',(2.708556680229,-0.7591881016237,7.63436877623));
#43784=CARTESIAN_POINT('Ctrl Pts',(2.773606268264,-0.5803351016669,7.640737884484));
#43785=CARTESIAN_POINT('Ctrl Pts',(2.865015042587,-0.4307700699685,7.649762753622));
#43786=CARTESIAN_POINT('Ctrl Pts',(2.980841699795,-0.3181327676405,7.658830046356));
#43787=CARTESIAN_POINT('Ctrl Pts',(3.112743733696,-0.2504501741924,7.6652140151));
#43788=CARTESIAN_POINT('Ctrl Pts',(3.224577167091,-0.2326920076717,7.666977451746));
#43789=CARTESIAN_POINT('Ctrl Pts',(3.287204681318,-0.2368974193595,7.666582838974));
#43790=CARTESIAN_POINT('Ctrl Pts',(3.305617539918,-0.2394455144739,7.666401482426));
#43791=CARTESIAN_POINT('Ctrl Pts',(2.354707813324,-1.817087042029,7.300711712326));
#43792=CARTESIAN_POINT('Ctrl Pts',(2.34719425366,-1.803021267319,7.302353914292));
#43793=CARTESIAN_POINT('Ctrl Pts',(2.290915031225,-1.694244596348,7.31560478624));
#43794=CARTESIAN_POINT('Ctrl Pts',(2.206032845101,-1.481950544316,7.349512634112));
#43795=CARTESIAN_POINT('Ctrl Pts',(2.139909159661,-1.170091282631,7.413473773373));
#43796=CARTESIAN_POINT('Ctrl Pts',(2.126223235302,-0.8711180476606,7.483575579401));
#43797=CARTESIAN_POINT('Ctrl Pts',(2.160037805531,-0.5901682844192,7.555449904233));
#43798=CARTESIAN_POINT('Ctrl Pts',(2.239342696343,-0.3303374624533,7.626078694443));
#43799=CARTESIAN_POINT('Ctrl Pts',(2.364778982571,-0.09589688494384,7.692513876796));
#43800=CARTESIAN_POINT('Ctrl Pts',(2.537224667366,0.105246040717,7.750964265596));
#43801=CARTESIAN_POINT('Ctrl Pts',(2.752985727524,0.2602729087259,7.79651453519));
#43802=CARTESIAN_POINT('Ctrl Pts',(2.996933379488,0.3550315871828,7.824430482657));
#43803=CARTESIAN_POINT('Ctrl Pts',(3.203127274003,0.3801014864107,7.831768774722));
#43804=CARTESIAN_POINT('Ctrl Pts',(3.318595594879,0.3741633816109,7.830072397969));
#43805=CARTESIAN_POINT('Ctrl Pts',(3.352552019354,0.3705590653944,7.82915107849));
#43806=CARTESIAN_POINT('Ctrl Pts',(1.722078738097,-1.841162035607,7.310012002466));
#43807=CARTESIAN_POINT('Ctrl Pts',(1.714517855214,-1.82325387619,7.318210429835));
#43808=CARTESIAN_POINT('Ctrl Pts',(1.658918378237,-1.685294382398,7.381280276636));
#43809=CARTESIAN_POINT('Ctrl Pts',(1.589006788219,-1.423058481785,7.500753094977));
#43810=CARTESIAN_POINT('Ctrl Pts',(1.568209302474,-1.051506193311,7.667791090927));
#43811=CARTESIAN_POINT('Ctrl Pts',(1.613417879879,-0.7047595538035,7.821222793726));
#43812=CARTESIAN_POINT('Ctrl Pts',(1.714294320514,-0.3859681540512,7.959996344744));
#43813=CARTESIAN_POINT('Ctrl Pts',(1.865759429155,-0.0966333636266,8.083750427066));
#43814=CARTESIAN_POINT('Ctrl Pts',(2.066526668314,0.1601126450525,8.191369643204));
#43815=CARTESIAN_POINT('Ctrl Pts',(2.315861782763,0.3772080734943,8.280260680351));
#43816=CARTESIAN_POINT('Ctrl Pts',(2.608197466777,0.542551163196,8.346280004011));
#43817=CARTESIAN_POINT('Ctrl Pts',(2.926010971638,0.6427899774458,8.38547381194));
#43818=CARTESIAN_POINT('Ctrl Pts',(3.189996159877,0.6692080185729,8.395646328464));
#43819=CARTESIAN_POINT('Ctrl Pts',(3.337814974144,0.6629510827252,8.393278067348));
#43820=CARTESIAN_POINT('Ctrl Pts',(3.381343738726,0.6591564736418,8.391950440612));
#43821=CARTESIAN_POINT('',(1.75000000021594,-1.78647023985835,7.3336606126813));
#43822=CARTESIAN_POINT('Origin',(1.75,-2.186029020505,8.250368190795));
#43823=CARTESIAN_POINT('',(3.25,-0.04336631913618,7.86687525911));
#43824=CARTESIAN_POINT('Origin',(3.25,-0.2250371090282,8.850234666499));
#43825=CARTESIAN_POINT('Ctrl Pts',(1.75000000048586,-1.78647023867652,7.33366060996403));
#43826=CARTESIAN_POINT('Ctrl Pts',(1.75001261091093,-1.67132937033661,7.38385324834833));
#43827=CARTESIAN_POINT('Ctrl Pts',(1.77542675361188,-1.45285226422692,7.47262865678146));
#43828=CARTESIAN_POINT('Ctrl Pts',(1.861160899812,-1.164361559054,7.576243569427));
#43829=CARTESIAN_POINT('Ctrl Pts',(1.977195804371,-0.9138167090022,7.656329079677));
#43830=CARTESIAN_POINT('Ctrl Pts',(2.112596345794,-0.6991889689988,7.717855015608));
#43831=CARTESIAN_POINT('Ctrl Pts',(2.261791685601,-0.5166888823143,7.765159563871));
#43832=CARTESIAN_POINT('Ctrl Pts',(2.421231729676,-0.3644382359967,7.801148505907));
#43833=CARTESIAN_POINT('Ctrl Pts',(2.587582423301,-0.2420433787695,7.827817542484));
#43834=CARTESIAN_POINT('Ctrl Pts',(2.757987815569,-0.1491336781293,7.84673056923));
#43835=CARTESIAN_POINT('Ctrl Pts',(2.929826816222,-0.08520576210219,7.859080936862));
#43836=CARTESIAN_POINT('Ctrl Pts',(3.096992661939,-0.04997560015663,7.865659537624));
#43837=CARTESIAN_POINT('Ctrl Pts',(3.200093400178,-0.04336596610774,7.866875225272));
#43838=CARTESIAN_POINT('Ctrl Pts',(3.25,-0.04336631913618,7.86687525911));
#43839=CARTESIAN_POINT('Origin',(1.75,1.41,0.));
#43840=CARTESIAN_POINT('',(1.75,-5.923658654762,3.196474735617));
#43841=CARTESIAN_POINT('Origin',(1.75,-6.840365986607,3.596034077569));
#43842=CARTESIAN_POINT('Origin',(1.75,1.41,0.));
#43843=CARTESIAN_POINT('Ctrl Pts',(3.271450805884,-6.600784524332,2.179511695863));
#43844=CARTESIAN_POINT('Ctrl Pts',(3.264316214845,-6.600377874579,2.178186642191));
#43845=CARTESIAN_POINT('Ctrl Pts',(3.240231918653,-6.599695561688,2.175981939566));
#43846=CARTESIAN_POINT('Ctrl Pts',(3.197202365664,-6.602584594832,2.185291506928));
#43847=CARTESIAN_POINT('Ctrl Pts',(3.141761803778,-6.613837343706,2.222175058386));
#43848=CARTESIAN_POINT('Ctrl Pts',(3.083432184706,-6.633291854611,2.288342755621));
#43849=CARTESIAN_POINT('Ctrl Pts',(3.023840460015,-6.66019722422,2.384794977911));
#43850=CARTESIAN_POINT('Ctrl Pts',(2.964463630781,-6.693298019679,2.511543641683));
#43851=CARTESIAN_POINT('Ctrl Pts',(2.906684619961,-6.731189795874,2.66885803549));
#43852=CARTESIAN_POINT('Ctrl Pts',(2.852103604317,-6.772317939251,2.857792631679));
#43853=CARTESIAN_POINT('Ctrl Pts',(2.803187857468,-6.814706270047,3.080231240091));
#43854=CARTESIAN_POINT('Ctrl Pts',(2.764302638213,-6.85538301175,3.337654190934));
#43855=CARTESIAN_POINT('Ctrl Pts',(2.750023886213,-6.878666337879,3.535090238471));
#43856=CARTESIAN_POINT('Ctrl Pts',(2.748171519073,-6.888664773212,3.644483876021));
#43857=CARTESIAN_POINT('Ctrl Pts',(2.748037895908,-6.889914238717,3.658707376734));
#43858=CARTESIAN_POINT('Ctrl Pts',(3.305695023565,-6.256408875213,1.649469417717));
#43859=CARTESIAN_POINT('Ctrl Pts',(3.287257504913,-6.256590398572,1.646913457279));
#43860=CARTESIAN_POINT('Ctrl Pts',(3.224574537333,-6.256985835413,1.642697452954));
#43861=CARTESIAN_POINT('Ctrl Pts',(3.112635733078,-6.255219576771,1.660485800177));
#43862=CARTESIAN_POINT('Ctrl Pts',(2.980650256738,-6.248826651561,1.728271881478));
#43863=CARTESIAN_POINT('Ctrl Pts',(2.864782305834,-6.239750546342,1.841066970101));
#43864=CARTESIAN_POINT('Ctrl Pts',(2.773367855811,-6.230722480542,1.990835841996));
#43865=CARTESIAN_POINT('Ctrl Pts',(2.708363725574,-6.224362431101,2.169903227412));
#43866=CARTESIAN_POINT('Ctrl Pts',(2.669158301008,-6.222767402465,2.373417325382));
#43867=CARTESIAN_POINT('Ctrl Pts',(2.655195161133,-6.22773834187,2.598889472782));
#43868=CARTESIAN_POINT('Ctrl Pts',(2.667348643033,-6.241277363413,2.844712958734));
#43869=CARTESIAN_POINT('Ctrl Pts',(2.707993195755,-6.266049883286,3.107654258154));
#43870=CARTESIAN_POINT('Ctrl Pts',(2.756810997999,-6.293038359982,3.292099408065));
#43871=CARTESIAN_POINT('Ctrl Pts',(2.788464197933,-6.310948959069,3.38854088252));
#43872=CARTESIAN_POINT('Ctrl Pts',(2.792655545842,-6.313325094994,3.400979580454));
#43873=CARTESIAN_POINT('Ctrl Pts',(3.352694515196,-6.419142450118,1.039481056806));
#43874=CARTESIAN_POINT('Ctrl Pts',(3.318692730551,-6.420065951233,1.035865662458));
#43875=CARTESIAN_POINT('Ctrl Pts',(3.203122611875,-6.421766407795,1.029912756346));
#43876=CARTESIAN_POINT('Ctrl Pts',(2.996735102831,-6.414415900882,1.055025197856));
#43877=CARTESIAN_POINT('Ctrl Pts',(2.752632908899,-6.386458010439,1.149927772965));
#43878=CARTESIAN_POINT('Ctrl Pts',(2.536792417474,-6.340846931723,1.305166068799));
#43879=CARTESIAN_POINT('Ctrl Pts',(2.36433046361,-6.282324327712,1.506570330996));
#43880=CARTESIAN_POINT('Ctrl Pts',(2.238971023845,-6.215824387893,1.741270810204));
#43881=CARTESIAN_POINT('Ctrl Pts',(2.159845582096,-6.145179984273,2.001219054871));
#43882=CARTESIAN_POINT('Ctrl Pts',(2.126218782839,-6.073339305311,2.282127143621));
#43883=CARTESIAN_POINT('Ctrl Pts',(2.14004402452,-6.003289201097,2.580974729488));
#43884=CARTESIAN_POINT('Ctrl Pts',(2.206252171837,-5.939446912097,2.892483751437));
#43885=CARTESIAN_POINT('Ctrl Pts',(2.290967627635,-5.905574269497,3.104384124248));
#43886=CARTESIAN_POINT('Ctrl Pts',(2.347082827887,-5.89237152092,3.212853022938));
#43887=CARTESIAN_POINT('Ctrl Pts',(2.354531186858,-5.890744549661,3.226799824363));
#43888=CARTESIAN_POINT('Ctrl Pts',(3.381527042583,-6.981918423624,0.7508744730096));
#43889=CARTESIAN_POINT('Ctrl Pts',(3.33793980561,-6.983249539883,0.7470681478622));
#43890=CARTESIAN_POINT('Ctrl Pts',(3.189989944912,-6.985623678342,0.7407954945952));
#43891=CARTESIAN_POINT('Ctrl Pts',(2.925754637913,-6.975433994821,0.7672586248663));
#43892=CARTESIAN_POINT('Ctrl Pts',(2.607728547645,-6.936180022559,0.8676509822134));
#43893=CARTESIAN_POINT('Ctrl Pts',(2.315255948472,-6.870066961331,1.033223765781));
#43894=CARTESIAN_POINT('Ctrl Pts',(2.065845059635,-6.781052513204,1.250609837518));
#43895=CARTESIAN_POINT('Ctrl Pts',(1.865111694256,-6.673301299875,1.507655263828));
#43896=CARTESIAN_POINT('Ctrl Pts',(1.713837092142,-6.549474404633,1.797142544492));
#43897=CARTESIAN_POINT('Ctrl Pts',(1.613202352312,-6.410704136534,2.115912157827));
#43898=CARTESIAN_POINT('Ctrl Pts',(1.568201988779,-6.257320639317,2.462537074865));
#43899=CARTESIAN_POINT('Ctrl Pts',(1.589188572213,-6.090455036669,2.833709173528));
#43900=CARTESIAN_POINT('Ctrl Pts',(1.658984742568,-5.97119718329,3.095447355188));
#43901=CARTESIAN_POINT('Ctrl Pts',(1.714424163993,-5.908325889543,3.23301009736));
#43902=CARTESIAN_POINT('Ctrl Pts',(1.721918698242,-5.900199786108,3.250765686424));
#43903=CARTESIAN_POINT('',(3.25,-6.574209262715,2.135037109028));
#43904=CARTESIAN_POINT('',(3.25,-6.45687525911,1.453366319136));
#43905=CARTESIAN_POINT('Origin',(3.25,-7.440234666499,1.635037109028));
#43906=CARTESIAN_POINT('Ctrl Pts',(3.25,-6.57420926271478,2.13503710902813));
#43907=CARTESIAN_POINT('Ctrl Pts',(3.24051328877442,-6.574209580288,2.13503810640009));
#43908=CARTESIAN_POINT('Ctrl Pts',(3.23080615598635,-6.57445243030741,2.13600227329107));
#43909=CARTESIAN_POINT('Ctrl Pts',(3.22087230023474,-6.57497097820664,2.1380598369659));
#43910=CARTESIAN_POINT('Ctrl Pts',(3.21347574283905,-6.57535707897103,2.13959185919339));
#43911=CARTESIAN_POINT('Ctrl Pts',(3.20595370673705,-6.57589625420415,2.14173100212492));
#43912=CARTESIAN_POINT('Ctrl Pts',(3.19831104571938,-6.57660635689357,2.14454781654446));
#43913=CARTESIAN_POINT('Ctrl Pts',(3.19651447281003,-6.57677328190198,2.14520996974805));
#43914=CARTESIAN_POINT('Ctrl Pts',(3.19471116015858,-6.57694922279033,2.14590888702886));
#43915=CARTESIAN_POINT('Ctrl Pts',(3.19290156425008,-6.57713442323191,2.14664549535018));
#43916=CARTESIAN_POINT('Ctrl Pts',(3.18189733676813,-6.57826063476863,2.15112484098472));
#43917=CARTESIAN_POINT('Ctrl Pts',(3.17065888397034,-6.57973024826778,2.1570014501285));
#43918=CARTESIAN_POINT('Ctrl Pts',(3.15927245949691,-6.58157034387027,2.16439079707255));
#43919=CARTESIAN_POINT('Ctrl Pts',(3.1538680298637,-6.58244372314971,2.16789806185859));
#43920=CARTESIAN_POINT('Ctrl Pts',(3.14843060788739,-6.58340039015426,2.17174550131682));
#43921=CARTESIAN_POINT('Ctrl Pts',(3.14297129559834,-6.58444227478407,2.17594186663245));
#43922=CARTESIAN_POINT('Ctrl Pts',(3.13920633189964,-6.58516080078181,2.17883585075412));
#43923=CARTESIAN_POINT('Ctrl Pts',(3.13542993069291,-6.5859193107831,2.18189527048653));
#43924=CARTESIAN_POINT('Ctrl Pts',(3.13164589470533,-6.58671786767652,2.18512186217636));
#43925=CARTESIAN_POINT('Ctrl Pts',(3.12069286106816,-6.58902932045964,2.1944613524529));
#43926=CARTESIAN_POINT('Ctrl Pts',(3.109675479807,-6.59167741438172,2.20520508063705));
#43927=CARTESIAN_POINT('Ctrl Pts',(3.09866120950954,-6.59464872736088,2.21734787551539));
#43928=CARTESIAN_POINT('Ctrl Pts',(3.09442640256284,-6.59579114864755,2.22201658172238));
#43929=CARTESIAN_POINT('Ctrl Pts',(3.09019212355419,-6.59698119320272,2.22689159758761));
#43930=CARTESIAN_POINT('Ctrl Pts',(3.08596246544424,-6.59821749385538,2.23197066469041));
#43931=CARTESIAN_POINT('Ctrl Pts',(3.08024996729594,-6.59988721869021,2.23883035894125));
#43932=CARTESIAN_POINT('Ctrl Pts',(3.07454429121136,-6.60164320384453,2.24606655891752));
#43933=CARTESIAN_POINT('Ctrl Pts',(3.06885114450466,-6.60348280832308,2.25367794990381));
#43934=CARTESIAN_POINT('Ctrl Pts',(3.05557765797147,-6.60777181869476,2.27142379433048));
#43935=CARTESIAN_POINT('Ctrl Pts',(3.04237135767047,-6.61251695827372,2.29121255884396));
#43936=CARTESIAN_POINT('Ctrl Pts',(3.02927014080688,-6.61768864373912,2.31306301272805));
#43937=CARTESIAN_POINT('Ctrl Pts',(3.02178682413499,-6.62064267163348,2.32554382787229));
#43938=CARTESIAN_POINT('Ctrl Pts',(3.01433747439815,-6.62373755466617,2.3387007727525));
#43939=CARTESIAN_POINT('Ctrl Pts',(3.00693454048262,-6.62696290842619,2.35252311012848));
#43940=CARTESIAN_POINT('Ctrl Pts',(2.99581808697545,-6.6318061902286,2.37327912018529));
#43941=CARTESIAN_POINT('Ctrl Pts',(2.98480625277407,-6.6369442289306,2.39553659560213));
#43942=CARTESIAN_POINT('Ctrl Pts',(2.97393305392326,-6.64235017239947,2.4193015558268));
#43943=CARTESIAN_POINT('Ctrl Pts',(2.96487468961802,-6.64685381535004,2.43909993074558));
#43944=CARTESIAN_POINT('Ctrl Pts',(2.95591340816756,-6.65154466262965,2.45994580479158));
#43945=CARTESIAN_POINT('Ctrl Pts',(2.94707248054145,-6.65639850762819,2.48181799973957));
#43946=CARTESIAN_POINT('Ctrl Pts',(2.93823408053821,-6.66125096491153,2.50368394142292));
#43947=CARTESIAN_POINT('Ctrl Pts',(2.92951596079112,-6.66626612348122,2.52657487624024));
#43948=CARTESIAN_POINT('Ctrl Pts',(2.92094383128304,-6.67142497211021,2.55049507921643));
#43949=CARTESIAN_POINT('Ctrl Pts',(2.91065031956988,-6.67761977688293,2.5792187340894));
#43950=CARTESIAN_POINT('Ctrl Pts',(2.90056879809431,-6.68402127602502,2.6094220654221));
#43951=CARTESIAN_POINT('Ctrl Pts',(2.8907337765054,-6.69059072399738,2.64112227472971));
#43952=CARTESIAN_POINT('Ctrl Pts',(2.88418583059476,-6.69496452120737,2.66222759249904));
#43953=CARTESIAN_POINT('Ctrl Pts',(2.87774725879252,-6.69941230199369,2.68399537478204));
#43954=CARTESIAN_POINT('Ctrl Pts',(2.87143408618968,-6.70392417886007,2.70644225837694));
#43955=CARTESIAN_POINT('Ctrl Pts',(2.86159165554342,-6.71095833394112,2.74143764166619));
#43956=CARTESIAN_POINT('Ctrl Pts',(2.85205449398499,-6.71814491868167,2.77807325337933));
#43957=CARTESIAN_POINT('Ctrl Pts',(2.84288373170243,-6.72544280974844,2.81644159973842));
#43958=CARTESIAN_POINT('Ctrl Pts',(2.84175743423344,-6.72633909252018,2.82115376761089));
#43959=CARTESIAN_POINT('Ctrl Pts',(2.84063668982235,-6.72723702172671,2.82589202074456));
#43960=CARTESIAN_POINT('Ctrl Pts',(2.83952163404616,-6.72813649253441,2.83065648517027));
#43961=CARTESIAN_POINT('Ctrl Pts',(2.83514517450144,-6.73166680705819,2.8493564338692));
#43962=CARTESIAN_POINT('Ctrl Pts',(2.83085621640419,-6.73522097501525,2.86846030126194));
#43963=CARTESIAN_POINT('Ctrl Pts',(2.82666626830219,-6.73879389815918,2.88798042967713));
#43964=CARTESIAN_POINT('Ctrl Pts',(2.81859266003575,-6.74567856143616,2.92559375239581));
#43965=CARTESIAN_POINT('Ctrl Pts',(2.81088601077042,-6.75262925430877,2.96474438901527));
#43966=CARTESIAN_POINT('Ctrl Pts',(2.80364920149339,-6.75958428980929,3.00546602378017));
#43967=CARTESIAN_POINT('Ctrl Pts',(2.80088318048451,-6.76224261250034,3.02103046564451));
#43968=CARTESIAN_POINT('Ctrl Pts',(2.79818602344303,-6.76490133183295,3.03682401832795));
#43969=CARTESIAN_POINT('Ctrl Pts',(2.79556434006813,-6.76755605070014,3.05284692811978));
#43970=CARTESIAN_POINT('Ctrl Pts',(2.79319374416818,-6.76995651817167,3.0673352697027));
#43971=CARTESIAN_POINT('Ctrl Pts',(2.79088485160737,-6.77235370295779,3.0820111151052));
#43972=CARTESIAN_POINT('Ctrl Pts',(2.78864396027109,-6.77474457481874,3.09687549807305));
#43973=CARTESIAN_POINT('Ctrl Pts',(2.78243004536069,-6.78137438058622,3.13809392284103));
#43974=CARTESIAN_POINT('Ctrl Pts',(2.77673782796066,-6.78795234727477,3.18075634451844));
#43975=CARTESIAN_POINT('Ctrl Pts',(2.77172743500744,-6.79439750337758,3.22480001727387));
#43976=CARTESIAN_POINT('Ctrl Pts',(2.76860707762661,-6.79841139821653,3.25222940268233));
#43977=CARTESIAN_POINT('Ctrl Pts',(2.76575155268839,-6.80237343980551,3.28019374186988));
#43978=CARTESIAN_POINT('Ctrl Pts',(2.76320363662809,-6.806260205241,3.30866920745312));
#43979=CARTESIAN_POINT('Ctrl Pts',(2.76246674850062,-6.80738430479368,3.31690465635168));
#43980=CARTESIAN_POINT('Ctrl Pts',(2.76175561008452,-6.80850208713546,3.32518281325778));
#43981=CARTESIAN_POINT('Ctrl Pts',(2.76107146865022,-6.80961300152605,3.33350267279286));
#43982=CARTESIAN_POINT('Ctrl Pts',(2.75804225864649,-6.81453185721365,3.3703409645109));
#43983=CARTESIAN_POINT('Ctrl Pts',(2.75553951217967,-6.81931358854474,3.40799423196495));
#43984=CARTESIAN_POINT('Ctrl Pts',(2.75367822980329,-6.82391801056441,3.44648708900259));
#43985=CARTESIAN_POINT('Ctrl Pts',(2.75194379522927,-6.82820863773932,3.48235662870593));
#43986=CARTESIAN_POINT('Ctrl Pts',(2.75076637573596,-6.83234532670531,3.5189555638735));
#43987=CARTESIAN_POINT('Ctrl Pts',(2.75026751838297,-6.83628130815854,3.55627119138643));
#43988=CARTESIAN_POINT('Ctrl Pts',(2.75009151577668,-6.83766996764193,3.56943657355102));
#43989=CARTESIAN_POINT('Ctrl Pts',(2.75000025092927,-6.83903350525114,3.58269083008542));
#43990=CARTESIAN_POINT('Ctrl Pts',(2.7500000000008,-6.84036938720128,3.59603220353762));
#43991=CARTESIAN_POINT('Ctrl Pts',(2.74999999998808,-6.84036945491068,3.59603287974736));
#43992=CARTESIAN_POINT('Ctrl Pts',(2.7499999999756,-6.84036952262001,3.59603355595731));
#43993=CARTESIAN_POINT('Ctrl Pts',(2.74999999996335,-6.84036959032926,3.59603423216749));
#43994=CARTESIAN_POINT('Ctrl Pts',(3.25,-6.45687525911025,1.45336631913605));
#43995=CARTESIAN_POINT('Ctrl Pts',(3.200061038244,-6.45687531917522,1.45336599401248));
#43996=CARTESIAN_POINT('Ctrl Pts',(3.14847540739251,-6.4562670418847,1.45667483599627));
#43997=CARTESIAN_POINT('Ctrl Pts',(3.09479707713993,-6.45486414723981,1.46421034877569));
#43998=CARTESIAN_POINT('Ctrl Pts',(3.04111874688734,-6.45346125259492,1.47174586155511));
#43999=CARTESIAN_POINT('Ctrl Pts',(2.98534771723367,-6.45126498433326,1.48350827579869));
#44000=CARTESIAN_POINT('Ctrl Pts',(2.92880284639516,-6.44810528300073,1.50006045254051));
#44001=CARTESIAN_POINT('Ctrl Pts',(2.87225797555666,-6.4449455816682,1.51661262928234));
#44002=CARTESIAN_POINT('Ctrl Pts',(2.81493926353333,-6.44082214246287,1.53795450990436));
#44003=CARTESIAN_POINT('Ctrl Pts',(2.75786489396516,-6.43560370021495,1.56412997515346));
#44004=CARTESIAN_POINT('Ctrl Pts',(2.700790524397,-6.43038525796702,1.59030544040256));
#44005=CARTESIAN_POINT('Ctrl Pts',(2.643960497284,-6.4240722818765,1.62131458592504));
#44006=CARTESIAN_POINT('Ctrl Pts',(2.58779565893966,-6.41646225785502,1.65725330784731));
#44007=CARTESIAN_POINT('Ctrl Pts',(2.53512661061407,-6.40932589398821,1.69095514582072));
#44008=CARTESIAN_POINT('Ctrl Pts',(2.48304252316936,-6.4010485467861,1.72899184972167));
#44009=CARTESIAN_POINT('Ctrl Pts',(2.43194867115751,-6.39141658065603,1.77141167859568));
#44010=CARTESIAN_POINT('Ctrl Pts',(2.42855743126309,-6.39077728049533,1.77422719964817));
#44011=CARTESIAN_POINT('Ctrl Pts',(2.42517055369546,-6.39013199469215,1.77706202360263));
#44012=CARTESIAN_POINT('Ctrl Pts',(2.42178815695477,-6.38948065302519,1.77991616181372));
#44013=CARTESIAN_POINT('Ctrl Pts',(2.37166766403781,-6.37982904562717,1.82220889828441));
#44014=CARTESIAN_POINT('Ctrl Pts',(2.3225310457101,-6.36885175503254,1.86874387943997));
#44015=CARTESIAN_POINT('Ctrl Pts',(2.27483701918363,-6.35629580130176,1.91954409344578));
#44016=CARTESIAN_POINT('Ctrl Pts',(2.27081892151714,-6.35523799486225,1.92382387932716));
#44017=CARTESIAN_POINT('Ctrl Pts',(2.2668110628251,-6.35416895545652,1.92813392605475));
#44018=CARTESIAN_POINT('Ctrl Pts',(2.26281371740039,-6.353088516178,1.93247424044547));
#44019=CARTESIAN_POINT('Ctrl Pts',(2.2201788328164,-6.34156476752845,1.97876716323444));
#44020=CARTESIAN_POINT('Ctrl Pts',(2.1787399299299,-6.32874810757987,2.02850464921655));
#44021=CARTESIAN_POINT('Ctrl Pts',(2.13882776655781,-6.31436833841078,2.08185824987127));
#44022=CARTESIAN_POINT('Ctrl Pts',(2.13058023305217,-6.31139687262177,2.0928833502885));
#44023=CARTESIAN_POINT('Ctrl Pts',(2.12239789278961,-6.30835849921372,2.10406278968684));
#44024=CARTESIAN_POINT('Ctrl Pts',(2.11428366431634,-6.3052505765884,2.11539796266622));
#44025=CARTESIAN_POINT('Ctrl Pts',(2.07988507840782,-6.29207518427888,2.16345107366793));
#44026=CARTESIAN_POINT('Ctrl Pts',(2.04671057025077,-6.27765365439441,2.21430410098874));
#44027=CARTESIAN_POINT('Ctrl Pts',(2.01509997230188,-6.26171202128629,2.26822279823904));
#44028=CARTESIAN_POINT('Ctrl Pts',(2.0031695090356,-6.25569533446156,2.28857277826633));
#44029=CARTESIAN_POINT('Ctrl Pts',(1.99146181797665,-6.24946164733413,2.30935923610152));
#44030=CARTESIAN_POINT('Ctrl Pts',(1.97999516912917,-6.24299445217726,2.33059561377431));
#44031=CARTESIAN_POINT('Ctrl Pts',(1.94999818237139,-6.22607613802455,2.38615040997562));
#44032=CARTESIAN_POINT('Ctrl Pts',(1.92165078304898,-6.20756304660474,2.4447853243894));
#44033=CARTESIAN_POINT('Ctrl Pts',(1.89563069728732,-6.18715556759926,2.50663664732157));
#44034=CARTESIAN_POINT('Ctrl Pts',(1.88535055886863,-6.17909288437544,2.53107316021189));
#44035=CARTESIAN_POINT('Ctrl Pts',(1.87543369533783,-6.17073402192865,2.55601144677107));
#44036=CARTESIAN_POINT('Ctrl Pts',(1.865921901754,-6.1620585630372,2.58145871900657));
#44037=CARTESIAN_POINT('Ctrl Pts',(1.84188066661732,-6.14013117938556,2.64577717272496));
#44038=CARTESIAN_POINT('Ctrl Pts',(1.82042716017291,-6.11618429015519,2.71334849296128));
#44039=CARTESIAN_POINT('Ctrl Pts',(1.80262601149376,-6.08988601050222,2.78418925891778));
#44040=CARTESIAN_POINT('Ctrl Pts',(1.79555783429077,-6.07944393712419,2.81231750479677));
#44041=CARTESIAN_POINT('Ctrl Pts',(1.78906548420749,-6.06863070306812,2.84096085726446));
#44042=CARTESIAN_POINT('Ctrl Pts',(1.78321560761792,-6.05742376295122,2.87011887288863));
#44043=CARTESIAN_POINT('Ctrl Pts',(1.76727058462547,-6.02687697874084,2.94959494771222));
#44044=CARTESIAN_POINT('Ctrl Pts',(1.75609878882583,-5.99340723684766,3.03289665525687));
#44045=CARTESIAN_POINT('Ctrl Pts',(1.75187206416855,-5.95661567846224,3.11977137717403));
#44046=CARTESIAN_POINT('Ctrl Pts',(1.75064269165845,-5.94591459567352,3.14503949932704));
#44047=CARTESIAN_POINT('Ctrl Pts',(1.75000085690326,-5.93493232465646,3.17060960179539));
#44048=CARTESIAN_POINT('Ctrl Pts',(1.75,-5.92365865476181,3.19647473561692));
#44049=CARTESIAN_POINT('Origin',(-41.76566382177,-7.440234666499,1.635037109028));
#44050=CARTESIAN_POINT('',(4.75,-6.45687525911,1.453366319136));
#44051=CARTESIAN_POINT('',(4.75,-6.574209262715,2.135037109028));
#44052=CARTESIAN_POINT('Origin',(4.75,-7.440234666499,1.635037109028));
#44053=CARTESIAN_POINT('',(4.75,-6.574209262851,2.135037109265));
#44054=CARTESIAN_POINT('',(3.25,-6.45687525911,1.453366319136));
#44055=CARTESIAN_POINT('Origin',(4.75,-7.440234666499,1.635037109028));
#44056=CARTESIAN_POINT('Origin',(4.75,-5.965195555416,1.36253092419));
#44057=CARTESIAN_POINT('Origin',(4.75,-6.141196560822,2.385037109028));
#44058=CARTESIAN_POINT('Origin',(4.75,-6.110531496591,2.331923659762));
#44059=CARTESIAN_POINT('',(4.75,-8.966250804401,6.278174593044));
#44060=CARTESIAN_POINT('',(4.75,-6.574209262851,2.135037109265));
#44061=CARTESIAN_POINT('Origin',(4.75,-8.533238102513,6.528174593052));
#44062=CARTESIAN_POINT('Origin',(5.25,-8.966250804405,6.278174593052));
#44063=CARTESIAN_POINT('',(3.25,-8.966250804405,6.278174593052));
#44064=CARTESIAN_POINT('',(4.75,-8.966250804401,6.278174593044));
#44065=CARTESIAN_POINT('',(3.25,-8.966250804398,6.278174593039));
#44066=CARTESIAN_POINT('Origin',(3.25,-6.461881837768,2.940480301938));
#44067=CARTESIAN_POINT('Origin',(3.25,-8.533238102513,6.528174593052));
#44068=CARTESIAN_POINT('Origin',(3.25,-6.368174593052,7.778174593052));
#44069=CARTESIAN_POINT('Origin',(3.25,-6.368174593052,7.778174593052));
#44070=CARTESIAN_POINT('Origin',(5.25,-6.368174593052,7.778174593052));
#44071=CARTESIAN_POINT('',(4.75,-4.868174593052,10.37625080441));
#44072=CARTESIAN_POINT('Origin',(4.75,-6.368174593052,7.778174593052));
#44073=CARTESIAN_POINT('',(4.75,-4.868174593043,10.3762508044));
#44074=CARTESIAN_POINT('Origin',(4.75,-6.368174593052,7.778174593052));
#44075=CARTESIAN_POINT('Origin',(4.75,-5.118174593052,9.943238102513));
#44076=CARTESIAN_POINT('Origin',(4.75,-5.171288042318,9.973903166745));
#44077=CARTESIAN_POINT('',(4.75,-0.7250371092557,7.984209262846));
#44078=CARTESIAN_POINT('',(4.75,-4.868174593043,10.3762508044));
#44079=CARTESIAN_POINT('Origin',(4.75,-0.9750371090282,7.551196560822));
#44080=CARTESIAN_POINT('Origin',(5.25,-0.3950637418857,7.793699050369));
#44081=CARTESIAN_POINT('',(3.25,-0.7250371090282,7.984209262715));
#44082=CARTESIAN_POINT('Origin',(33.40462042024,-0.2250371090282,8.850234666499));
#44083=CARTESIAN_POINT('',(4.75,-0.04336631913618,7.86687525911));
#44084=CARTESIAN_POINT('Origin',(4.75,-0.2250371090282,8.850234666499));
#44085=CARTESIAN_POINT('',(4.75,-0.04336631887412,7.866875259159));
#44086=CARTESIAN_POINT('Origin',(4.75,-0.2250371090282,8.850234666499));
#44087=CARTESIAN_POINT('Origin',(4.75,0.04746907580983,7.375195555416));
#44088=CARTESIAN_POINT('Origin',(4.75,1.41,0.));
#44089=CARTESIAN_POINT('',(4.75,1.41,8.));
#44090=CARTESIAN_POINT('Origin',(4.75,1.41,0.));
#44091=CARTESIAN_POINT('Origin',(4.75,1.41,7.5));
#44092=CARTESIAN_POINT('Origin',(-4.6,1.41,0.));
#44093=CARTESIAN_POINT('',(4.75,1.410000000002,-8.));
#44094=CARTESIAN_POINT('Origin',(4.75,1.41,0.));
#44095=CARTESIAN_POINT('',(-4.1,1.410000000002,8.));
#44096=CARTESIAN_POINT('',(-4.1,1.410000000002,8.));
#44097=CARTESIAN_POINT('',(-4.1,1.41,-8.));
#44098=CARTESIAN_POINT('Origin',(-4.1,1.41,0.));
#44099=CARTESIAN_POINT('',(-4.1,1.410000000002,-8.));
#44100=CARTESIAN_POINT('Origin',(4.75,1.41,0.));
#44101=CARTESIAN_POINT('Origin',(4.75,1.41,-7.5));
#44102=CARTESIAN_POINT('Origin',(4.75,4.213822859968,-7.5));
#44103=CARTESIAN_POINT('',(4.75000019975999,3.6383472114225,-8.00000004058105));
#44104=CARTESIAN_POINT('',(4.75000019976,3.638347231863,-8.000000176328));
#44105=CARTESIAN_POINT('Origin',(4.75,3.638347150101,-7.5));
#44106=CARTESIAN_POINT('Origin',(-4.6,1.41,-8.));
#44107=CARTESIAN_POINT('',(-4.09999992634177,3.59647863879817,-8.00000011306536));
#44108=CARTESIAN_POINT('',(-4.1,1.410000000002,-8.));
#44109=CARTESIAN_POINT('',(-1.576219094765,2.688757347123,-8.));
#44110=CARTESIAN_POINT('Ctrl Pts',(-4.099999915327,3.596478469713,-8.));
#44111=CARTESIAN_POINT('Ctrl Pts',(-4.018359390359,3.529042992373,-8.));
#44112=CARTESIAN_POINT('Ctrl Pts',(-3.93452530619,3.465279502913,-8.));
#44113=CARTESIAN_POINT('Ctrl Pts',(-3.84862157962933,3.40513255040783,-8.));
#44114=CARTESIAN_POINT('Ctrl Pts',(-3.76271785306867,3.34498559790267,-8.));
#44115=CARTESIAN_POINT('Ctrl Pts',(-3.67474448411633,3.28845518235233,-8.));
#44116=CARTESIAN_POINT('Ctrl Pts',(-3.58456988763017,3.23541665283533,-8.));
#44117=CARTESIAN_POINT('Ctrl Pts',(-3.494395291144,3.18237812331833,-8.));
#44118=CARTESIAN_POINT('Ctrl Pts',(-3.402019467124,3.13283147983467,-8.));
#44119=CARTESIAN_POINT('Ctrl Pts',(-3.307166927403,3.08676170221583,-8.));
#44120=CARTESIAN_POINT('Ctrl Pts',(-3.212314387682,3.040691924597,-8.));
#44121=CARTESIAN_POINT('Ctrl Pts',(-3.11498513226,2.998099012843,-8.));
#44122=CARTESIAN_POINT('Ctrl Pts',(-3.0152306510545,2.95919441423967,-8.));
#44123=CARTESIAN_POINT('Ctrl Pts',(-2.915476169849,2.92028981563633,-8.));
#44124=CARTESIAN_POINT('Ctrl Pts',(-2.81329646286,2.88507353018367,-8.));
#44125=CARTESIAN_POINT('Ctrl Pts',(-2.706913955166,2.8534050156445,-8.));
#44126=CARTESIAN_POINT('Ctrl Pts',(-2.600531447472,2.82173650110533,-8.));
#44127=CARTESIAN_POINT('Ctrl Pts',(-2.489946139073,2.79361575747967,-8.));
#44128=CARTESIAN_POINT('Ctrl Pts',(-2.37284548982433,2.76958445078183,-8.));
#44129=CARTESIAN_POINT('Ctrl Pts',(-2.25574484057567,2.745553144084,-8.));
#44130=CARTESIAN_POINT('Ctrl Pts',(-2.13212885047733,2.725611274314,-8.));
#44131=CARTESIAN_POINT('Ctrl Pts',(-1.99962443142992,2.711412599665,-8.));
#44132=CARTESIAN_POINT('Ctrl Pts',(-1.8671200123825,2.697213925016,-8.));
#44133=CARTESIAN_POINT('Ctrl Pts',(-1.725727164386,2.688758445488,-8.));
#44134=CARTESIAN_POINT('Ctrl Pts',(-1.576219094765,2.688757347123,-8.));
#44135=CARTESIAN_POINT('',(2.16937313768,2.688757347123,-8.));
#44136=CARTESIAN_POINT('',(-1.576219094765,2.688757347123,-8.));
#44137=CARTESIAN_POINT('Ctrl Pts',(2.16937313768,2.688757347123,-8.));
#44138=CARTESIAN_POINT('Ctrl Pts',(2.284499469128,2.688757798533,-8.));
#44139=CARTESIAN_POINT('Ctrl Pts',(2.3964607117535,2.6937462920655,-8.));
#44140=CARTESIAN_POINT('Ctrl Pts',(2.50432998544575,2.70274264988892,-8.));
#44141=CARTESIAN_POINT('Ctrl Pts',(2.612199259138,2.71173900771233,-8.));
#44142=CARTESIAN_POINT('Ctrl Pts',(2.715976563897,2.72474322982667,-8.));
#44143=CARTESIAN_POINT('Ctrl Pts',(2.81844949985083,2.7415977468805,-8.));
#44144=CARTESIAN_POINT('Ctrl Pts',(2.92092243580467,2.75845226393433,-8.));
#44145=CARTESIAN_POINT('Ctrl Pts',(3.02209100295334,2.77915707592767,-8.));
#44146=CARTESIAN_POINT('Ctrl Pts',(3.12132923442132,2.80345374875183,-8.));
#44147=CARTESIAN_POINT('Ctrl Pts',(3.22056746588931,2.82775042157599,-8.));
#44148=CARTESIAN_POINT('Ctrl Pts',(3.31787536167661,2.85563895523098,-8.));
#44149=CARTESIAN_POINT('Ctrl Pts',(3.41368272796592,2.88706205193797,-8.));
#44150=CARTESIAN_POINT('Ctrl Pts',(3.50949009425531,2.91848514864499,-8.));
#44151=CARTESIAN_POINT('Ctrl Pts',(3.6037969310467,2.95344280840401,-8.));
#44152=CARTESIAN_POINT('Ctrl Pts',(3.69671207446142,2.99197095919337,-8.));
#44153=CARTESIAN_POINT('Ctrl Pts',(3.78962721787606,3.03049910998269,-8.));
#44154=CARTESIAN_POINT('Ctrl Pts',(3.88115066791403,3.07259775180235,-8.));
#44155=CARTESIAN_POINT('Ctrl Pts',(3.97141476700251,3.11841262290817,-8.));
#44156=CARTESIAN_POINT('Ctrl Pts',(4.061678866091,3.164227494014,-8.));
#44157=CARTESIAN_POINT('Ctrl Pts',(4.15068361423,3.213758594406,-8.));
#44158=CARTESIAN_POINT('Ctrl Pts',(4.2384834233655,3.26725712317767,-8.));
#44159=CARTESIAN_POINT('Ctrl Pts',(4.326283232501,3.32075565194933,-8.));
#44160=CARTESIAN_POINT('Ctrl Pts',(4.412878102633,3.37822160910067,-8.));
#44161=CARTESIAN_POINT('Ctrl Pts',(4.49819320382275,3.43997159218608,-8.));
#44162=CARTESIAN_POINT('Ctrl Pts',(4.58350830152976,3.50172157275074,-8.));
#44163=CARTESIAN_POINT('Ctrl Pts',(4.66754363039901,3.56775557889971,-8.));
#44164=CARTESIAN_POINT('Ctrl Pts',(4.75000018966185,3.63834722321791,-8.));
#44165=CARTESIAN_POINT('Ctrl Pts',(2.116278824535,3.685575955387,-8.914669819439));
#44166=CARTESIAN_POINT('Ctrl Pts',(2.133974364313,3.685202511829,-8.913936796476));
#44167=CARTESIAN_POINT('Ctrl Pts',(2.239909103176,3.683895874728,-8.90958933508));
#44168=CARTESIAN_POINT('Ctrl Pts',(2.429044891448,3.691486482049,-8.902264402712));
#44169=CARTESIAN_POINT('Ctrl Pts',(2.679654460364,3.723106835226,-8.893510969338));
#44170=CARTESIAN_POINT('Ctrl Pts',(2.918517115661,3.77349021367,-8.886064087219));
#44171=CARTESIAN_POINT('Ctrl Pts',(3.148793502593,3.841976725606,-8.879768421771));
#44172=CARTESIAN_POINT('Ctrl Pts',(3.371320421461,3.928221561954,-8.874576435951));
#44173=CARTESIAN_POINT('Ctrl Pts',(3.586961347311,4.032566912426,-8.870469771728));
#44174=CARTESIAN_POINT('Ctrl Pts',(3.796243341077,4.155927546394,-8.867468981321));
#44175=CARTESIAN_POINT('Ctrl Pts',(3.999311125999,4.299791587489,-8.865635475613));
#44176=CARTESIAN_POINT('Ctrl Pts',(4.196870836309,4.467121255863,-8.865073355886));
#44177=CARTESIAN_POINT('Ctrl Pts',(4.390781885124,4.664118803414,-8.865984111162));
#44178=CARTESIAN_POINT('Ctrl Pts',(4.58185832671,4.900643864149,-8.868774418082));
#44179=CARTESIAN_POINT('Ctrl Pts',(4.766586072556,5.188641909635,-8.874118740203));
#44180=CARTESIAN_POINT('Ctrl Pts',(4.935004609316,5.539877033665,-8.882942615775));
#44181=CARTESIAN_POINT('Ctrl Pts',(5.06881085959,5.961167749208,-8.896284405282));
#44182=CARTESIAN_POINT('Ctrl Pts',(5.142480202847,6.444827636589,-8.914820452271));
#44183=CARTESIAN_POINT('Ctrl Pts',(5.134565454299,6.910226196755,-8.935812671574));
#44184=CARTESIAN_POINT('Ctrl Pts',(5.086154708016,7.20557677316,-8.950861426659));
#44185=CARTESIAN_POINT('Ctrl Pts',(5.059038787903,7.325804132106,-8.957281445266));
#44186=CARTESIAN_POINT('Ctrl Pts',(2.1154288364,3.637085259508,-8.348384030449));
#44187=CARTESIAN_POINT('Ctrl Pts',(2.133400208805,3.636290273659,-8.347686475024));
#44188=CARTESIAN_POINT('Ctrl Pts',(2.241031179989,3.632497380359,-8.343553235046));
#44189=CARTESIAN_POINT('Ctrl Pts',(2.433665358953,3.636061516638,-8.33661798874));
#44190=CARTESIAN_POINT('Ctrl Pts',(2.689779275819,3.66336607149,-8.328377510496));
#44191=CARTESIAN_POINT('Ctrl Pts',(2.934551817168,3.710677008797,-8.321401663127));
#44192=CARTESIAN_POINT('Ctrl Pts',(3.171022006258,3.777280474976,-8.315529203019));
#44193=CARTESIAN_POINT('Ctrl Pts',(3.399874678972,3.862820491692,-8.310703523916));
#44194=CARTESIAN_POINT('Ctrl Pts',(3.621834783565,3.96763839521,-8.306897709465));
#44195=CARTESIAN_POINT('Ctrl Pts',(3.837283647501,4.092660683915,-8.304122996033));
#44196=CARTESIAN_POINT('Ctrl Pts',(4.046201161548,4.239396089147,-8.302430243022));
#44197=CARTESIAN_POINT('Ctrl Pts',(4.249124654791,4.410851402467,-8.30191168612));
#44198=CARTESIAN_POINT('Ctrl Pts',(4.447727052512,4.613350620516,-8.302751920613));
#44199=CARTESIAN_POINT('Ctrl Pts',(4.642490961035,4.856958632612,-8.305328882577));
#44200=CARTESIAN_POINT('Ctrl Pts',(4.829272674408,5.153781459785,-8.310276411291));
#44201=CARTESIAN_POINT('Ctrl Pts',(4.997130608976,5.515463539827,-8.318479830472));
#44202=CARTESIAN_POINT('Ctrl Pts',(5.126539475247,5.948065657011,-8.330966280555));
#44203=CARTESIAN_POINT('Ctrl Pts',(5.191058871723,6.442132504575,-8.348484454665));
#44204=CARTESIAN_POINT('Ctrl Pts',(5.170988750385,6.91385957546,-8.368577870152));
#44205=CARTESIAN_POINT('Ctrl Pts',(5.113623097214,7.210715672424,-8.383180326519));
#44206=CARTESIAN_POINT('Ctrl Pts',(5.082734909316,7.331093861617,-8.389443006712));
#44207=CARTESIAN_POINT('Ctrl Pts',(2.107932622538,3.209437931445,-7.974093609674));
#44208=CARTESIAN_POINT('Ctrl Pts',(2.128396203266,3.20832377114,-7.973710572124));
#44209=CARTESIAN_POINT('Ctrl Pts',(2.250984002149,3.202768031486,-7.97144548218));
#44210=CARTESIAN_POINT('Ctrl Pts',(2.470711253402,3.204775266025,-7.967678546612));
#44211=CARTESIAN_POINT('Ctrl Pts',(2.763453159674,3.233567093421,-7.963258313335));
#44212=CARTESIAN_POINT('Ctrl Pts',(3.043704631512,3.285693179689,-7.959557451335));
#44213=CARTESIAN_POINT('Ctrl Pts',(3.314817166296,3.360322787411,-7.956471695572));
#44214=CARTESIAN_POINT('Ctrl Pts',(3.577466067767,3.457049507122,-7.953956646518));
#44215=CARTESIAN_POINT('Ctrl Pts',(3.832382497416,3.5762604501,-7.951986459763));
#44216=CARTESIAN_POINT('Ctrl Pts',(4.079906764865,3.719010073588,-7.950557558931));
#44217=CARTESIAN_POINT('Ctrl Pts',(4.319915478746,3.887014376219,-7.949688993494));
#44218=CARTESIAN_POINT('Ctrl Pts',(4.552916354557,4.083696712316,-7.949423413387));
#44219=CARTESIAN_POINT('Ctrl Pts',(4.780697367817,4.316276202614,-7.949853814381));
#44220=CARTESIAN_POINT('Ctrl Pts',(5.003620995656,4.596243417174,-7.951177111079));
#44221=CARTESIAN_POINT('Ctrl Pts',(5.216642853094,4.937350941106,-7.953731995165));
#44222=CARTESIAN_POINT('Ctrl Pts',(5.406819439974,5.352632881146,-7.958009960562));
#44223=CARTESIAN_POINT('Ctrl Pts',(5.551348297991,5.848391301807,-7.964620728133));
#44224=CARTESIAN_POINT('Ctrl Pts',(5.619772718639,6.412753788441,-7.974098483983));
#44225=CARTESIAN_POINT('Ctrl Pts',(5.590729149136,6.949067622384,-7.985268994065));
#44226=CARTESIAN_POINT('Ctrl Pts',(5.521121943126,7.28486103587,-7.993617512756));
#44227=CARTESIAN_POINT('Ctrl Pts',(5.484197631687,7.420713649103,-7.997235986271));
#44228=CARTESIAN_POINT('Ctrl Pts',(2.097982686268,2.641809757266,-8.001132743794));
#44229=CARTESIAN_POINT('Ctrl Pts',(2.121761001818,2.640657299117,-8.001167370025));
#44230=CARTESIAN_POINT('Ctrl Pts',(2.26420112762,2.63504805256,-8.001379534588));
#44231=CARTESIAN_POINT('Ctrl Pts',(2.519463443997,2.638838702993,-8.001787552801));
#44232=CARTESIAN_POINT('Ctrl Pts',(2.859471577427,2.674089067881,-8.002358257106));
#44233=CARTESIAN_POINT('Ctrl Pts',(3.18492826935,2.736224863315,-8.002904688175));
#44234=CARTESIAN_POINT('Ctrl Pts',(3.499756825995,2.824300917133,-8.003410580015));
#44235=CARTESIAN_POINT('Ctrl Pts',(3.804770782395,2.937849332127,-8.003858188745));
#44236=CARTESIAN_POINT('Ctrl Pts',(4.10084877835,3.077324021872,-8.004231772651));
#44237=CARTESIAN_POINT('Ctrl Pts',(4.388417761842,3.24395206713,-8.004515730234));
#44238=CARTESIAN_POINT('Ctrl Pts',(4.667370373622,3.439727472378,-8.00469383333));
#44239=CARTESIAN_POINT('Ctrl Pts',(4.938340469526,3.668629169678,-8.004749158421));
#44240=CARTESIAN_POINT('Ctrl Pts',(5.203468267774,3.93904415572,-8.004659626021));
#44241=CARTESIAN_POINT('Ctrl Pts',(5.463274621234,4.26431174805,-8.004390090535));
#44242=CARTESIAN_POINT('Ctrl Pts',(5.712047138579,4.660396215544,-8.003894643709));
#44243=CARTESIAN_POINT('Ctrl Pts',(5.934939194387,5.142453440912,-8.003137596628));
#44244=CARTESIAN_POINT('Ctrl Pts',(6.1056490689,5.717890833968,-8.002138506643));
#44245=CARTESIAN_POINT('Ctrl Pts',(6.1888494719,6.37312249819,-8.001050166323));
#44246=CARTESIAN_POINT('Ctrl Pts',(6.159033073884,6.9961590832,-8.000264096742));
#44247=CARTESIAN_POINT('Ctrl Pts',(6.080744158775,7.386544638581,-8.000048758441));
#44248=CARTESIAN_POINT('Ctrl Pts',(6.038895767987,7.544540690767,-8.000015016273));
#44249=CARTESIAN_POINT('',(5.18295248725182,7.29695751098408,-8.53243621599188));
#44250=CARTESIAN_POINT('Ctrl Pts',(5.1829522985385,7.29695750739212,-8.53243627219658));
#44251=CARTESIAN_POINT('Ctrl Pts',(5.18723923406474,7.24664967889388,-8.54361501736799));
#44252=CARTESIAN_POINT('Ctrl Pts',(5.19130154250867,7.19348202716866,-8.55459110489445));
#44253=CARTESIAN_POINT('Ctrl Pts',(5.19490205157409,7.13800448322447,-8.56468063816348));
#44254=CARTESIAN_POINT('Ctrl Pts',(5.19528501692091,7.13210365740475,-8.56575380352356));
#44255=CARTESIAN_POINT('Ctrl Pts',(5.19566273688535,7.12617665834645,-8.56681692760366));
#44256=CARTESIAN_POINT('Ctrl Pts',(5.19603491554704,7.12022412060748,-8.56786918139442));
#44257=CARTESIAN_POINT('Ctrl Pts',(5.19789902987704,7.09040991565347,-8.57313955708245));
#44258=CARTESIAN_POINT('Ctrl Pts',(5.19962419820451,7.05995761975205,-8.57814494571069));
#44259=CARTESIAN_POINT('Ctrl Pts',(5.20121350787315,7.02852136024741,-8.5827781149027));
#44260=CARTESIAN_POINT('Ctrl Pts',(5.20218206777201,7.00936341958488,-8.585601669036));
#44261=CARTESIAN_POINT('Ctrl Pts',(5.20309921267649,6.98983994056404,-8.58828700549728));
#44262=CARTESIAN_POINT('Ctrl Pts',(5.20395612249813,6.96987196846932,-8.59081022277285));
#44263=CARTESIAN_POINT('Ctrl Pts',(5.20461321692097,6.95456015529194,-8.59274507280901));
#44264=CARTESIAN_POINT('Ctrl Pts',(5.20523474535529,6.93898696204747,-8.59458460040998));
#44265=CARTESIAN_POINT('Ctrl Pts',(5.20581397145749,6.92311679382367,-8.59631817378764));
#44266=CARTESIAN_POINT('Ctrl Pts',(5.2077358588334,6.8704591600474,-8.60207021565373));
#44267=CARTESIAN_POINT('Ctrl Pts',(5.20919999246733,6.81452954470778,-8.60664116434144));
#44268=CARTESIAN_POINT('Ctrl Pts',(5.20999840830055,6.75545526215373,-8.60910833131169));
#44269=CARTESIAN_POINT('Ctrl Pts',(5.21026934367702,6.73540892499787,-8.6099455426796));
#44270=CARTESIAN_POINT('Ctrl Pts',(5.21046332268927,6.71500010887712,-8.61054064166149));
#44271=CARTESIAN_POINT('Ctrl Pts',(5.21057211880332,6.69423259999795,-8.61085815377749));
#44272=CARTESIAN_POINT('Ctrl Pts',(5.21076175376346,6.65803419573641,-8.61141158712377));
#44273=CARTESIAN_POINT('Ctrl Pts',(5.21069210583572,6.62074565536196,-8.61111312886292));
#44274=CARTESIAN_POINT('Ctrl Pts',(5.21029733445679,6.58264849326771,-8.60988509567174));
#44275=CARTESIAN_POINT('Ctrl Pts',(5.20991968294653,6.54620347326579,-8.60871031803069));
#44276=CARTESIAN_POINT('Ctrl Pts',(5.2092443421083,6.50901873038902,-8.60668481503895));
#44277=CARTESIAN_POINT('Ctrl Pts',(5.20826147406231,6.47133598480579,-8.60374314939847));
#44278=CARTESIAN_POINT('Ctrl Pts',(5.20794528621798,6.45921347645598,-8.60279681797445));
#44279=CARTESIAN_POINT('Ctrl Pts',(5.20759766387723,6.44703937354788,-8.60175569533908));
#44280=CARTESIAN_POINT('Ctrl Pts',(5.20721943055202,6.43482153224083,-8.60061767598738));
#44281=CARTESIAN_POINT('Ctrl Pts',(5.20717293371244,6.43331957308106,-8.60047777741232));
#44282=CARTESIAN_POINT('Ctrl Pts',(5.20712597375788,6.43181695506658,-8.60033641779852));
#44283=CARTESIAN_POINT('Ctrl Pts',(5.20707854776624,6.43031369019317,-8.60019360443901));
#44284=CARTESIAN_POINT('Ctrl Pts',(5.20577851568142,6.38910648503552,-8.5962788323262));
#44285=CARTESIAN_POINT('Ctrl Pts',(5.20412386978512,6.34741327362881,-8.59127149360352));
#44286=CARTESIAN_POINT('Ctrl Pts',(5.20208863155282,6.30548216541678,-8.58532297130938));
#44287=CARTESIAN_POINT('Ctrl Pts',(5.19996000458014,6.26162701051749,-8.57910149570916));
#44288=CARTESIAN_POINT('Ctrl Pts',(5.19741530186008,6.21751183338102,-8.5718504727011));
#44289=CARTESIAN_POINT('Ctrl Pts',(5.19448099156681,6.17341777707288,-8.56374594101904));
#44290=CARTESIAN_POINT('Ctrl Pts',(5.1941972595391,6.1691541189196,-8.56296227638308));
#44291=CARTESIAN_POINT('Ctrl Pts',(5.19390992441439,6.16489065499327,-8.56217063370893));
#44292=CARTESIAN_POINT('Ctrl Pts',(5.19361903494277,6.16062763730049,-8.56137117349791));
#44293=CARTESIAN_POINT('Ctrl Pts',(5.1889645568448,6.09241574096818,-8.54857913251516));
#44294=CARTESIAN_POINT('Ctrl Pts',(5.18339170218387,6.02431529261517,-8.53380517569397));
#44295=CARTESIAN_POINT('Ctrl Pts',(5.17695209220329,5.95634040206383,-8.51767149052187));
#44296=CARTESIAN_POINT('Ctrl Pts',(5.17573675136541,5.94351157226104,-8.51462659704009));
#44297=CARTESIAN_POINT('Ctrl Pts',(5.17449040621829,5.93068722455044,-8.51153334083738));
#44298=CARTESIAN_POINT('Ctrl Pts',(5.17321317578403,5.91786749114468,-8.50839599056089));
#44299=CARTESIAN_POINT('Ctrl Pts',(5.17212619654791,5.90695733456609,-8.50572596758343));
#44300=CARTESIAN_POINT('Ctrl Pts',(5.17101684657982,5.89605052010649,-8.50302400883112));
#44301=CARTESIAN_POINT('Ctrl Pts',(5.16988525053059,5.88514714324858,-8.50029275191432));
#44302=CARTESIAN_POINT('Ctrl Pts',(5.16230316750045,5.8120907653105,-8.48199239046117));
#44303=CARTESIAN_POINT('Ctrl Pts',(5.15372750951834,5.73919017115096,-8.46237195280239));
#44304=CARTESIAN_POINT('Ctrl Pts',(5.14431889499684,5.66677187873498,-8.44211748739085));
#44305=CARTESIAN_POINT('Ctrl Pts',(5.14193079042821,5.64839059054679,-8.43697647738624));
#44306=CARTESIAN_POINT('Ctrl Pts',(5.13948886442781,5.63004056205971,-8.43179463827499));
#44307=CARTESIAN_POINT('Ctrl Pts',(5.13699536057964,5.61172763420576,-8.42658313372846));
#44308=CARTESIAN_POINT('Ctrl Pts',(5.12949546600836,5.55664649675454,-8.41090810892934));
#44309=CARTESIAN_POINT('Ctrl Pts',(5.12153284902103,5.50190222651919,-8.39496012661076));
#44310=CARTESIAN_POINT('Ctrl Pts',(5.11322560411293,5.44781430353963,-8.37903587164113));
#44311=CARTESIAN_POINT('Ctrl Pts',(5.10788953745503,5.41307152592815,-8.36880710302587));
#44312=CARTESIAN_POINT('Ctrl Pts',(5.10241161165168,5.37860001522318,-8.35858787364834));
#44313=CARTESIAN_POINT('Ctrl Pts',(5.09683002250716,5.34449059744963,-8.34845164351308));
#44314=CARTESIAN_POINT('Ctrl Pts',(5.08797042045967,5.29034905106899,-8.33236250421331));
#44315=CARTESIAN_POINT('Ctrl Pts',(5.07884119105764,5.23711372307129,-8.31649212545848));
#44316=CARTESIAN_POINT('Ctrl Pts',(5.069511669899,5.18459806022679,-8.30092096452761));
#44317=CARTESIAN_POINT('Ctrl Pts',(5.06381317828989,5.152521380301,-8.29141006590805));
#44318=CARTESIAN_POINT('Ctrl Pts',(5.05803892964553,5.12071336580347,-8.28201092988208));
#44319=CARTESIAN_POINT('Ctrl Pts',(5.05219551521658,5.08913373399478,-8.27274283293787));
#44320=CARTESIAN_POINT('Ctrl Pts',(5.04772070181313,5.06495044844973,-8.2656454406624));
#44321=CARTESIAN_POINT('Ctrl Pts',(5.04320144113992,5.04089952986362,-8.25862713571524));
#44322=CARTESIAN_POINT('Ctrl Pts',(5.03863450812376,5.01690204575399,-8.2516724774818));
#44323=CARTESIAN_POINT('Ctrl Pts',(5.03131471129866,4.97843931652748,-8.24052567828929));
#44324=CARTESIAN_POINT('Ctrl Pts',(5.02387456159545,4.94011435349542,-8.22954086069226));
#44325=CARTESIAN_POINT('Ctrl Pts',(5.01627292819204,4.90159183136664,-8.21867609358834));
#44326=CARTESIAN_POINT('Ctrl Pts',(5.01228433768763,4.88137899580684,-8.21297533105433));
#44327=CARTESIAN_POINT('Ctrl Pts',(5.00825063655086,4.86111159023468,-8.20730808233553));
#44328=CARTESIAN_POINT('Ctrl Pts',(5.00416124115483,4.84074012217289,-8.20167162155164));
#44329=CARTESIAN_POINT('Ctrl Pts',(4.99669364977443,4.80354005111777,-8.19137895432589));
#44330=CARTESIAN_POINT('Ctrl Pts',(4.98903930399197,4.76599468914279,-8.18118853798181));
#44331=CARTESIAN_POINT('Ctrl Pts',(4.98117932932182,4.7278550640792,-8.17108846758484));
#44332=CARTESIAN_POINT('Ctrl Pts',(4.97331935465168,4.6897154390156,-8.16098839718786));
#44333=CARTESIAN_POINT('Ctrl Pts',(4.9652543657701,4.65098125419039,-8.15097822975307));
#44334=CARTESIAN_POINT('Ctrl Pts',(4.95693176799035,4.61139297708926,-8.14108593475121));
#44335=CARTESIAN_POINT('Ctrl Pts',(4.95491385635422,4.6017943340777,-8.13868743157702));
#44336=CARTESIAN_POINT('Ctrl Pts',(4.95288061937741,4.5921454452916,-8.13629605936647));
#44337=CARTESIAN_POINT('Ctrl Pts',(4.95083097602889,4.58244253309453,-8.13391261591468));
#44338=CARTESIAN_POINT('Ctrl Pts',(4.94184067356442,4.53988287728865,-8.12345817389968));
#44339=CARTESIAN_POINT('Ctrl Pts',(4.93254499040935,4.49629030101477,-8.11315052694005));
#44340=CARTESIAN_POINT('Ctrl Pts',(4.92297544431639,4.45162169242285,-8.10312070556636));
#44341=CARTESIAN_POINT('Ctrl Pts',(4.91373348375058,4.40848218349251,-8.09343422590291));
#44342=CARTESIAN_POINT('Ctrl Pts',(4.90423648988793,4.36433828423002,-8.08400699033239));
#44343=CARTESIAN_POINT('Ctrl Pts',(4.8944929279702,4.3191572751814,-8.07500141838257));
#44344=CARTESIAN_POINT('Ctrl Pts',(4.89305231704439,4.31247714569442,-8.07366992118948));
#44345=CARTESIAN_POINT('Ctrl Pts',(4.89160627326198,4.30577436841791,-8.07234772096928));
#44346=CARTESIAN_POINT('Ctrl Pts',(4.89015477736819,4.29904886650588,-8.07103542504457));
#44347=CARTESIAN_POINT('Ctrl Pts',(4.88444745348448,4.27260399824501,-8.06587543946994));
#44348=CARTESIAN_POINT('Ctrl Pts',(4.87865286577492,4.24581034509846,-8.0608695711381));
#44349=CARTESIAN_POINT('Ctrl Pts',(4.87278236715416,4.21865081450186,-8.05605112229944));
#44350=CARTESIAN_POINT('Ctrl Pts',(4.86417516312855,4.17883007078203,-8.04898641197064));
#44351=CARTESIAN_POINT('Ctrl Pts',(4.85540597405651,4.13822187706632,-8.04232278026814));
#44352=CARTESIAN_POINT('Ctrl Pts',(4.84649415516862,4.09678027383868,-8.03619910573178));
#44353=CARTESIAN_POINT('Ctrl Pts',(4.83865735079759,4.06033768659553,-8.03081411755181));
#44354=CARTESIAN_POINT('Ctrl Pts',(4.83071011442131,4.02325035891697,-8.0258473682564));
#44355=CARTESIAN_POINT('Ctrl Pts',(4.82264849588103,3.98550100986324,-8.02141843089699));
#44356=CARTESIAN_POINT('Ctrl Pts',(4.81465734732444,3.94808164367814,-8.01702820873377));
#44357=CARTESIAN_POINT('Ctrl Pts',(4.80654432476385,3.91002527144511,-8.01316842437477));
#44358=CARTESIAN_POINT('Ctrl Pts',(4.79835549762466,3.87129242944051,-8.00996662431293));
#44359=CARTESIAN_POINT('Ctrl Pts',(4.79482934650976,3.85461386831123,-8.00858791272628));
#44360=CARTESIAN_POINT('Ctrl Pts',(4.79128883489312,3.83781012371503,-8.00733171078698));
#44361=CARTESIAN_POINT('Ctrl Pts',(4.78773614681455,3.82087945116332,-8.00621041663226));
#44362=CARTESIAN_POINT('Ctrl Pts',(4.77983289626817,3.78321575985821,-8.00371600438864));
#44363=CARTESIAN_POINT('Ctrl Pts',(4.77187114760531,3.74492163519567,-8.0018874550049));
#44364=CARTESIAN_POINT('Ctrl Pts',(4.76385756247949,3.705998673479,-8.0008822568962));
#44365=CARTESIAN_POINT('Ctrl Pts',(4.75925693393927,3.68365285874913,-8.00030516898425));
#44366=CARTESIAN_POINT('Ctrl Pts',(4.75463874402007,3.66110036062685,-7.99999998526946));
#44367=CARTESIAN_POINT('Ctrl Pts',(4.75000019976002,3.63834723186299,-7.99999998599622));
#44368=CARTESIAN_POINT('',(2.169373137679,3.679332757285,-8.863031548225));
#44369=CARTESIAN_POINT('Origin',(2.169373138313,2.688757347123,-9.));
#44370=CARTESIAN_POINT('',(5.13980281059253,6.65770465916531,-8.87505252673587));
#44371=CARTESIAN_POINT('Origin',(2.10038301328526,6.72679850008447,-8.99999817412645));
#44372=CARTESIAN_POINT('Ctrl Pts',(5.18295251264825,7.29695736715025,-8.53243592896757));
#44373=CARTESIAN_POINT('Ctrl Pts',(5.17654833497352,7.1943406645062,-8.58329263403164));
#44374=CARTESIAN_POINT('Ctrl Pts',(5.1699516725902,7.09359920983857,-8.63567789420594));
#44375=CARTESIAN_POINT('Ctrl Pts',(5.157494193214,6.90937313701787,-8.73460493631109));
#44376=CARTESIAN_POINT('Ctrl Pts',(5.15310666387399,6.84592850506508,-8.76944708099986));
#44377=CARTESIAN_POINT('Ctrl Pts',(5.14396640620889,6.71587927969526,-8.84203148010505));
#44378=CARTESIAN_POINT('Ctrl Pts',(5.14187631370327,6.68681172236822,-8.85857429491814));
#44379=CARTESIAN_POINT('Ctrl Pts',(5.13980325342901,6.65769808278058,-8.87503678322028));
#44380=CARTESIAN_POINT('Ctrl Pts',(5.031171575324,8.155237335624,-8.328092758217));
#44381=CARTESIAN_POINT('Ctrl Pts',(5.038708713357,8.115239371898,-8.340486420358));
#44382=CARTESIAN_POINT('Ctrl Pts',(5.055903779581,8.021823545362,-8.369528270796));
#44383=CARTESIAN_POINT('Ctrl Pts',(5.081440156798,7.873580856051,-8.415449976165));
#44384=CARTESIAN_POINT('Ctrl Pts',(5.107114572603,7.709609696431,-8.465029851269));
#44385=CARTESIAN_POINT('Ctrl Pts',(5.130275638286,7.542561037424,-8.513074805866));
#44386=CARTESIAN_POINT('Ctrl Pts',(5.150590806214,7.370633393346,-8.558423192441));
#44387=CARTESIAN_POINT('Ctrl Pts',(5.167866499439,7.188862495842,-8.599955644047));
#44388=CARTESIAN_POINT('Ctrl Pts',(5.181671783386,6.98691179701,-8.635615603358));
#44389=CARTESIAN_POINT('Ctrl Pts',(5.190015050755,6.752775192089,-8.658681825984));
#44390=CARTESIAN_POINT('Ctrl Pts',(5.188780785953,6.485018200615,-8.655143868828));
#44391=CARTESIAN_POINT('Ctrl Pts',(5.174650084459,6.201354130137,-8.616792553242));
#44392=CARTESIAN_POINT('Ctrl Pts',(5.148239374427,5.917872628893,-8.55261185355));
#44393=CARTESIAN_POINT('Ctrl Pts',(5.111611019512,5.639452557662,-8.474210057388));
#44394=CARTESIAN_POINT('Ctrl Pts',(5.067315842323,5.369156561314,-8.390508586803));
#44395=CARTESIAN_POINT('Ctrl Pts',(5.017976873343,5.108292633657,-8.307637532437));
#44396=CARTESIAN_POINT('Ctrl Pts',(4.964741308491,4.85146302315,-8.227986869471));
#44397=CARTESIAN_POINT('Ctrl Pts',(4.906610173435,4.585932850899,-8.151357345673));
#44398=CARTESIAN_POINT('Ctrl Pts',(4.842079312509,4.298108371584,-8.07947238098));
#44399=CARTESIAN_POINT('Ctrl Pts',(4.771105566726,3.978310550728,-8.019756056663));
#44400=CARTESIAN_POINT('Ctrl Pts',(4.721281427315,3.742419916668,-7.998750565229));
#44401=CARTESIAN_POINT('Ctrl Pts',(4.695191509856,3.613080798913,-7.997107751107));
#44402=CARTESIAN_POINT('Ctrl Pts',(4.692661092446,3.600476016323,-7.997045622421));
#44403=CARTESIAN_POINT('Ctrl Pts',(5.313497515126,8.076389263026,-8.153031867848));
#44404=CARTESIAN_POINT('Ctrl Pts',(5.317534510854,8.033660503279,-8.161010743624));
#44405=CARTESIAN_POINT('Ctrl Pts',(5.326265824451,7.934136921648,-8.179935247545));
#44406=CARTESIAN_POINT('Ctrl Pts',(5.337462630015,7.777617310787,-8.210478293268));
#44407=CARTESIAN_POINT('Ctrl Pts',(5.346478990087,7.607149574909,-8.243740345299));
#44408=CARTESIAN_POINT('Ctrl Pts',(5.352349552748,7.437371290181,-8.275637786151));
#44409=CARTESIAN_POINT('Ctrl Pts',(5.355278570525,7.268196900007,-8.304695219039));
#44410=CARTESIAN_POINT('Ctrl Pts',(5.355687020392,7.097302977515,-8.329452046748));
#44411=CARTESIAN_POINT('Ctrl Pts',(5.354195232211,6.91945862717,-8.347946571836));
#44412=CARTESIAN_POINT('Ctrl Pts',(5.352174075495,6.730414811562,-8.357264936963));
#44413=CARTESIAN_POINT('Ctrl Pts',(5.352554332008,6.524883545689,-8.356085858452));
#44414=CARTESIAN_POINT('Ctrl Pts',(5.355545391982,6.28889745216,-8.339458569343));
#44415=CARTESIAN_POINT('Ctrl Pts',(5.355743304285,6.024221707419,-8.302176740217));
#44416=CARTESIAN_POINT('Ctrl Pts',(5.348567768536,5.745007024714,-8.25096946318));
#44417=CARTESIAN_POINT('Ctrl Pts',(5.332271520057,5.462498551095,-8.194966634583));
#44418=CARTESIAN_POINT('Ctrl Pts',(5.307199470508,5.183786132192,-8.140920516122));
#44419=CARTESIAN_POINT('Ctrl Pts',(5.273996300018,4.906787526201,-8.092132289014));
#44420=CARTESIAN_POINT('Ctrl Pts',(5.231834820217,4.620390772582,-8.05003102277));
#44421=CARTESIAN_POINT('Ctrl Pts',(5.178762545894,4.312871161624,-8.018232907273));
#44422=CARTESIAN_POINT('Ctrl Pts',(5.113457189332,3.978364205831,-8.00511529044));
#44423=CARTESIAN_POINT('Ctrl Pts',(5.062572556357,3.740423131644,-8.01837619026));
#44424=CARTESIAN_POINT('Ctrl Pts',(5.034564290784,3.613522785182,-8.03453190803));
#44425=CARTESIAN_POINT('Ctrl Pts',(5.031834968443,3.601189986531,-8.036192956447));
#44426=CARTESIAN_POINT('Ctrl Pts',(5.343715148193,7.936726246008,-7.842947387839));
#44427=CARTESIAN_POINT('Ctrl Pts',(5.341552423568,7.892678299717,-7.8509163253));
#44428=CARTESIAN_POINT('Ctrl Pts',(5.335836718102,7.790705225447,-7.86998804917));
#44429=CARTESIAN_POINT('Ctrl Pts',(5.324457252268,7.632826661304,-7.901227441035));
#44430=CARTESIAN_POINT('Ctrl Pts',(5.309356049496,7.464506176445,-7.935456809141));
#44431=CARTESIAN_POINT('Ctrl Pts',(5.29203668893,7.301307301607,-7.968041021536));
#44432=CARTESIAN_POINT('Ctrl Pts',(5.273219125013,7.14428292257,-7.996958180074));
#44433=CARTESIAN_POINT('Ctrl Pts',(5.253815840562,6.993090308133,-8.020196513283));
#44434=CARTESIAN_POINT('Ctrl Pts',(5.235340681084,6.846770386955,-8.035318131012));
#44435=CARTESIAN_POINT('Ctrl Pts',(5.222346509965,6.707286169975,-8.040470406053));
#44436=CARTESIAN_POINT('Ctrl Pts',(5.224401525058,6.56633478398,-8.040118999002));
#44437=CARTESIAN_POINT('Ctrl Pts',(5.245703537717,6.385473319824,-8.029564849193));
#44438=CARTESIAN_POINT('Ctrl Pts',(5.27671001174,6.153667134501,-7.995362006865));
#44439=CARTESIAN_POINT('Ctrl Pts',(5.307543849893,5.889969376952,-7.943666866687));
#44440=CARTESIAN_POINT('Ctrl Pts',(5.33238773401,5.610077285361,-7.886145647549));
#44441=CARTESIAN_POINT('Ctrl Pts',(5.348757652582,5.324444421342,-7.831644909872));
#44442=CARTESIAN_POINT('Ctrl Pts',(5.356373795317,5.03314145169,-7.7847870628));
#44443=CARTESIAN_POINT('Ctrl Pts',(5.35504567828,4.725491437746,-7.748168605561));
#44444=CARTESIAN_POINT('Ctrl Pts',(5.343331751932,4.389196488746,-7.727282197562));
#44445=CARTESIAN_POINT('Ctrl Pts',(5.319122436767,4.018254298991,-7.733197090829));
#44446=CARTESIAN_POINT('Ctrl Pts',(5.293895775961,3.752329054664,-7.766551305318));
#44447=CARTESIAN_POINT('Ctrl Pts',(5.278459817194,3.610625652574,-7.79561095396));
#44448=CARTESIAN_POINT('Ctrl Pts',(5.276941725209,3.596855779951,-7.798547106358));
#44449=CARTESIAN_POINT('Ctrl Pts',(5.099664136616,7.838671252106,-7.625242200552));
#44450=CARTESIAN_POINT('Ctrl Pts',(5.093148727071,7.795683164535,-7.637613336092));
#44451=CARTESIAN_POINT('Ctrl Pts',(5.077597570703,7.696715214695,-7.666988881474));
#44452=CARTESIAN_POINT('Ctrl Pts',(5.051961619203,7.545392264572,-7.71448895437));
#44453=CARTESIAN_POINT('Ctrl Pts',(5.022970150104,7.386288154655,-7.766261388878));
#44454=CARTESIAN_POINT('Ctrl Pts',(4.993567957957,7.234152663538,-7.815863008815));
#44455=CARTESIAN_POINT('Ctrl Pts',(4.964591406833,7.08976474703,-7.860893443632));
#44456=CARTESIAN_POINT('Ctrl Pts',(4.936960987655,6.952649665104,-7.898984011573));
#44457=CARTESIAN_POINT('Ctrl Pts',(4.912271046082,6.822153566707,-7.926998796839));
#44458=CARTESIAN_POINT('Ctrl Pts',(4.895742416311,6.700350837807,-7.940621984007));
#44459=CARTESIAN_POINT('Ctrl Pts',(4.898304229926,6.578973325192,-7.938960061882));
#44460=CARTESIAN_POINT('Ctrl Pts',(4.925677905901,6.420257064082,-7.914374379919));
#44461=CARTESIAN_POINT('Ctrl Pts',(4.969099180964,6.211279092219,-7.857172641533));
#44462=CARTESIAN_POINT('Ctrl Pts',(5.018624475667,5.968030337843,-7.777665034204));
#44463=CARTESIAN_POINT('Ctrl Pts',(5.067579257769,5.703664743327,-7.690521915594));
#44464=CARTESIAN_POINT('Ctrl Pts',(5.112174401207,5.427114642955,-7.606620402143));
#44465=CARTESIAN_POINT('Ctrl Pts',(5.151461612933,5.137862158608,-7.531345219964));
#44466=CARTESIAN_POINT('Ctrl Pts',(5.185885099729,4.824158450321,-7.467143262251));
#44467=CARTESIAN_POINT('Ctrl Pts',(5.215098814274,4.471110576435,-7.419991233884));
#44468=CARTESIAN_POINT('Ctrl Pts',(5.23727508881,4.068727117922,-7.4034147995));
#44469=CARTESIAN_POINT('Ctrl Pts',(5.245608391033,3.76940638382,-7.427953662365));
#44470=CARTESIAN_POINT('Ctrl Pts',(5.248015394314,3.606514035979,-7.455559442076));
#44471=CARTESIAN_POINT('Ctrl Pts',(5.248230402702,3.590651920927,-7.458387517839));
#44472=CARTESIAN_POINT('',(5.246082198634,7.96024107558274,-8.031111952023));
#44473=CARTESIAN_POINT('Ctrl Pts',(5.246082198634,7.960241075785,-8.031111952023));
#44474=CARTESIAN_POINT('Ctrl Pts',(5.24531416124,7.961564936488,-8.037211072505));
#44475=CARTESIAN_POINT('Ctrl Pts',(5.243746788157,7.960077213467,-8.049657858755));
#44476=CARTESIAN_POINT('Ctrl Pts',(5.241420859859,7.951438324206,-8.068128465827));
#44477=CARTESIAN_POINT('Ctrl Pts',(5.239201509839,7.939491726482,-8.085752715982));
#44478=CARTESIAN_POINT('Ctrl Pts',(5.236885850808,7.924335625739,-8.104141772995));
#44479=CARTESIAN_POINT('Ctrl Pts',(5.234470453135,7.906262887624,-8.123322872162));
#44480=CARTESIAN_POINT('Ctrl Pts',(5.232015563957,7.886079705568,-8.142817580344));
#44481=CARTESIAN_POINT('Ctrl Pts',(5.229553400312,7.864393101416,-8.16237005635));
#44482=CARTESIAN_POINT('Ctrl Pts',(5.226947781756,7.84014329634,-8.183061733116));
#44483=CARTESIAN_POINT('Ctrl Pts',(5.224222732637,7.813560756387,-8.20470182906));
#44484=CARTESIAN_POINT('Ctrl Pts',(5.221362028258,7.784508545691,-8.22741918737));
#44485=CARTESIAN_POINT('Ctrl Pts',(5.218362980801,7.752937676919,-8.251235152442));
#44486=CARTESIAN_POINT('Ctrl Pts',(5.215224251798,7.718786278869,-8.276160353447));
#44487=CARTESIAN_POINT('Ctrl Pts',(5.211941467388,7.681930867577,-8.302229523409));
#44488=CARTESIAN_POINT('Ctrl Pts',(5.208473403288,7.641774422659,-8.329770033749));
#44489=CARTESIAN_POINT('Ctrl Pts',(5.204791140956,7.5977585816,-8.35901152383));
#44490=CARTESIAN_POINT('Ctrl Pts',(5.200873339775,7.549273843232,-8.390123492704));
#44491=CARTESIAN_POINT('Ctrl Pts',(5.196708849019,7.495676152098,-8.423194380345));
#44492=CARTESIAN_POINT('Ctrl Pts',(5.192299032893,7.436264363619,-8.45821376354));
#44493=CARTESIAN_POINT('Ctrl Pts',(5.187673532847,7.370324268216,-8.494944723498));
#44494=CARTESIAN_POINT('Ctrl Pts',(5.184525962137,7.322165181379,-8.51994250699));
#44495=CARTESIAN_POINT('Ctrl Pts',(5.182952650723,7.296957647765,-8.532436450571));
#44496=CARTESIAN_POINT('Origin',(4.69181087540435,7.94978071640467,-7.96462206846104));
#44497=CARTESIAN_POINT('Origin',(4.75,10.48573680623,-7.968642341825));
#44498=CARTESIAN_POINT('',(5.246082198634,10.41979065289,-8.031111952022));
#44499=CARTESIAN_POINT('',(5.246082198634,7.960241075785,-8.031111952023));
#44500=CARTESIAN_POINT('Origin',(4.75,10.41979065293,-7.968642341825));
#44501=CARTESIAN_POINT('Ctrl Pts',(5.24583498938,10.46559780792,-8.030265711223));
#44502=CARTESIAN_POINT('Ctrl Pts',(5.24583498938,10.46530050489,-8.030301692655));
#44503=CARTESIAN_POINT('Ctrl Pts',(5.245834989379,10.46004562112,-8.030931668211));
#44504=CARTESIAN_POINT('Ctrl Pts',(5.245834989331,10.4498027854,-8.03195283292));
#44505=CARTESIAN_POINT('Ctrl Pts',(5.245834989351,10.43481488829,-8.032844402977));
#44506=CARTESIAN_POINT('Ctrl Pts',(5.245834989345,10.42449916127,-8.033050835857));
#44507=CARTESIAN_POINT('Ctrl Pts',(5.245834989346,10.41918940524,-8.033044320572));
#44508=CARTESIAN_POINT('Ctrl Pts',(5.245834989346,10.41888877729,-8.033043589861));
#44509=CARTESIAN_POINT('Ctrl Pts',(5.248664215617,10.46298074913,-8.008641229529));
#44510=CARTESIAN_POINT('Ctrl Pts',(5.248664215617,10.46270014925,-8.008675189523));
#44511=CARTESIAN_POINT('Ctrl Pts',(5.248664215617,10.45774061605,-8.009269768448));
#44512=CARTESIAN_POINT('Ctrl Pts',(5.248664215601,10.44807755293,-8.01023338741));
#44513=CARTESIAN_POINT('Ctrl Pts',(5.248664215608,10.43394801199,-8.011073679399));
#44514=CARTESIAN_POINT('Ctrl Pts',(5.248664215606,10.42422714206,-8.011268221533));
#44515=CARTESIAN_POINT('Ctrl Pts',(5.248664215606,10.41922413839,-8.011262073099));
#44516=CARTESIAN_POINT('Ctrl Pts',(5.248664215606,10.41894087986,-8.011261383974));
#44517=CARTESIAN_POINT('Ctrl Pts',(5.250054025977,10.46034699506,-7.986878796461));
#44518=CARTESIAN_POINT('Ctrl Pts',(5.250054025977,10.46008320489,-7.986910722122));
#44519=CARTESIAN_POINT('Ctrl Pts',(5.250054025977,10.45542090641,-7.987469678606));
#44520=CARTESIAN_POINT('Ctrl Pts',(5.250054025978,10.44634131451,-7.988375384713));
#44521=CARTESIAN_POINT('Ctrl Pts',(5.250054025978,10.43307560553,-7.989164071509));
#44522=CARTESIAN_POINT('Ctrl Pts',(5.250054025978,10.42395338754,-7.989346647043));
#44523=CARTESIAN_POINT('Ctrl Pts',(5.250054025978,10.41925909312,-7.9893408678));
#44524=CARTESIAN_POINT('Ctrl Pts',(5.250054025978,10.41899331481,-7.989340220527));
#44525=CARTESIAN_POINT('Ctrl Pts',(5.249998396461,10.45770796146,-7.965072739197));
#44526=CARTESIAN_POINT('Ctrl Pts',(5.249998396461,10.45746101469,-7.965102626446));
#44527=CARTESIAN_POINT('Ctrl Pts',(5.249998396461,10.45309654676,-7.965625889082));
#44528=CARTESIAN_POINT('Ctrl Pts',(5.249998396461,10.44460159568,-7.966473566244));
#44529=CARTESIAN_POINT('Ctrl Pts',(5.249998396461,10.43220145028,-7.967210544403));
#44530=CARTESIAN_POINT('Ctrl Pts',(5.249998396461,10.42367908425,-7.967381129347));
#44531=CARTESIAN_POINT('Ctrl Pts',(5.249998396461,10.41929411792,-7.967375720036));
#44532=CARTESIAN_POINT('Ctrl Pts',(5.249998396461,10.41904585488,-7.967375114698));
#44533=CARTESIAN_POINT('',(5.24599641608878,10.4645576409889,-8.02912516883275));
#44534=CARTESIAN_POINT('Ctrl Pts',(5.245996542241,10.46455752845,-8.029125198361));
#44535=CARTESIAN_POINT('Ctrl Pts',(5.2460120432,10.4595955694,-8.029591626281));
#44536=CARTESIAN_POINT('Ctrl Pts',(5.246039094108,10.44966467169,-8.030367134869));
#44537=CARTESIAN_POINT('Ctrl Pts',(5.246067839312,10.43474154707,-8.031026583047));
#44538=CARTESIAN_POINT('Ctrl Pts',(5.246078758439,10.424776975,-8.031139333386));
#44539=CARTESIAN_POINT('Ctrl Pts',(5.246082198634,10.41979065289,-8.031111952022));
#44540=CARTESIAN_POINT('Origin',(4.750000004037,10.4571165168,-7.96641902307));
#44541=CARTESIAN_POINT('Origin',(8.197306954564,11.98889246271,39.41676));
#44542=CARTESIAN_POINT('',(4.23,10.15082771808,-16.1));
#44543=CARTESIAN_POINT('',(5.246082198634,10.41979065289,-8.031111952022));
#44544=CARTESIAN_POINT('',(1.218893149689,13.14,-16.1));
#44545=CARTESIAN_POINT('Origin',(1.2063075471585,10.1383337960431,-16.1));
#44546=CARTESIAN_POINT('',(2.23784458253126,13.4097224533938,-8.00832639825692));
#44547=CARTESIAN_POINT('',(2.237844640648,13.40972245349,-8.008326395313));
#44548=CARTESIAN_POINT('',(2.25070091824063,13.4097088030271,-8.00792916996587));
#44549=CARTESIAN_POINT('Ctrl Pts',(2.237844640648,13.4097224534935,-8.00832639531314));
#44550=CARTESIAN_POINT('Ctrl Pts',(2.23927596418,13.4097214685921,-8.00835594235443));
#44551=CARTESIAN_POINT('Ctrl Pts',(2.24070638414192,13.409720288815,-8.00836088798532));
#44552=CARTESIAN_POINT('Ctrl Pts',(2.242134536513,13.4097189970496,-8.00833938734947));
#44553=CARTESIAN_POINT('Ctrl Pts',(2.24356268888409,13.4097177052841,-8.00831788671363));
#44554=CARTESIAN_POINT('Ctrl Pts',(2.24498857359248,13.4097163045634,-8.0082699399031));
#44555=CARTESIAN_POINT('Ctrl Pts',(2.24641625272802,13.4097145733304,-8.00820227825647));
#44556=CARTESIAN_POINT('Ctrl Pts',(2.24784393186355,13.4097128420974,-8.00813461660984));
#44557=CARTESIAN_POINT('Ctrl Pts',(2.24927340557576,13.4097107742197,-8.00804723994156));
#44558=CARTESIAN_POINT('Ctrl Pts',(2.25069783394685,13.4097088006893,-8.00792869483126));
#44559=CARTESIAN_POINT('',(3.726652166637,12.93059538988,-8.835890668796));
#44560=CARTESIAN_POINT('Ctrl Pts',(3.72665216664103,12.9305953898865,-8.83589066879675));
#44561=CARTESIAN_POINT('Ctrl Pts',(3.67915834207035,12.9615640469669,-8.82131895211287));
#44562=CARTESIAN_POINT('Ctrl Pts',(3.62945060498817,12.9922562972525,-8.80384623652916));
#44563=CARTESIAN_POINT('Ctrl Pts',(3.57741786220796,13.0223335068074,-8.78336557823536));
#44564=CARTESIAN_POINT('Ctrl Pts',(3.54859552520211,13.0389940828921,-8.7720207902441));
#44565=CARTESIAN_POINT('Ctrl Pts',(3.51906017611917,13.0554651496962,-8.75975308160159));
#44566=CARTESIAN_POINT('Ctrl Pts',(3.48879640079114,13.0716831311055,-8.74654451168046));
#44567=CARTESIAN_POINT('Ctrl Pts',(3.43564340987221,13.1001671589318,-8.72334598507696));
#44568=CARTESIAN_POINT('Ctrl Pts',(3.38024111998694,13.1278688643674,-8.69724485914804));
#44569=CARTESIAN_POINT('Ctrl Pts',(3.32267013814449,13.1543499903996,-8.6683223432563));
#44570=CARTESIAN_POINT('Ctrl Pts',(3.2882857383413,13.1701659031319,-8.65104830487951));
#44571=CARTESIAN_POINT('Ctrl Pts',(3.2531286892389,13.1855463882986,-8.63276796561064));
#44572=CARTESIAN_POINT('Ctrl Pts',(3.21722500639134,13.2003987422202,-8.61349976246249));
#44573=CARTESIAN_POINT('Ctrl Pts',(3.1662961337491,13.2214665988108,-8.58616808542137));
#44574=CARTESIAN_POINT('Ctrl Pts',(3.1138624144285,13.2414693868998,-8.55684832417649));
#44575=CARTESIAN_POINT('Ctrl Pts',(3.0601161068077,13.260114095891,-8.5257623363328));
#44576=CARTESIAN_POINT('Ctrl Pts',(3.01253212736738,13.276621080065,-8.49824053861466));
#44577=CARTESIAN_POINT('Ctrl Pts',(2.96391993758325,13.2920637610469,-8.46933439956908));
#44578=CARTESIAN_POINT('Ctrl Pts',(2.9144358224046,13.3062639442575,-8.43920159758119));
#44579=CARTESIAN_POINT('Ctrl Pts',(2.86519697669492,13.3203937438433,-8.40921814971057));
#44580=CARTESIAN_POINT('Ctrl Pts',(2.815090644569,13.3332926101047,-8.3780196179234));
#44581=CARTESIAN_POINT('Ctrl Pts',(2.76435866544655,13.3447958777846,-8.34589203270953));
#44582=CARTESIAN_POINT('Ctrl Pts',(2.7140258684057,13.3562086325687,-8.31401724181916));
#44583=CARTESIAN_POINT('Ctrl Pts',(2.66307764286107,13.3662474711529,-8.28122800576709));
#44584=CARTESIAN_POINT('Ctrl Pts',(2.61176745742015,13.3747999263361,-8.24780744521448));
#44585=CARTESIAN_POINT('Ctrl Pts',(2.60411434570424,13.3760755579558,-8.24282263993031));
#44586=CARTESIAN_POINT('Ctrl Pts',(2.59645320634571,13.377318213237,-8.23782379581316));
#44587=CARTESIAN_POINT('Ctrl Pts',(2.5887849046406,13.3785276155587,-8.23281185858658));
#44588=CARTESIAN_POINT('Ctrl Pts',(2.53100835148655,13.3876398153921,-8.19504959143641));
#44589=CARTESIAN_POINT('Ctrl Pts',(2.47282352961947,13.3948688395409,-8.15654399260822));
#44590=CARTESIAN_POINT('Ctrl Pts',(2.41410614342739,13.4001530742437,-8.11740588425265));
#44591=CARTESIAN_POINT('Ctrl Pts',(2.36011830391961,13.4050116763301,-8.08142025802558));
#44592=CARTESIAN_POINT('Ctrl Pts',(2.30567988186774,13.4082256836511,-8.04489985185588));
#44593=CARTESIAN_POINT('Ctrl Pts',(2.25070017668898,13.4097087374959,-8.00793027014345));
#44594=CARTESIAN_POINT('',(4.7344035079452,11.9058908155723,-8.81635043036525));
#44595=CARTESIAN_POINT('Ctrl Pts',(4.73440331546188,11.9058911216399,-8.81635051243198));
#44596=CARTESIAN_POINT('Ctrl Pts',(4.72046359241685,11.9278363177059,-8.82320870877306));
#44597=CARTESIAN_POINT('Ctrl Pts',(4.7062389061123,11.9498000076889,-8.82931631968062));
#44598=CARTESIAN_POINT('Ctrl Pts',(4.69171471142633,11.9717443529647,-8.83473627246239));
#44599=CARTESIAN_POINT('Ctrl Pts',(4.67828510618429,11.99203490268,-8.83974776038744));
#44600=CARTESIAN_POINT('Ctrl Pts',(4.66459968347873,12.0123086348396,-8.84417132437756));
#44601=CARTESIAN_POINT('Ctrl Pts',(4.65066152519305,12.0325405172014,-8.84810350783152));
#44602=CARTESIAN_POINT('Ctrl Pts',(4.64952548577476,12.034189531038,-8.84842400321635));
#44603=CARTESIAN_POINT('Ctrl Pts',(4.64838777480505,12.0358382710313,-8.84874126192524));
#44604=CARTESIAN_POINT('Ctrl Pts',(4.64724839785379,12.0374867260297,-8.8490553512748));
#44605=CARTESIAN_POINT('Ctrl Pts',(4.63345522748258,12.0574427384952,-8.85285768193062));
#44606=CARTESIAN_POINT('Ctrl Pts',(4.61941151381701,12.0773644259773,-8.85619092406822));
#44607=CARTESIAN_POINT('Ctrl Pts',(4.60512837445064,12.0971888001718,-8.85911085637126));
#44608=CARTESIAN_POINT('Ctrl Pts',(4.59086993131378,12.1169788970774,-8.86202573997202));
#44609=CARTESIAN_POINT('Ctrl Pts',(4.57637312672951,12.1366716679523,-8.86452897702727));
#44610=CARTESIAN_POINT('Ctrl Pts',(4.56164792893267,12.1562358343136,-8.86671785975084));
#44611=CARTESIAN_POINT('Ctrl Pts',(4.55878778915275,12.1600358681904,-8.86714301604671));
#44612=CARTESIAN_POINT('Ctrl Pts',(4.5559190227764,12.163831153263,-8.86755643208473));
#44613=CARTESIAN_POINT('Ctrl Pts',(4.55304168486563,12.1676216115795,-8.86795898918841));
#44614=CARTESIAN_POINT('Ctrl Pts',(4.53769059338692,12.1878443571057,-8.87010670041163));
#44615=CARTESIAN_POINT('Ctrl Pts',(4.52209512389882,12.2079306785399,-8.87193658943113));
#44616=CARTESIAN_POINT('Ctrl Pts',(4.50625622100327,12.2278491180283,-8.87351233966313));
#44617=CARTESIAN_POINT('Ctrl Pts',(4.49028964446776,12.2479281153336,-8.87510079164405));
#44618=CARTESIAN_POINT('Ctrl Pts',(4.47407608664396,12.2678366101076,-8.87643124991651));
#44619=CARTESIAN_POINT('Ctrl Pts',(4.45759282280626,12.2875811900474,-8.87759645773072));
#44620=CARTESIAN_POINT('Ctrl Pts',(4.45577719067703,12.2897560562675,-8.87772480541511));
#44621=CARTESIAN_POINT('Ctrl Pts',(4.45395825915881,12.291928970625,-8.87785117276641));
#44622=CARTESIAN_POINT('Ctrl Pts',(4.4521359772108,12.2940999687377,-8.87797570142284));
#44623=CARTESIAN_POINT('Ctrl Pts',(4.43445589041851,12.3151633585722,-8.87918389944961));
#44624=CARTESIAN_POINT('Ctrl Pts',(4.4164667575051,12.3360422242232,-8.8802047942972));
#44625=CARTESIAN_POINT('Ctrl Pts',(4.39819560771196,12.3566931431443,-8.88110001445564));
#44626=CARTESIAN_POINT('Ctrl Pts',(4.3805268560358,12.3766632031807,-8.88196571928834));
#44627=CARTESIAN_POINT('Ctrl Pts',(4.36259376952211,12.3964215516007,-8.8827145160085));
#44628=CARTESIAN_POINT('Ctrl Pts',(4.34438633829058,12.4159560389645,-8.88338663468743));
#44629=CARTESIAN_POINT('Ctrl Pts',(4.32470005956646,12.4370771602303,-8.88411334431939));
#44630=CARTESIAN_POINT('Ctrl Pts',(4.30470347925626,12.4579273790388,-8.88474555950459));
#44631=CARTESIAN_POINT('Ctrl Pts',(4.28442669500039,12.4784916687152,-8.88529467544084));
#44632=CARTESIAN_POINT('Ctrl Pts',(4.26655693998259,12.4966147997795,-8.88577860657772));
#44633=CARTESIAN_POINT('Ctrl Pts',(4.24846816043806,12.5145167582446,-8.88619719033868));
#44634=CARTESIAN_POINT('Ctrl Pts',(4.23017503613097,12.5321747993092,-8.8865275870937));
#44635=CARTESIAN_POINT('Ctrl Pts',(4.21022196148984,12.5514351621353,-8.88688796463247));
#44636=CARTESIAN_POINT('Ctrl Pts',(4.19003223173258,12.5703973128709,-8.88715309162067));
#44637=CARTESIAN_POINT('Ctrl Pts',(4.16959551499735,12.5890931961295,-8.88725343204916));
#44638=CARTESIAN_POINT('Ctrl Pts',(4.15003538727033,12.6069871596876,-8.88734946859078));
#44639=CARTESIAN_POINT('Ctrl Pts',(4.13024816422848,12.6246370788773,-8.88729400526859));
#44640=CARTESIAN_POINT('Ctrl Pts',(4.11025201335401,12.64203511309,-8.88702649602809));
#44641=CARTESIAN_POINT('Ctrl Pts',(4.08980779776577,12.6598229945922,-8.8867529925614));
#44642=CARTESIAN_POINT('Ctrl Pts',(4.06914411961136,12.6773454967263,-8.88626497991193));
#44643=CARTESIAN_POINT('Ctrl Pts',(4.04826969194302,12.694604597329,-8.88544282470021));
#44644=CARTESIAN_POINT('Ctrl Pts',(4.02845058586471,12.7109911517819,-8.88466223413203));
#44645=CARTESIAN_POINT('Ctrl Pts',(4.00844178534803,12.7271396854217,-8.88358014043497));
#44646=CARTESIAN_POINT('Ctrl Pts',(3.9882911131021,12.7430341197216,-8.88212228680299));
#44647=CARTESIAN_POINT('Ctrl Pts',(3.98721813638,12.7438804616107,-8.88204465946668));
#44648=CARTESIAN_POINT('Ctrl Pts',(3.98614476663789,12.744726079807,-8.88196597418561));
#44649=CARTESIAN_POINT('Ctrl Pts',(3.98507101418444,12.7455709708424,-8.88188622231604));
#44650=CARTESIAN_POINT('Ctrl Pts',(3.96573616424763,12.76078475809,-8.88045014603486));
#44651=CARTESIAN_POINT('Ctrl Pts',(3.94626957299195,12.7757655486749,-8.87867191548715));
#44652=CARTESIAN_POINT('Ctrl Pts',(3.92671322249069,12.7904833419625,-8.87644838982425));
#44653=CARTESIAN_POINT('Ctrl Pts',(3.90724135054377,12.8051375580557,-8.87423446923738));
#44654=CARTESIAN_POINT('Ctrl Pts',(3.88768089863728,12.8195308037399,-8.87157880919055));
#44655=CARTESIAN_POINT('Ctrl Pts',(3.86810143765954,12.8336381217342,-8.86842314569923));
#44656=CARTESIAN_POINT('Ctrl Pts',(3.86414329506343,12.8364900274294,-8.86778520341378));
#44657=CARTESIAN_POINT('Ctrl Pts',(3.86018445518521,12.8393302693263,-8.86712697652388));
#44658=CARTESIAN_POINT('Ctrl Pts',(3.8562256065573,12.8421586760638,-8.8664482126833));
#44659=CARTESIAN_POINT('Ctrl Pts',(3.83591435037889,12.8566700906745,-8.86296574908175));
#44660=CARTESIAN_POINT('Ctrl Pts',(3.81559298551218,12.8708755481986,-8.85893634747914));
#44661=CARTESIAN_POINT('Ctrl Pts',(3.79528162573602,12.8847698834918,-8.85425917623451));
#44662=CARTESIAN_POINT('Ctrl Pts',(3.77365563981166,12.8995635114316,-8.84927928120942));
#44663=CARTESIAN_POINT('Ctrl Pts',(3.75204127377548,12.9140042816332,-8.84356550746721));
#44664=CARTESIAN_POINT('Ctrl Pts',(3.73046143290345,12.9281088821324,-8.83704931856408));
#44665=CARTESIAN_POINT('Ctrl Pts',(3.72919155762041,12.9289388735886,-8.83666587054531));
#44666=CARTESIAN_POINT('Ctrl Pts',(3.7279218007954,12.9297677075523,-8.83627965703763));
#44667=CARTESIAN_POINT('Ctrl Pts',(3.72665216663739,12.9305953898806,-8.83589066879607));
#44668=CARTESIAN_POINT('Ctrl Pts',(5.24599603643705,10.464557593822,-8.02912518352156));
#44669=CARTESIAN_POINT('Ctrl Pts',(5.23960886297041,10.5293098253969,-8.0719644400836));
#44670=CARTESIAN_POINT('Ctrl Pts',(5.23114313036524,10.59324216141,-8.11397625912077));
#44671=CARTESIAN_POINT('Ctrl Pts',(5.22071935566554,10.6565502380626,-8.15506706152508));
#44672=CARTESIAN_POINT('Ctrl Pts',(5.2149946266579,10.6913189848239,-8.17763409844285));
#44673=CARTESIAN_POINT('Ctrl Pts',(5.20867842486534,10.7258993816846,-8.19992372898681));
#44674=CARTESIAN_POINT('Ctrl Pts',(5.20178440999674,10.7603234534577,-8.22192239442965));
#44675=CARTESIAN_POINT('Ctrl Pts',(5.19952708631644,10.7715950091284,-8.22912546976175));
#44676=CARTESIAN_POINT('Ctrl Pts',(5.19720777914531,10.782849802605,-8.23629735666203));
#44677=CARTESIAN_POINT('Ctrl Pts',(5.19482671544939,10.7940886657919,-8.24343732543202));
#44678=CARTESIAN_POINT('Ctrl Pts',(5.18426817063287,10.8439260728501,-8.27509867089527));
#44679=CARTESIAN_POINT('Ctrl Pts',(5.17248884820929,10.8934529095174,-8.30614206762962));
#44680=CARTESIAN_POINT('Ctrl Pts',(5.15960538071716,10.9423981591268,-8.33629953697301));
#44681=CARTESIAN_POINT('Ctrl Pts',(5.14750737623479,10.988359376441,-8.36461840373122));
#44682=CARTESIAN_POINT('Ctrl Pts',(5.13443630744655,11.0338077140869,-8.39215581953822));
#44683=CARTESIAN_POINT('Ctrl Pts',(5.12052994224784,11.0785214063487,-8.41872107326711));
#44684=CARTESIAN_POINT('Ctrl Pts',(5.1196270714083,11.0814244430728,-8.4204458225164));
#44685=CARTESIAN_POINT('Ctrl Pts',(5.11872069317206,11.0843243841839,-8.4221664860781));
#44686=CARTESIAN_POINT('Ctrl Pts',(5.11781085086665,11.087221169466,-8.42388301697232));
#44687=CARTESIAN_POINT('Ctrl Pts',(5.11529940807314,11.0952171820476,-8.42862116677971));
#44688=CARTESIAN_POINT('Ctrl Pts',(5.11276156857949,11.1031891491766,-8.43332782524898));
#44689=CARTESIAN_POINT('Ctrl Pts',(5.11019821719763,11.1111358016278,-8.4380018702359));
#44690=CARTESIAN_POINT('Ctrl Pts',(5.09292366871355,11.164688675427,-8.4695004846338));
#44691=CARTESIAN_POINT('Ctrl Pts',(5.07448826746994,11.2170967576868,-8.49951672097186));
#44692=CARTESIAN_POINT('Ctrl Pts',(5.05506589859061,11.268305622478,-8.52793313715213));
#44693=CARTESIAN_POINT('Ctrl Pts',(5.03928099584317,11.3099239727193,-8.55102766123532));
#44694=CARTESIAN_POINT('Ctrl Pts',(5.02284437489363,11.3507503323974,-8.57306654332118));
#44695=CARTESIAN_POINT('Ctrl Pts',(5.00585320087564,11.3907578171497,-8.59401165357297));
#44696=CARTESIAN_POINT('Ctrl Pts',(5.00377937125237,11.3956408644861,-8.59656807433924));
#44697=CARTESIAN_POINT('Ctrl Pts',(5.00169728428527,11.4005117154219,-8.59910822742005));
#44698=CARTESIAN_POINT('Ctrl Pts',(4.99960711231283,11.4053703106247,-8.60163199358955));
#44699=CARTESIAN_POINT('Ctrl Pts',(4.98127182930402,11.4479905922306,-8.62377082598037));
#44700=CARTESIAN_POINT('Ctrl Pts',(4.96231162670814,11.4896666639454,-8.64465675792625));
#44701=CARTESIAN_POINT('Ctrl Pts',(4.94287797767578,11.5302992819331,-8.6642046388798));
#44702=CARTESIAN_POINT('Ctrl Pts',(4.92335358393126,11.5711216324418,-8.68384379794728));
#44703=CARTESIAN_POINT('Ctrl Pts',(4.9033514176432,11.6108907593272,-8.70213236529609));
#44704=CARTESIAN_POINT('Ctrl Pts',(4.88304043862665,11.6495118066644,-8.71903408269427));
#44705=CARTESIAN_POINT('Ctrl Pts',(4.88030099105452,11.6547208285571,-8.72131370538767));
#44706=CARTESIAN_POINT('Ctrl Pts',(4.87755594704801,11.6599089739279,-8.72356817353367));
#44707=CARTESIAN_POINT('Ctrl Pts',(4.87480574064037,11.6650760180154,-8.72579746713904));
#44708=CARTESIAN_POINT('Ctrl Pts',(4.87364799763581,11.6672511671715,-8.72673592363798));
#44709=CARTESIAN_POINT('Ctrl Pts',(4.87248933984689,11.6694225769385,-8.72766991907993));
#44710=CARTESIAN_POINT('Ctrl Pts',(4.8713298016431,11.6715902270508,-8.72859944240856));
#44711=CARTESIAN_POINT('Ctrl Pts',(4.84830268699342,11.7146373017335,-8.7470587223081));
#44712=CARTESIAN_POINT('Ctrl Pts',(4.82492692307448,11.756209583914,-8.76374501041384));
#44713=CARTESIAN_POINT('Ctrl Pts',(4.80134248448596,11.796368798876,-8.77870090903335));
#44714=CARTESIAN_POINT('Ctrl Pts',(4.77918216802678,11.8341030408412,-8.7927537110577));
#44715=CARTESIAN_POINT('Ctrl Pts',(4.75683730732651,11.8705900200991,-8.80528012543115));
#44716=CARTESIAN_POINT('Ctrl Pts',(4.73440350757872,11.9058908193334,-8.81635041762902));
#44717=CARTESIAN_POINT('Ctrl Pts',(5.24405860277,10.41841896918,-8.057679818181));
#44718=CARTESIAN_POINT('Ctrl Pts',(5.235172178155,10.52502830086,-8.128371564553));
#44719=CARTESIAN_POINT('Ctrl Pts',(5.20530028371,10.74104647072,-8.270140627685));
#44720=CARTESIAN_POINT('Ctrl Pts',(5.125913608767,11.05967157546,-8.468059100874));
#44721=CARTESIAN_POINT('Ctrl Pts',(5.016041643698,11.36413136551,-8.639703681194));
#44722=CARTESIAN_POINT('Ctrl Pts',(4.886112276442,11.64063777194,-8.773600837921));
#44723=CARTESIAN_POINT('Ctrl Pts',(4.781666447384,11.8219539015,-8.842625516305));
#44724=CARTESIAN_POINT('Ctrl Pts',(4.725327585499,11.91061577933,-8.869706635872));
#44725=CARTESIAN_POINT('Ctrl Pts',(4.720441050621,11.91824346637,-8.871985319865));
#44726=CARTESIAN_POINT('Ctrl Pts',(5.263405483213,10.56633525831,-7.765984057053));
#44727=CARTESIAN_POINT('Ctrl Pts',(5.24953910387,10.67241634538,-7.836077214095));
#44728=CARTESIAN_POINT('Ctrl Pts',(5.209789346079,10.88490733115,-7.975664007802));
#44729=CARTESIAN_POINT('Ctrl Pts',(5.11802262976,11.19199783826,-8.168244427088));
#44730=CARTESIAN_POINT('Ctrl Pts',(5.000199183344,11.47897625117,-8.333016823614));
#44731=CARTESIAN_POINT('Ctrl Pts',(4.868420870299,11.73341300754,-8.459550995621));
#44732=CARTESIAN_POINT('Ctrl Pts',(4.767730415513,11.89590862948,-8.523574335264));
#44733=CARTESIAN_POINT('Ctrl Pts',(4.715113959745,11.97405300316,-8.548439569164));
#44734=CARTESIAN_POINT('Ctrl Pts',(4.710562374606,11.98076613924,-8.550529537085));
#44735=CARTESIAN_POINT('Ctrl Pts',(5.429303416511,10.70239560335,-7.51838478119));
#44736=CARTESIAN_POINT('Ctrl Pts',(5.410831311191,10.81341375347,-7.588104635239));
#44737=CARTESIAN_POINT('Ctrl Pts',(5.361353134582,11.0336467798,-7.725975081631));
#44738=CARTESIAN_POINT('Ctrl Pts',(5.255448994482,11.34631646014,-7.913862147991));
#44739=CARTESIAN_POINT('Ctrl Pts',(5.12590846242,11.63265782121,-8.072310052117));
#44740=CARTESIAN_POINT('Ctrl Pts',(4.986818578048,11.88078489552,-8.191875405979));
#44741=CARTESIAN_POINT('Ctrl Pts',(4.884846125337,12.03511321985,-8.251040159787));
#44742=CARTESIAN_POINT('Ctrl Pts',(4.833039527478,12.10804408545,-8.273702750527));
#44743=CARTESIAN_POINT('Ctrl Pts',(4.828568893935,12.11429967682,-8.275604699134));
#44744=CARTESIAN_POINT('Ctrl Pts',(5.705336011203,10.79673328632,-7.369232710796));
#44745=CARTESIAN_POINT('Ctrl Pts',(5.683643415344,10.91707006838,-7.438886492236));
#44746=CARTESIAN_POINT('Ctrl Pts',(5.626721757645,11.15461489827,-7.575883270228));
#44747=CARTESIAN_POINT('Ctrl Pts',(5.508026128852,11.48875283381,-7.760751926392));
#44748=CARTESIAN_POINT('Ctrl Pts',(5.365574933928,11.79144130809,-7.914811324028));
#44749=CARTESIAN_POINT('Ctrl Pts',(5.215315821712,12.05040371183,-8.029331757309));
#44750=CARTESIAN_POINT('Ctrl Pts',(5.107305411296,12.20901075874,-8.084847190353));
#44751=CARTESIAN_POINT('Ctrl Pts',(5.053218350566,12.28317653379,-8.105803884447));
#44752=CARTESIAN_POINT('Ctrl Pts',(5.048556900723,12.28953202271,-8.10755978277));
#44753=CARTESIAN_POINT('',(5.0296756656025,12.2439817558929,-8.12864334680508));
#44754=CARTESIAN_POINT('Ctrl Pts',(5.02967626811991,12.2439818882291,-8.1286429048552));
#44755=CARTESIAN_POINT('Ctrl Pts',(5.02967648738242,12.2439809951838,-8.12864293636837));
#44756=CARTESIAN_POINT('Ctrl Pts',(5.02967670664473,12.2439801021382,-8.12864296788131));
#44757=CARTESIAN_POINT('Ctrl Pts',(5.02967692590687,12.2439792090923,-8.128642999394));
#44758=CARTESIAN_POINT('Ctrl Pts',(5.04084945619076,12.1984739392401,-8.13024873303066));
#44759=CARTESIAN_POINT('Ctrl Pts',(5.05153116834038,12.1521715925343,-8.13123707595096));
#44760=CARTESIAN_POINT('Ctrl Pts',(5.06169688000618,12.1054561046381,-8.13168208977979));
#44761=CARTESIAN_POINT('Ctrl Pts',(5.07037995894368,12.0655539037551,-8.13206219993155));
#44762=CARTESIAN_POINT('Ctrl Pts',(5.07868691827156,12.0253495868224,-8.13204747369092));
#44763=CARTESIAN_POINT('Ctrl Pts',(5.08661210601055,11.9850816455577,-8.1317058711365));
#44764=CARTESIAN_POINT('Ctrl Pts',(5.08661217722911,11.9850812836957,-8.13170586806674));
#44765=CARTESIAN_POINT('Ctrl Pts',(5.08661224844763,11.9850809218336,-8.13170586499695));
#44766=CARTESIAN_POINT('Ctrl Pts',(5.08661231966612,11.9850805599716,-8.13170586192714));
#44767=CARTESIAN_POINT('Ctrl Pts',(5.09521421993041,11.9413741985835,-8.13133508399009));
#44768=CARTESIAN_POINT('Ctrl Pts',(5.10337425549314,11.8975974876453,-8.13057930125357));
#44769=CARTESIAN_POINT('Ctrl Pts',(5.11120333789497,11.8532839497436,-8.12948489008677));
#44770=CARTESIAN_POINT('Ctrl Pts',(5.11903242029681,11.8089704118418,-8.12839047891998));
#44771=CARTESIAN_POINT('Ctrl Pts',(5.12653112604953,11.7641199980392,-8.12695640896504));
#44772=CARTESIAN_POINT('Ctrl Pts',(5.13378775745265,11.7182705694087,-8.12518126233682));
#44773=CARTESIAN_POINT('Ctrl Pts',(5.14486231968076,11.6482983850321,-8.12247215797336));
#44774=CARTESIAN_POINT('Ctrl Pts',(5.15535472479294,11.5759944016464,-8.11897642123504));
#44775=CARTESIAN_POINT('Ctrl Pts',(5.16519525578843,11.5013255754757,-8.11473197728622));
#44776=CARTESIAN_POINT('Ctrl Pts',(5.16825083759386,11.4781401694458,-8.11341403563144));
#44777=CARTESIAN_POINT('Ctrl Pts',(5.17124340411837,11.454726808459,-8.11202422654111));
#44778=CARTESIAN_POINT('Ctrl Pts',(5.17417040688738,11.43108476995,-8.11056461713076));
#44779=CARTESIAN_POINT('Ctrl Pts',(5.18231808703616,11.3652741838185,-8.10650161085566));
#44780=CARTESIAN_POINT('Ctrl Pts',(5.18995660706929,11.2976897736154,-8.1018934020723));
#44781=CARTESIAN_POINT('Ctrl Pts',(5.19698873514388,11.2287393237199,-8.09680289807924));
#44782=CARTESIAN_POINT('Ctrl Pts',(5.20061866017442,11.1931476847043,-8.09417522297627));
#44783=CARTESIAN_POINT('Ctrl Pts',(5.20408727345096,11.1571920463045,-8.09141990128149));
#44784=CARTESIAN_POINT('Ctrl Pts',(5.20738320932935,11.1209287096605,-8.08855055885703));
#44785=CARTESIAN_POINT('Ctrl Pts',(5.21389434195574,11.0492903638078,-8.08288216306126));
#44786=CARTESIAN_POINT('Ctrl Pts',(5.21973050537357,10.9764512949221,-8.07676267753496));
#44787=CARTESIAN_POINT('Ctrl Pts',(5.22481639026868,10.9030631605354,-8.07031469790219));
#44788=CARTESIAN_POINT('Ctrl Pts',(5.2272924227007,10.8673345892811,-8.06717553785022));
#44789=CARTESIAN_POINT('Ctrl Pts',(5.2295912026956,10.8314759452762,-8.0639591438049));
#44790=CARTESIAN_POINT('Ctrl Pts',(5.23170748242673,10.7955629743409,-8.06068231933708));
#44791=CARTESIAN_POINT('Ctrl Pts',(5.23678672400019,10.709368955508,-8.05281767704946));
#44792=CARTESIAN_POINT('Ctrl Pts',(5.24081943893851,10.6228631481432,-8.04460206063475));
#44793=CARTESIAN_POINT('Ctrl Pts',(5.24379785372006,10.5358259237703,-8.03611817822594));
#44794=CARTESIAN_POINT('Ctrl Pts',(5.24460940073787,10.5121103552351,-8.03380652253884));
#44795=CARTESIAN_POINT('Ctrl Pts',(5.24534248481075,10.4883555620476,-8.03147495313888));
#44796=CARTESIAN_POINT('Ctrl Pts',(5.24599653617109,10.4645576403199,-8.02912520903265));
#44797=CARTESIAN_POINT('Origin',(5.589034133447,12.40999918796,-8.940774072981));
#44798=CARTESIAN_POINT('Ctrl Pts',(4.987098562407,12.27585194406,-8.14835087597));
#44799=CARTESIAN_POINT('Ctrl Pts',(4.987098562407,12.26694242033,-8.150208671023));
#44800=CARTESIAN_POINT('Ctrl Pts',(4.987098562412,12.17370434769,-8.169454091409));
#44801=CARTESIAN_POINT('Ctrl Pts',(4.987098562457,11.99360631362,-8.202795817883));
#44802=CARTESIAN_POINT('Ctrl Pts',(4.987098562454,11.72908230884,-8.245409589304));
#44803=CARTESIAN_POINT('Ctrl Pts',(4.987098562392,11.44720983869,-8.286072928672));
#44804=CARTESIAN_POINT('Ctrl Pts',(4.987098562673,11.14595693493,-8.325928645102));
#44805=CARTESIAN_POINT('Ctrl Pts',(4.987098561544,10.8306092651,-8.365103658667));
#44806=CARTESIAN_POINT('Ctrl Pts',(4.987098564536,10.60836950429,-8.39178141968));
#44807=CARTESIAN_POINT('Ctrl Pts',(4.987098564583,10.49206836173,-8.405568226311));
#44808=CARTESIAN_POINT('Ctrl Pts',(4.987098564577,10.48360845566,-8.406570214801));
#44809=CARTESIAN_POINT('Ctrl Pts',(5.170465299867,12.25567265706,-8.051672134066));
#44810=CARTESIAN_POINT('Ctrl Pts',(5.170465299867,12.24689977024,-8.05350152513));
#44811=CARTESIAN_POINT('Ctrl Pts',(5.170465299868,12.15505390585,-8.072460052785));
#44812=CARTESIAN_POINT('Ctrl Pts',(5.170465299882,11.97691816161,-8.105445604263));
#44813=CARTESIAN_POINT('Ctrl Pts',(5.170465299881,11.71430579976,-8.147754747855));
#44814=CARTESIAN_POINT('Ctrl Pts',(5.170465299862,11.43376848665,-8.188227714547));
#44815=CARTESIAN_POINT('Ctrl Pts',(5.170465299947,11.13345274852,-8.227960364163));
#44816=CARTESIAN_POINT('Ctrl Pts',(5.170465299605,10.81868443806,-8.267063873485));
#44817=CARTESIAN_POINT('Ctrl Pts',(5.170465300511,10.59665069964,-8.293717021343));
#44818=CARTESIAN_POINT('Ctrl Pts',(5.170465300525,10.48044461194,-8.307492560892));
#44819=CARTESIAN_POINT('Ctrl Pts',(5.170465300523,10.47199157144,-8.308493735951));
#44820=CARTESIAN_POINT('Ctrl Pts',(5.268224992253,12.21809716683,-7.871648373944));
#44821=CARTESIAN_POINT('Ctrl Pts',(5.268224992253,12.20957870917,-7.873424874444));
#44822=CARTESIAN_POINT('Ctrl Pts',(5.268224992253,12.1203252509,-7.891849184266));
#44823=CARTESIAN_POINT('Ctrl Pts',(5.26822499225,11.94584345154,-7.92417150864));
#44824=CARTESIAN_POINT('Ctrl Pts',(5.26822499225,11.6867907259,-7.965913410188));
#44825=CARTESIAN_POINT('Ctrl Pts',(5.268224992254,11.40873958487,-8.006031887316));
#44826=CARTESIAN_POINT('Ctrl Pts',(5.268224992235,11.11016892614,-8.045535376416));
#44827=CARTESIAN_POINT('Ctrl Pts',(5.268224992313,10.79647943042,-8.08450573896));
#44828=CARTESIAN_POINT('Ctrl Pts',(5.268224992105,10.5748293226,-8.111113055102));
#44829=CARTESIAN_POINT('Ctrl Pts',(5.268224992102,10.45880023486,-8.12486761442));
#44830=CARTESIAN_POINT('Ctrl Pts',(5.268224992103,10.45035997864,-8.125867274802));
#44831=CARTESIAN_POINT('Ctrl Pts',(5.2475241072,12.17575325026,-7.668779135705));
#44832=CARTESIAN_POINT('Ctrl Pts',(5.2475241072,12.16752150946,-7.670496033694));
#44833=CARTESIAN_POINT('Ctrl Pts',(5.2475241072,12.08118944034,-7.688318332065));
#44834=CARTESIAN_POINT('Ctrl Pts',(5.2475241072,11.91082528085,-7.71989326411));
#44835=CARTESIAN_POINT('Ctrl Pts',(5.2475241072,11.65578391841,-7.76099593914));
#44836=CARTESIAN_POINT('Ctrl Pts',(5.2475241072,11.38053445109,-7.800714941067));
#44837=CARTESIAN_POINT('Ctrl Pts',(5.247524107202,11.08393032682,-7.839960188592));
#44838=CARTESIAN_POINT('Ctrl Pts',(5.247524107192,10.77145655021,-7.87878050769));
#44839=CARTESIAN_POINT('Ctrl Pts',(5.24752410722,10.55023875671,-7.905336175952));
#44840=CARTESIAN_POINT('Ctrl Pts',(5.24752410722,10.43440913067,-7.919067092593));
#44841=CARTESIAN_POINT('Ctrl Pts',(5.24752410722,10.42598328108,-7.920065046084));
#44842=CARTESIAN_POINT('Origin',(4.749999999929,12.16096907947,-7.722576335477));
#44843=CARTESIAN_POINT('Ctrl Pts',(4.898897183639,12.56298745161,-8.111309650193));
#44844=CARTESIAN_POINT('Ctrl Pts',(4.89889718364,12.554339838,-8.11368287565));
#44845=CARTESIAN_POINT('Ctrl Pts',(4.898897183641,12.52891246354,-8.12068549036));
#44846=CARTESIAN_POINT('Ctrl Pts',(4.89889718364,12.48660188763,-8.132388056127));
#44847=CARTESIAN_POINT('Ctrl Pts',(4.898897183642,12.43566213767,-8.146358919788));
#44848=CARTESIAN_POINT('Ctrl Pts',(4.898897183636,12.3827628083,-8.160506999916));
#44849=CARTESIAN_POINT('Ctrl Pts',(4.89889718366,12.32404545876,-8.175382572088));
#44850=CARTESIAN_POINT('Ctrl Pts',(4.898897183575,12.26901024473,-8.187959846287));
#44851=CARTESIAN_POINT('Ctrl Pts',(4.898897183596,12.23121289109,-8.195258127902));
#44852=CARTESIAN_POINT('Ctrl Pts',(4.898897183619,12.21791966919,-8.197644398133));
#44853=CARTESIAN_POINT('Ctrl Pts',(5.135442534893,12.54345730779,-8.040151306101));
#44854=CARTESIAN_POINT('Ctrl Pts',(5.135442534894,12.53476840202,-8.042535951411));
#44855=CARTESIAN_POINT('Ctrl Pts',(5.135442534894,12.50925370929,-8.04956268475));
#44856=CARTESIAN_POINT('Ctrl Pts',(5.135442534893,12.46696460986,-8.061259268755));
#44857=CARTESIAN_POINT('Ctrl Pts',(5.135442534894,12.41631345353,-8.075150729294));
#44858=CARTESIAN_POINT('Ctrl Pts',(5.135442534892,12.36408597898,-8.089117876537));
#44859=CARTESIAN_POINT('Ctrl Pts',(5.1354425349,12.30667505225,-8.103660339634));
#44860=CARTESIAN_POINT('Ctrl Pts',(5.135442534872,12.2535255264,-8.115798090918));
#44861=CARTESIAN_POINT('Ctrl Pts',(5.135442534879,12.21766329577,-8.122718057467));
#44862=CARTESIAN_POINT('Ctrl Pts',(5.135442534887,12.20513665072,-8.124962380836));
#44863=CARTESIAN_POINT('Ctrl Pts',(5.272152548789,12.48875957496,-7.840859374117));
#44864=CARTESIAN_POINT('Ctrl Pts',(5.272152548789,12.47995502296,-7.843276002811));
#44865=CARTESIAN_POINT('Ctrl Pts',(5.272152548789,12.45419577947,-7.850370284774));
#44866=CARTESIAN_POINT('Ctrl Pts',(5.272152548789,12.41196682884,-7.862050115762));
#44867=CARTESIAN_POINT('Ctrl Pts',(5.272152548789,12.36212393169,-7.875719193362));
#44868=CARTESIAN_POINT('Ctrl Pts',(5.272152548789,12.31177810915,-7.889179605035));
#44869=CARTESIAN_POINT('Ctrl Pts',(5.272152548788,12.25802605798,-7.902789135359));
#44870=CARTESIAN_POINT('Ctrl Pts',(5.272152548793,12.21015774612,-7.91369592249));
#44871=CARTESIAN_POINT('Ctrl Pts',(5.272152548792,12.17971518072,-7.919556348637));
#44872=CARTESIAN_POINT('Ctrl Pts',(5.27215254879,12.16933547408,-7.92140312391));
#44873=CARTESIAN_POINT('Ctrl Pts',(5.24752410724,12.42350167598,-7.603091333436));
#44874=CARTESIAN_POINT('Ctrl Pts',(5.24752410724,12.41455915062,-7.605546120356));
#44875=CARTESIAN_POINT('Ctrl Pts',(5.24752410724,12.38850814241,-7.612720992154));
#44876=CARTESIAN_POINT('Ctrl Pts',(5.24752410724,12.34635095316,-7.624380835719));
#44877=CARTESIAN_POINT('Ctrl Pts',(5.24752410724,12.29747236096,-7.637784596229));
#44878=CARTESIAN_POINT('Ctrl Pts',(5.24752410724,12.24937146982,-7.650640439906));
#44879=CARTESIAN_POINT('Ctrl Pts',(5.24752410724,12.19998469156,-7.663136921674));
#44880=CARTESIAN_POINT('Ctrl Pts',(5.24752410724,12.15841720627,-7.672575089719));
#44881=CARTESIAN_POINT('Ctrl Pts',(5.24752410724,12.13444064867,-7.677171416297));
#44882=CARTESIAN_POINT('Ctrl Pts',(5.24752410724,12.12662237706,-7.678543891224));
#44883=CARTESIAN_POINT('',(4.94560181045734,12.5323463870464,-8.10194138985371));
#44884=CARTESIAN_POINT('Ctrl Pts',(4.94560184643657,12.5323464095504,-8.10194147144728));
#44885=CARTESIAN_POINT('Ctrl Pts',(4.95021211447075,12.5147636855834,-8.10475801671934));
#44886=CARTESIAN_POINT('Ctrl Pts',(4.95491126399553,12.4971660349781,-8.10746710439704));
#44887=CARTESIAN_POINT('Ctrl Pts',(4.95963939106893,12.479691369481,-8.11001463335363));
#44888=CARTESIAN_POINT('Ctrl Pts',(4.96436751814233,12.4622167039839,-8.11256216231023));
#44889=CARTESIAN_POINT('Ctrl Pts',(4.96912560118877,12.4448656279846,-8.11495030211727));
#44890=CARTESIAN_POINT('Ctrl Pts',(4.97403921096105,12.4273482120725,-8.11714242005925));
#44891=CARTESIAN_POINT('Ctrl Pts',(4.97895282073333,12.4098307961603,-8.11933453800122));
#44892=CARTESIAN_POINT('Ctrl Pts',(4.98402319765244,12.3921474782198,-8.1213325009636));
#44893=CARTESIAN_POINT('Ctrl Pts',(4.98939982954737,12.373733426845,-8.12309825180934));
#44894=CARTESIAN_POINT('Ctrl Pts',(4.98939999823955,12.3737328491029,-8.12309830720989));
#44895=CARTESIAN_POINT('Ctrl Pts',(4.98940016693203,12.3737322713602,-8.1230983626102));
#44896=CARTESIAN_POINT('Ctrl Pts',(4.98940033562481,12.3737316936166,-8.12309841801029));
#44897=CARTESIAN_POINT('Ctrl Pts',(4.99267300103294,12.3625233823873,-8.12417318794445));
#44898=CARTESIAN_POINT('Ctrl Pts',(4.99606140290895,12.351040972025,-8.12516300805067));
#44899=CARTESIAN_POINT('Ctrl Pts',(4.99971722500461,12.3389118378633,-8.1260244993316));
#44900=CARTESIAN_POINT('Ctrl Pts',(5.00206681182121,12.331116476662,-8.12657817741093));
#44901=CARTESIAN_POINT('Ctrl Pts',(5.00452676102123,12.3230533869738,-8.12707838512241));
#44902=CARTESIAN_POINT('Ctrl Pts',(5.00713555182364,12.3146157102113,-8.12750524934951));
#44903=CARTESIAN_POINT('Ctrl Pts',(5.00713615243389,12.3146137676427,-8.12750534762456));
#44904=CARTESIAN_POINT('Ctrl Pts',(5.00713675305202,12.3146118250542,-8.12750544589568));
#44905=CARTESIAN_POINT('Ctrl Pts',(5.00713735367803,12.3146098824458,-8.12750554416287));
#44906=CARTESIAN_POINT('Ctrl Pts',(5.01088701655042,12.3024823248453,-8.12811901883954));
#44907=CARTESIAN_POINT('Ctrl Pts',(5.01493909774003,12.2895935841365,-8.12857880355176));
#44908=CARTESIAN_POINT('Ctrl Pts',(5.01923367534567,12.2761717227083,-8.12876405602454));
#44909=CARTESIAN_POINT('Ctrl Pts',(5.022576808797,12.2657234136918,-8.12890826665376));
#44910=CARTESIAN_POINT('Ctrl Pts',(5.02606683982151,12.2549517050472,-8.1288857258758));
#44911=CARTESIAN_POINT('Ctrl Pts',(5.02967477611916,12.2439868176467,-8.12864292461177));
#44912=CARTESIAN_POINT('Ctrl Pts',(5.02967514605934,12.2439856933606,-8.12864289971612));
#44913=CARTESIAN_POINT('Ctrl Pts',(5.02967551600076,12.2439845690726,-8.12864287481815));
#44914=CARTESIAN_POINT('Ctrl Pts',(5.02967588594343,12.2439834447825,-8.12864284991788));
#44915=CARTESIAN_POINT('Origin',(4.75,12.40999995988,-7.658352400433));
#44916=CARTESIAN_POINT('Ctrl Pts',(4.788362511431,11.83313520712,-9.106545692781));
#44917=CARTESIAN_POINT('Ctrl Pts',(4.781336029248,11.84312717048,-9.104679624838));
#44918=CARTESIAN_POINT('Ctrl Pts',(4.734941170835,11.90883089472,-9.091371892558));
#44919=CARTESIAN_POINT('Ctrl Pts',(4.6532235905,12.02218862506,-9.056946451773));
#44920=CARTESIAN_POINT('Ctrl Pts',(4.549498077196,12.16165915061,-9.003256917041));
#44921=CARTESIAN_POINT('Ctrl Pts',(4.447593846191,12.29168835275,-8.957496121759));
#44922=CARTESIAN_POINT('Ctrl Pts',(4.341839766253,12.414305274,-8.932669224563));
#44923=CARTESIAN_POINT('Ctrl Pts',(4.228724956104,12.52955087474,-8.936334256315));
#44924=CARTESIAN_POINT('Ctrl Pts',(4.107910016511,12.63834393914,-8.967414470431));
#44925=CARTESIAN_POINT('Ctrl Pts',(3.979407961331,12.74469289949,-9.016725402368));
#44926=CARTESIAN_POINT('Ctrl Pts',(3.841297009246,12.85384478495,-9.070431947384));
#44927=CARTESIAN_POINT('Ctrl Pts',(3.729267056962,12.9393797692,-9.102292739764));
#44928=CARTESIAN_POINT('Ctrl Pts',(3.664730289745,12.98734865969,-9.113614610693));
#44929=CARTESIAN_POINT('Ctrl Pts',(3.654902747863,12.99461778491,-9.115173463341));
#44930=CARTESIAN_POINT('Ctrl Pts',(4.680427221163,11.86641353654,-8.700123170612));
#44931=CARTESIAN_POINT('Ctrl Pts',(4.676272585031,11.87520161857,-8.697396084167));
#44932=CARTESIAN_POINT('Ctrl Pts',(4.648832174484,11.93327375709,-8.678686998039));
#44933=CARTESIAN_POINT('Ctrl Pts',(4.600262965426,12.03705267819,-8.638017975965));
#44934=CARTESIAN_POINT('Ctrl Pts',(4.533070467253,12.17352591546,-8.581549342235));
#44935=CARTESIAN_POINT('Ctrl Pts',(4.455773084827,12.30711579047,-8.535907121682));
#44936=CARTESIAN_POINT('Ctrl Pts',(4.361227371916,12.43386093394,-8.511743794177));
#44937=CARTESIAN_POINT('Ctrl Pts',(4.248215637988,12.54667493896,-8.515289415159));
#44938=CARTESIAN_POINT('Ctrl Pts',(4.122219669974,12.64113543641,-8.5456642095));
#44939=CARTESIAN_POINT('Ctrl Pts',(3.990318356226,12.71964485498,-8.595335621598));
#44940=CARTESIAN_POINT('Ctrl Pts',(3.856141420295,12.78951953089,-8.653002372258));
#44941=CARTESIAN_POINT('Ctrl Pts',(3.754500915548,12.84053766811,-8.692483554684));
#44942=CARTESIAN_POINT('Ctrl Pts',(3.697931827769,12.86909429444,-8.710053949906));
#44943=CARTESIAN_POINT('Ctrl Pts',(3.689358918034,12.87342214564,-8.712605773735));
#44944=CARTESIAN_POINT('Ctrl Pts',(4.784902130706,12.02281152679,-8.322549113858));
#44945=CARTESIAN_POINT('Ctrl Pts',(4.783249396625,12.0307502655,-8.320163567466));
#44946=CARTESIAN_POINT('Ctrl Pts',(4.772172682196,12.08365258323,-8.304031208104));
#44947=CARTESIAN_POINT('Ctrl Pts',(4.750277919023,12.18357420515,-8.271503273055));
#44948=CARTESIAN_POINT('Ctrl Pts',(4.708455753188,12.32563533914,-8.229059679281));
#44949=CARTESIAN_POINT('Ctrl Pts',(4.64410750416,12.47120052511,-8.195846114845));
#44950=CARTESIAN_POINT('Ctrl Pts',(4.550310030587,12.61049200715,-8.178540175844));
#44951=CARTESIAN_POINT('Ctrl Pts',(4.428613845404,12.73035393126,-8.181069390516));
#44952=CARTESIAN_POINT('Ctrl Pts',(4.289450200103,12.8216762436,-8.202883496443));
#44953=CARTESIAN_POINT('Ctrl Pts',(4.145901869533,12.88451933817,-8.239255237444));
#44954=CARTESIAN_POINT('Ctrl Pts',(4.007076074327,12.92646200883,-8.283117800936));
#44955=CARTESIAN_POINT('Ctrl Pts',(3.909998388249,12.94939041283,-8.315416010061));
#44956=CARTESIAN_POINT('Ctrl Pts',(3.858816430071,12.96108040816,-8.33110977569));
#44957=CARTESIAN_POINT('Ctrl Pts',(3.851123107886,12.96283050514,-8.333428536116));
#44958=CARTESIAN_POINT('Ctrl Pts',(5.065907741302,12.24861789423,-8.103492626421));
#44959=CARTESIAN_POINT('Ctrl Pts',(5.065527744701,12.25635351501,-8.10253388458));
#44960=CARTESIAN_POINT('Ctrl Pts',(5.062604240513,12.30832323267,-8.096071415204));
#44961=CARTESIAN_POINT('Ctrl Pts',(5.051749274438,12.41143376592,-8.083273366865));
#44962=CARTESIAN_POINT('Ctrl Pts',(5.015421902483,12.56574894735,-8.06684237541));
#44963=CARTESIAN_POINT('Ctrl Pts',(4.947917990377,12.72759143794,-8.054099213111));
#44964=CARTESIAN_POINT('Ctrl Pts',(4.844151662906,12.88353862421,-8.047489469458));
#44965=CARTESIAN_POINT('Ctrl Pts',(4.707965973537,13.0175075369,-8.048454343592));
#44966=CARTESIAN_POINT('Ctrl Pts',(4.55217013723,13.11796378328,-8.056792463515));
#44967=CARTESIAN_POINT('Ctrl Pts',(4.392726930966,13.18269400941,-8.070771847542));
#44968=CARTESIAN_POINT('Ctrl Pts',(4.242265944582,13.21764248226,-8.087806560847));
#44969=CARTESIAN_POINT('Ctrl Pts',(4.142357453441,13.22855503805,-8.100585259883));
#44970=CARTESIAN_POINT('Ctrl Pts',(4.092131989576,13.23171649105,-8.106921727197));
#44971=CARTESIAN_POINT('Ctrl Pts',(4.084641136283,13.23213762389,-8.107861429889));
#44972=CARTESIAN_POINT('',(4.07998030874528,13.1991631723816,-8.13213865329994));
#44973=CARTESIAN_POINT('Origin',(4.250000000204,13.7774991556,-8.930023854874));
#44974=CARTESIAN_POINT('',(4.37884053358692,13.1060646994139,-8.10486259615161));
#44975=CARTESIAN_POINT('Ctrl Pts',(4.07998006873709,13.199162565666,-8.13213914414405));
#44976=CARTESIAN_POINT('Ctrl Pts',(4.09485186734027,13.193838138298,-8.1328296702141));
#44977=CARTESIAN_POINT('Ctrl Pts',(4.10974150168657,13.1886223428026,-8.13304462029991));
#44978=CARTESIAN_POINT('Ctrl Pts',(4.12429557597898,13.1836267075159,-8.13289104638594));
#44979=CARTESIAN_POINT('Ctrl Pts',(4.12918128878347,13.1819497036202,-8.13283949257201));
#44980=CARTESIAN_POINT('Ctrl Pts',(4.13402937140421,13.180297908932,-8.13274643888225));
#44981=CARTESIAN_POINT('Ctrl Pts',(4.13882700960573,13.1786767289353,-8.13261589628058));
#44982=CARTESIAN_POINT('Ctrl Pts',(4.14982115159217,13.1749616753359,-8.13231674827529));
#44983=CARTESIAN_POINT('Ctrl Pts',(4.1605547904494,13.1714012335344,-8.13182659094922));
#44984=CARTESIAN_POINT('Ctrl Pts',(4.17127413559097,13.167913595797,-8.13117410839025));
#44985=CARTESIAN_POINT('Ctrl Pts',(4.17916746539731,13.1653454281951,-8.13069364433551));
#44986=CARTESIAN_POINT('Ctrl Pts',(4.18705381055708,13.1628158836012,-8.13012481013473));
#44987=CARTESIAN_POINT('Ctrl Pts',(4.19504044070577,13.1602770806608,-8.1294759888259));
#44988=CARTESIAN_POINT('Ctrl Pts',(4.19541353866471,13.1601584796767,-8.1294456789328));
#44989=CARTESIAN_POINT('Ctrl Pts',(4.1957868479523,13.1600398659674,-8.12941519061416));
#44990=CARTESIAN_POINT('Ctrl Pts',(4.19616036801421,13.1599212399424,-8.12938452432067));
#44991=CARTESIAN_POINT('Ctrl Pts',(4.2146408337908,13.1540520392814,-8.12786726341492));
#44992=CARTESIAN_POINT('Ctrl Pts',(4.23363533465402,13.1481515382724,-8.12591324528158));
#44993=CARTESIAN_POINT('Ctrl Pts',(4.25304057514006,13.1422859855327,-8.12357336709919));
#44994=CARTESIAN_POINT('Ctrl Pts',(4.26970170652261,13.1372498848516,-8.12156437278427));
#44995=CARTESIAN_POINT('Ctrl Pts',(4.28666681876166,13.1322389726019,-8.11927345682789));
#44996=CARTESIAN_POINT('Ctrl Pts',(4.30410507510598,13.1271836418196,-8.11672864605214));
#44997=CARTESIAN_POINT('Ctrl Pts',(4.30738768281662,13.1262320175586,-8.11624960644464));
#44998=CARTESIAN_POINT('Ctrl Pts',(4.31068710664069,13.1252786827765,-8.11576159716865));
#44999=CARTESIAN_POINT('Ctrl Pts',(4.31400453763256,13.1243229759357,-8.11526484703306));
#45000=CARTESIAN_POINT('Ctrl Pts',(4.32243271701589,13.1218949318522,-8.11400281648542));
#45001=CARTESIAN_POINT('Ctrl Pts',(4.3309757891944,13.1194539364639,-8.11268351689281));
#45002=CARTESIAN_POINT('Ctrl Pts',(4.33962681908085,13.1170044688423,-8.11131131639514));
#45003=CARTESIAN_POINT('Ctrl Pts',(4.35247016390373,13.113367981891,-8.10927414343549));
#45004=CARTESIAN_POINT('Ctrl Pts',(4.36555134351534,13.1097126394271,-8.10712032501676));
#45005=CARTESIAN_POINT('Ctrl Pts',(4.37884065455455,13.1060648835415,-8.10486301077009));
#45006=CARTESIAN_POINT('Ctrl Pts',(4.37884065455455,13.1060648835415,-8.10486301077009));
#45007=CARTESIAN_POINT('Ctrl Pts',(4.40088041631503,13.0999932368117,-8.10112911915094));
#45008=CARTESIAN_POINT('Ctrl Pts',(4.42265612898972,13.0929706812728,-8.09778340187562));
#45009=CARTESIAN_POINT('Ctrl Pts',(4.44398948902647,13.0850867284134,-8.09478417341399));
#45010=CARTESIAN_POINT('Ctrl Pts',(4.46147906082444,13.0786232852731,-8.09232533798311));
#45011=CARTESIAN_POINT('Ctrl Pts',(4.4786711993718,13.0715818552625,-8.09009958193691));
#45012=CARTESIAN_POINT('Ctrl Pts',(4.49547706814209,13.0640361851508,-8.08808524355259));
#45013=CARTESIAN_POINT('Ctrl Pts',(4.4979403304374,13.0629302045595,-8.08778999884612));
#45014=CARTESIAN_POINT('Ctrl Pts',(4.50039519708596,13.061813096606,-8.08749945327738));
#45015=CARTESIAN_POINT('Ctrl Pts',(4.50284193021159,13.0606847513753,-8.0872135239302));
#45016=CARTESIAN_POINT('Ctrl Pts',(4.52169287715546,13.0519913733136,-8.08501057057294));
#45017=CARTESIAN_POINT('Ctrl Pts',(4.5400613236599,13.0426349823631,-8.08308024202485));
#45018=CARTESIAN_POINT('Ctrl Pts',(4.55805604718657,13.0325834246664,-8.08138572021557));
#45019=CARTESIAN_POINT('Ctrl Pts',(4.57309759700418,13.0241814614123,-8.07996929199574));
#45020=CARTESIAN_POINT('Ctrl Pts',(4.587878377846,13.0152928662986,-8.0787179159458));
#45021=CARTESIAN_POINT('Ctrl Pts',(4.60245530568187,13.0058732724124,-8.0776191783943));
#45022=CARTESIAN_POINT('Ctrl Pts',(4.62156620056932,12.9935238342681,-8.07617869257368));
#45023=CARTESIAN_POINT('Ctrl Pts',(4.64033533417057,12.9802899205033,-8.07498840147022));
#45024=CARTESIAN_POINT('Ctrl Pts',(4.658580103847,12.9661945309864,-8.07407068066976));
#45025=CARTESIAN_POINT('Ctrl Pts',(4.67306102697751,12.9550069821323,-8.07334228318367));
#45026=CARTESIAN_POINT('Ctrl Pts',(4.68721151853636,12.9432770722533,-8.07278554246642));
#45027=CARTESIAN_POINT('Ctrl Pts',(4.70095515912211,12.9310535381473,-8.0724046213927));
#45028=CARTESIAN_POINT('Ctrl Pts',(4.71548774639111,12.9181283182958,-8.07200183373888));
#45029=CARTESIAN_POINT('Ctrl Pts',(4.72957256114547,12.9046467480563,-8.07179427222516));
#45030=CARTESIAN_POINT('Ctrl Pts',(4.74303440840472,12.8908181191709,-8.07177340722922));
#45031=CARTESIAN_POINT('Ctrl Pts',(4.75646072516754,12.8770259888462,-8.07175259730325));
#45032=CARTESIAN_POINT('Ctrl Pts',(4.76926682763735,12.8628893785513,-8.07191751001232));
#45033=CARTESIAN_POINT('Ctrl Pts',(4.78132056089648,12.8486445744751,-8.0722488014773));
#45034=CARTESIAN_POINT('Ctrl Pts',(4.78301098153662,12.8466468771388,-8.07229526193219));
#45035=CARTESIAN_POINT('Ctrl Pts',(4.7846866790031,12.844647087327,-8.07234497703885));
#45036=CARTESIAN_POINT('Ctrl Pts',(4.78634736250329,12.8426458887586,-8.07239787626646));
#45037=CARTESIAN_POINT('Ctrl Pts',(4.78831507021373,12.8402747121602,-8.07246055540914));
#45038=CARTESIAN_POINT('Ctrl Pts',(4.7902610940703,12.8379010652391,-8.07252802476904));
#45039=CARTESIAN_POINT('Ctrl Pts',(4.79218599750568,12.8355248500579,-8.07260019582179));
#45040=CARTESIAN_POINT('Ctrl Pts',(4.80452002164109,12.8202989977593,-8.07306263954241));
#45041=CARTESIAN_POINT('Ctrl Pts',(4.8159898093593,12.8049711843504,-8.07371690328845));
#45042=CARTESIAN_POINT('Ctrl Pts',(4.82675788022687,12.7895092955398,-8.07454053334698));
#45043=CARTESIAN_POINT('Ctrl Pts',(4.83598106412313,12.7762657122055,-8.07524599782486));
#45044=CARTESIAN_POINT('Ctrl Pts',(4.84468889125999,12.7629226466895,-8.07607603852168));
#45045=CARTESIAN_POINT('Ctrl Pts',(4.8529624584254,12.7494397032225,-8.0770243456723));
#45046=CARTESIAN_POINT('Ctrl Pts',(4.86112597842197,12.7361360971231,-8.07796003933771));
#45047=CARTESIAN_POINT('Ctrl Pts',(4.86885749410308,12.7226987514876,-8.07901338713688));
#45048=CARTESIAN_POINT('Ctrl Pts',(4.87624950212912,12.7089270234116,-8.08021320923806));
#45049=CARTESIAN_POINT('Ctrl Pts',(4.88127004455736,12.6995734695637,-8.08102811064835));
#45050=CARTESIAN_POINT('Ctrl Pts',(4.88613305397369,12.6900652213929,-8.08191086999274));
#45051=CARTESIAN_POINT('Ctrl Pts',(4.89085471528834,12.6803362971401,-8.08287436954563));
#45052=CARTESIAN_POINT('Ctrl Pts',(4.89573634274051,12.6702777646559,-8.0838705116986));
#45053=CARTESIAN_POINT('Ctrl Pts',(4.90046688079482,12.6599832461541,-8.08495295057575));
#45054=CARTESIAN_POINT('Ctrl Pts',(4.90505964902812,12.6493781808306,-8.08613810577501));
#45055=CARTESIAN_POINT('Ctrl Pts',(4.91245225821607,12.6323080611628,-8.08804575466347));
#45056=CARTESIAN_POINT('Ctrl Pts',(4.9195153698735,12.6144440009625,-8.09020459190755));
#45057=CARTESIAN_POINT('Ctrl Pts',(4.92605059631757,12.595935442534,-8.09265778829463));
#45058=CARTESIAN_POINT('Ctrl Pts',(4.93258977518952,12.5774156903477,-8.09511246834594));
#45059=CARTESIAN_POINT('Ctrl Pts',(4.9386000478383,12.558251267161,-8.09786168643568));
#45060=CARTESIAN_POINT('Ctrl Pts',(4.94392696676981,12.5386194520126,-8.10094653022285));
#45061=CARTESIAN_POINT('Ctrl Pts',(4.94449294521136,12.5365335963266,-8.10127429099817));
#45062=CARTESIAN_POINT('Ctrl Pts',(4.94505125356847,12.5344424843935,-8.10160584008563));
#45063=CARTESIAN_POINT('Ctrl Pts',(4.94560173849934,12.5323463420389,-8.10194122666757));
#45064=CARTESIAN_POINT('Ctrl Pts',(4.362160434186,13.06588598318,-8.125550161894));
#45065=CARTESIAN_POINT('Ctrl Pts',(4.369323430001,13.06383284013,-8.124118373749));
#45066=CARTESIAN_POINT('Ctrl Pts',(4.411515161595,13.05105630538,-8.115946316457));
#45067=CARTESIAN_POINT('Ctrl Pts',(4.487401204605,13.02082765928,-8.103918878687));
#45068=CARTESIAN_POINT('Ctrl Pts',(4.584800540606,12.96515873103,-8.093255079523));
#45069=CARTESIAN_POINT('Ctrl Pts',(4.673083800226,12.89664807489,-8.088013558801));
#45070=CARTESIAN_POINT('Ctrl Pts',(4.749096288908,12.81794410941,-8.088006774574));
#45071=CARTESIAN_POINT('Ctrl Pts',(4.811637239583,12.7322492577,-8.092781506338));
#45072=CARTESIAN_POINT('Ctrl Pts',(4.862806047777,12.63865887931,-8.102320087941));
#45073=CARTESIAN_POINT('Ctrl Pts',(4.890937846641,12.56489261123,-8.113320933997));
#45074=CARTESIAN_POINT('Ctrl Pts',(4.903190205307,12.52241499748,-8.121099998878));
#45075=CARTESIAN_POINT('Ctrl Pts',(4.905166983626,12.51516790621,-8.122470492991));
#45076=CARTESIAN_POINT('Ctrl Pts',(4.32819169137,13.30401108901,-8.053821312685));
#45077=CARTESIAN_POINT('Ctrl Pts',(4.339664949579,13.30254401372,-8.052284708458));
#45078=CARTESIAN_POINT('Ctrl Pts',(4.407297404261,13.29255218229,-8.043617185725));
#45079=CARTESIAN_POINT('Ctrl Pts',(4.529416968505,13.26023103414,-8.031694840149));
#45080=CARTESIAN_POINT('Ctrl Pts',(4.685790994072,13.18630244384,-8.021667416542));
#45081=CARTESIAN_POINT('Ctrl Pts',(4.825614762497,13.0860945265,-8.016876941016));
#45082=CARTESIAN_POINT('Ctrl Pts',(4.942633266184,12.96494921969,-8.016866232753));
#45083=CARTESIAN_POINT('Ctrl Pts',(5.034025620724,12.82959125095,-8.02124418716));
#45084=CARTESIAN_POINT('Ctrl Pts',(5.10212953111,12.68003156756,-8.030166647604));
#45085=CARTESIAN_POINT('Ctrl Pts',(5.132448218904,12.5616988631,-8.04102142987));
#45086=CARTESIAN_POINT('Ctrl Pts',(5.142003665006,12.49388627405,-8.049150073241));
#45087=CARTESIAN_POINT('Ctrl Pts',(5.143405454875,12.48232839475,-8.050596112836));
#45088=CARTESIAN_POINT('Ctrl Pts',(4.258497095234,13.43734788581,-7.852905774059));
#45089=CARTESIAN_POINT('Ctrl Pts',(4.273532865299,13.43711178824,-7.850948149822));
#45090=CARTESIAN_POINT('Ctrl Pts',(4.362214226134,13.43371377916,-7.839982893492));
#45091=CARTESIAN_POINT('Ctrl Pts',(4.522777339243,13.40629043844,-7.825554672333));
#45092=CARTESIAN_POINT('Ctrl Pts',(4.728216508237,13.32352445065,-7.813942645311));
#45093=CARTESIAN_POINT('Ctrl Pts',(4.91025077699,13.20090894489,-7.808542095672));
#45094=CARTESIAN_POINT('Ctrl Pts',(5.059442211679,13.04647229783,-7.808526441464));
#45095=CARTESIAN_POINT('Ctrl Pts',(5.17118679781,12.87059606495,-7.813472689643));
#45096=CARTESIAN_POINT('Ctrl Pts',(5.247606559789,12.67474389681,-7.823762479838));
#45097=CARTESIAN_POINT('Ctrl Pts',(5.273659508659,12.51948199623,-7.836833373193));
#45098=CARTESIAN_POINT('Ctrl Pts',(5.276855433658,12.43082409665,-7.847020998172));
#45099=CARTESIAN_POINT('Ctrl Pts',(5.277058326871,12.4157247669,-7.84884462381));
#45100=CARTESIAN_POINT('Ctrl Pts',(4.185096455794,13.40463740749,-7.615110234522));
#45101=CARTESIAN_POINT('Ctrl Pts',(4.201310261247,13.40571164913,-7.612608815703));
#45102=CARTESIAN_POINT('Ctrl Pts',(4.296978205788,13.40968717958,-7.598599206084));
#45103=CARTESIAN_POINT('Ctrl Pts',(4.470532763759,13.39190175455,-7.580205416763));
#45104=CARTESIAN_POINT('Ctrl Pts',(4.692585515909,13.31378080213,-7.565515822195));
#45105=CARTESIAN_POINT('Ctrl Pts',(4.8881074932,13.18834210605,-7.558724365674));
#45106=CARTESIAN_POINT('Ctrl Pts',(5.045857555171,13.02505917063,-7.558705015931));
#45107=CARTESIAN_POINT('Ctrl Pts',(5.160104768517,12.83642484523,-7.564923537623));
#45108=CARTESIAN_POINT('Ctrl Pts',(5.232400577203,12.6252251833,-7.577935915749));
#45109=CARTESIAN_POINT('Ctrl Pts',(5.249694969059,12.45763771892,-7.594566946463));
#45110=CARTESIAN_POINT('Ctrl Pts',(5.245790521177,12.36220114111,-7.607576997605));
#45111=CARTESIAN_POINT('Ctrl Pts',(5.244721418994,12.34595674815,-7.609906775374));
#45112=CARTESIAN_POINT('',(4.25000024490979,13.4099999999935,-7.66332090715394));
#45113=CARTESIAN_POINT('Origin',(4.250000381636,12.90999999997,-7.66332088393));
#45114=CARTESIAN_POINT('Ctrl Pts',(4.25000025238628,13.41,-7.6633209585883));
#45115=CARTESIAN_POINT('Ctrl Pts',(4.28415493337604,13.4099999913798,-7.65835623525745));
#45116=CARTESIAN_POINT('Ctrl Pts',(4.31814697540359,13.4082459767664,-7.65381476712852));
#45117=CARTESIAN_POINT('Ctrl Pts',(4.35172158509816,13.4048129065936,-7.64966299552958));
#45118=CARTESIAN_POINT('Ctrl Pts',(4.38544423063766,13.4013646994631,-7.64549291810304));
#45119=CARTESIAN_POINT('Ctrl Pts',(4.41874511751802,13.3962228787199,-7.6417159812516));
#45120=CARTESIAN_POINT('Ctrl Pts',(4.45138625796055,13.389511906566,-7.63829818044653));
#45121=CARTESIAN_POINT('Ctrl Pts',(4.46161634966191,13.3874086142298,-7.6372270041586));
#45122=CARTESIAN_POINT('Ctrl Pts',(4.47178182289008,13.3851515282507,-7.63619110452606));
#45123=CARTESIAN_POINT('Ctrl Pts',(4.4818759025286,13.3827453756387,-7.63518943471117));
#45124=CARTESIAN_POINT('Ctrl Pts',(4.51075697499333,13.3758609175766,-7.63232346777357));
#45125=CARTESIAN_POINT('Ctrl Pts',(4.53904771285317,13.3677623319655,-7.62973771995563));
#45126=CARTESIAN_POINT('Ctrl Pts',(4.56681852051631,13.3584861754701,-7.6274026746863));
#45127=CARTESIAN_POINT('Ctrl Pts',(4.59478006125459,13.3491463092736,-7.62505159205967));
#45128=CARTESIAN_POINT('Ctrl Pts',(4.62221532564241,13.3386123996553,-7.62295466751495));
#45129=CARTESIAN_POINT('Ctrl Pts',(4.6491849939952,13.3268704055476,-7.621081772125));
#45130=CARTESIAN_POINT('Ctrl Pts',(4.66440127267806,13.3202455760429,-7.62002508511557));
#45131=CARTESIAN_POINT('Ctrl Pts',(4.67946907126468,13.3132352797687,-7.61903971135721));
#45132=CARTESIAN_POINT('Ctrl Pts',(4.69439624426327,13.3058303288484,-7.61812023979166));
#45133=CARTESIAN_POINT('Ctrl Pts',(4.72551027391046,13.2903955333589,-7.61620370371663));
#45134=CARTESIAN_POINT('Ctrl Pts',(4.75599854582717,13.2732465032488,-7.61457349131395));
#45135=CARTESIAN_POINT('Ctrl Pts',(4.78560383747331,13.2544693773512,-7.61323779027849));
#45136=CARTESIAN_POINT('Ctrl Pts',(4.8151597086785,13.2357235963176,-7.61190431894354));
#45137=CARTESIAN_POINT('Ctrl Pts',(4.84383490385939,13.2153554159023,-7.61086437653432));
#45138=CARTESIAN_POINT('Ctrl Pts',(4.87139399083305,13.1934982502575,-7.61012610981066));
#45139=CARTESIAN_POINT('Ctrl Pts',(4.87626049766555,13.1896386141944,-7.60999574337079));
#45140=CARTESIAN_POINT('Ctrl Pts',(4.88109226752965,13.1857326622559,-7.60987478380504));
#45141=CARTESIAN_POINT('Ctrl Pts',(4.88588809340355,13.1817812725556,-7.60976327597167));
#45142=CARTESIAN_POINT('Ctrl Pts',(4.90576650621335,13.1654029974264,-7.60930108263906));
#45143=CARTESIAN_POINT('Ctrl Pts',(4.92503580965707,13.1482315816514,-7.60900127509333));
#45144=CARTESIAN_POINT('Ctrl Pts',(4.9435328183971,13.1304250341334,-7.60885617900091));
#45145=CARTESIAN_POINT('Ctrl Pts',(4.96217990656388,13.1124740093932,-7.60870990564038));
#45146=CARTESIAN_POINT('Ctrl Pts',(4.98004168199111,13.0938779739926,-7.60872086448693));
#45147=CARTESIAN_POINT('Ctrl Pts',(4.99699092323015,13.074834235439,-7.60888119288522));
#45148=CARTESIAN_POINT('Ctrl Pts',(5.01326443784369,13.0565497262225,-7.60903512936508));
#45149=CARTESIAN_POINT('Ctrl Pts',(5.02869681276836,13.0378531896953,-7.6093267627795));
#45150=CARTESIAN_POINT('Ctrl Pts',(5.04321411733002,13.0189428249584,-7.609749133877));
#45151=CARTESIAN_POINT('Ctrl Pts',(5.06060603931925,12.9962879590434,-7.61025514001244));
#45152=CARTESIAN_POINT('Ctrl Pts',(5.07669654126715,12.9733258348404,-7.61094878551759));
#45153=CARTESIAN_POINT('Ctrl Pts',(5.09161639757621,12.9500757718421,-7.61181896630913));
#45154=CARTESIAN_POINT('Ctrl Pts',(5.10693797017169,12.9261997022139,-7.61271257666923));
#45155=CARTESIAN_POINT('Ctrl Pts',(5.12102551994337,12.902019406217,-7.61379235670061));
#45156=CARTESIAN_POINT('Ctrl Pts',(5.13398627545505,12.8775128498845,-7.61504628102299));
#45157=CARTESIAN_POINT('Ctrl Pts',(5.14079582648039,12.8646371617619,-7.61570508996722));
#45158=CARTESIAN_POINT('Ctrl Pts',(5.14729371912646,12.8516707591378,-7.61641197017769));
#45159=CARTESIAN_POINT('Ctrl Pts',(5.15349116847712,12.8386067060649,-7.61716517758683));
#45160=CARTESIAN_POINT('Ctrl Pts',(5.16284753929381,12.8188837332737,-7.61830230472141));
#45161=CARTESIAN_POINT('Ctrl Pts',(5.1715142138442,12.7989569858579,-7.61954502237368));
#45162=CARTESIAN_POINT('Ctrl Pts',(5.17955764954905,12.7786767909224,-7.62092269173428));
#45163=CARTESIAN_POINT('Ctrl Pts',(5.18754921097392,12.758527388418,-7.62229147613468));
#45164=CARTESIAN_POINT('Ctrl Pts',(5.19492576677389,12.7380285473847,-7.62379347717676));
#45165=CARTESIAN_POINT('Ctrl Pts',(5.20170404880516,12.7170169433238,-7.62545749163233));
#45166=CARTESIAN_POINT('Ctrl Pts',(5.20833992004127,12.6964467902424,-7.62708654536765));
#45167=CARTESIAN_POINT('Ctrl Pts',(5.21440256391927,12.6753846636706,-7.6288708762714));
#45168=CARTESIAN_POINT('Ctrl Pts',(5.21985838876017,12.6536692548344,-7.63083750393334));
#45169=CARTESIAN_POINT('Ctrl Pts',(5.22089342463171,12.6495495794844,-7.6312105969551));
#45170=CARTESIAN_POINT('Ctrl Pts',(5.22190647058077,12.6454063817389,-7.63159025095984));
#45171=CARTESIAN_POINT('Ctrl Pts',(5.22289708207348,12.641238551485,-7.63197665043367));
#45172=CARTESIAN_POINT('Ctrl Pts',(5.22930372598955,12.6142836811497,-7.63447563601622));
#45173=CARTESIAN_POINT('Ctrl Pts',(5.23476590910481,12.5863081834297,-7.63725676286129));
#45174=CARTESIAN_POINT('Ctrl Pts',(5.23906231640469,12.5574982517462,-7.64035714954161));
#45175=CARTESIAN_POINT('Ctrl Pts',(5.24327909769855,12.5292222591504,-7.643400076258));
#45176=CARTESIAN_POINT('Ctrl Pts',(5.24637240858335,12.5001429148305,-7.64675053868086));
#45177=CARTESIAN_POINT('Ctrl Pts',(5.24817002368789,12.4704698586976,-7.65044362962145));
#45178=CARTESIAN_POINT('Ctrl Pts',(5.24937639154043,12.4505564629351,-7.65292203902956));
#45179=CARTESIAN_POINT('Ctrl Pts',(5.25000000001406,12.4303763800539,-7.65555475684944));
#45180=CARTESIAN_POINT('Ctrl Pts',(5.25,12.40999999931,-7.658352389464));
#45181=CARTESIAN_POINT('Origin',(4.25,12.41,8.));
#45182=CARTESIAN_POINT('',(4.25,13.41,7.5));
#45183=CARTESIAN_POINT('Origin',(4.25,12.41,7.5));
#45184=CARTESIAN_POINT('',(4.249999999336,13.41,7.5));
#45185=CARTESIAN_POINT('Ctrl Pts',(4.24999999999483,12.91,7.99999999999811));
#45186=CARTESIAN_POINT('Ctrl Pts',(4.75000000031615,12.9099999999981,8.00000000000139));
#45187=CARTESIAN_POINT('Ctrl Pts',(4.74999999999708,12.4099999996768,7.9999999999991));
#45188=CARTESIAN_POINT('Ctrl Pts',(4.24999999999672,13.4100000000044,8.00000000000096));
#45189=CARTESIAN_POINT('Ctrl Pts',(5.25000000063966,13.4100000000007,8.00000000000752));
#45190=CARTESIAN_POINT('Ctrl Pts',(5.25000000000152,12.4099999993577,8.00000000000294));
#45191=CARTESIAN_POINT('Ctrl Pts',(4.25,13.4100000000016,7.49999999999652));
#45192=CARTESIAN_POINT('Ctrl Pts',(5.25000000063778,13.4099999999978,7.50000000000308));
#45193=CARTESIAN_POINT('Ctrl Pts',(5.24999999999965,12.40999999936,7.4999999999985));
#45194=CARTESIAN_POINT('',(4.75,12.41,8.));
#45195=CARTESIAN_POINT('',(4.25,12.91,8.));
#45196=CARTESIAN_POINT('Origin',(4.25,12.41,8.));
#45197=CARTESIAN_POINT('Origin',(4.75,12.41,7.5));
#45198=CARTESIAN_POINT('Origin',(4.25,12.91,7.5));
#45199=CARTESIAN_POINT('Origin',(-4.6,13.41,8.));
#45200=CARTESIAN_POINT('',(4.75,1.410000000002,8.));
#45201=CARTESIAN_POINT('',(-1.6,12.91,8.));
#45202=CARTESIAN_POINT('',(4.25,12.91,8.));
#45203=CARTESIAN_POINT('',(-4.1,10.41,8.));
#45204=CARTESIAN_POINT('Origin',(-1.6,10.41,8.));
#45205=CARTESIAN_POINT('',(-4.1,10.41,8.));
#45206=CARTESIAN_POINT('',(-4.40872847693047E-16,12.51,8.));
#45207=CARTESIAN_POINT('Origin',(0.,8.91,8.));
#45208=CARTESIAN_POINT('Origin',(0.,8.91,8.));
#45209=CARTESIAN_POINT('',(-4.40872847693047E-16,12.51,7.));
#45210=CARTESIAN_POINT('Origin',(0.,8.91,7.));
#45211=CARTESIAN_POINT('',(-4.40872847693047E-16,12.51,8.));
#45212=CARTESIAN_POINT('Origin',(-4.6,0.,7.));
#45213=CARTESIAN_POINT('',(0.,5.68,7.));
#45214=CARTESIAN_POINT('Origin',(0.,8.91,7.));
#45215=CARTESIAN_POINT('Origin',(0.,8.91,8.));
#45216=CARTESIAN_POINT('',(0.,5.68,-16.1));
#45217=CARTESIAN_POINT('Origin',(0.,8.91,-16.1));
#45218=CARTESIAN_POINT('',(3.95560916124595E-16,5.68,8.));
#45219=CARTESIAN_POINT('',(3.95560916124595E-16,5.68,8.));
#45220=CARTESIAN_POINT('Origin',(-4.6,0.,-16.1));
#45221=CARTESIAN_POINT('',(1.258051184494,4.68,-16.1));
#45222=CARTESIAN_POINT('',(4.23,7.656716133874,-16.1));
#45223=CARTESIAN_POINT('Origin',(1.2063075471551,7.70854277345064,-16.1));
#45224=CARTESIAN_POINT('',(-1.245641523513,4.68,-16.1));
#45225=CARTESIAN_POINT('',(1.258051184494,4.68,-16.1));
#45226=CARTESIAN_POINT('',(-4.23,7.689614180046,-16.1));
#45227=CARTESIAN_POINT('Origin',(-1.22687177271412,7.70854277344467,-16.1));
#45228=CARTESIAN_POINT('',(-4.23,10.14289693909,-16.1));
#45229=CARTESIAN_POINT('',(-4.23,10.14289693909,-16.1));
#45230=CARTESIAN_POINT('',(-1.231437138339,13.14,-16.1));
#45231=CARTESIAN_POINT('Origin',(-1.22687177271438,10.1383337960394,-16.1));
#45232=CARTESIAN_POINT('',(1.218893149689,13.14,-16.1));
#45233=CARTESIAN_POINT('',(4.23,10.15082771808,-16.1));
#45234=CARTESIAN_POINT('Origin',(-2.749877045436,12.05258860061,-47.51676));
#45235=CARTESIAN_POINT('',(1.258051184494,4.68,-16.1));
#45236=CARTESIAN_POINT('',(4.23,7.656716133874,-16.1));
#45237=CARTESIAN_POINT('Origin',(4.23,0.,-16.1));
#45238=CARTESIAN_POINT('Origin',(-4.6,3.56,-8.));
#45239=CARTESIAN_POINT('',(-1.576219094763,3.679332757285,-8.863031548225));
#45240=CARTESIAN_POINT('',(-1.576219094763,3.679332757285,-8.863031548225));
#45241=CARTESIAN_POINT('',(-1.576219094763,3.679332757285,-8.863031548225));
#45242=CARTESIAN_POINT('Origin',(-1.673987770644,2.688757347123,-9.));
#45243=CARTESIAN_POINT('Origin',(-1.576219094767,2.688757347123,-9.));
#45244=CARTESIAN_POINT('Ctrl Pts',(-4.555013514898,6.748954102442,-9.006265058719));
#45245=CARTESIAN_POINT('Ctrl Pts',(-4.556447823076,6.654112126016,-9.001984393795));
#45246=CARTESIAN_POINT('Ctrl Pts',(-4.549028255214,6.413451891621,-8.991281013082));
#45247=CARTESIAN_POINT('Ctrl Pts',(-4.494420707384,6.046862385281,-8.975598452435));
#45248=CARTESIAN_POINT('Ctrl Pts',(-4.385548769305,5.671570029758,-8.960309855565));
#45249=CARTESIAN_POINT('Ctrl Pts',(-4.249041101692,5.351127072694,-8.947889723381));
#45250=CARTESIAN_POINT('Ctrl Pts',(-4.095807849191,5.077797340177,-8.937834704605));
#45251=CARTESIAN_POINT('Ctrl Pts',(-3.93137473704,4.842250471115,-8.929646446674));
#45252=CARTESIAN_POINT('Ctrl Pts',(-3.75682360245,4.635573614044,-8.922909486779));
#45253=CARTESIAN_POINT('Ctrl Pts',(-3.571393820409,4.451722491939,-8.917364128898));
#45254=CARTESIAN_POINT('Ctrl Pts',(-3.374685391696,4.287862755454,-8.912889712537));
#45255=CARTESIAN_POINT('Ctrl Pts',(-3.166908514,4.14295750472,-8.909437356023));
#45256=CARTESIAN_POINT('Ctrl Pts',(-2.947784283048,4.016392071403,-8.906984289856));
#45257=CARTESIAN_POINT('Ctrl Pts',(-2.716575401331,3.908084602248,-8.905538460177));
#45258=CARTESIAN_POINT('Ctrl Pts',(-2.470263032896,3.817877379428,-8.905138263878));
#45259=CARTESIAN_POINT('Ctrl Pts',(-2.202177792142,3.746305952892,-8.905907855567));
#45260=CARTESIAN_POINT('Ctrl Pts',(-1.902141250127,3.696680270292,-8.908149149792));
#45261=CARTESIAN_POINT('Ctrl Pts',(-1.673459288454,3.683895992251,-8.91099064003));
#45262=CARTESIAN_POINT('Ctrl Pts',(-1.544864774431,3.685086791525,-8.912967262473));
#45263=CARTESIAN_POINT('Ctrl Pts',(-1.529192023974,3.685356654255,-8.913213783927));
#45264=CARTESIAN_POINT('Ctrl Pts',(-4.551445835519,6.748899079632,-8.43676403776));
#45265=CARTESIAN_POINT('Ctrl Pts',(-4.555316030739,6.654204804538,-8.432468577285));
#45266=CARTESIAN_POINT('Ctrl Pts',(-4.554009041628,6.413344898856,-8.421763232492));
#45267=CARTESIAN_POINT('Ctrl Pts',(-4.50813646724,6.044315347024,-8.406227812707));
#45268=CARTESIAN_POINT('Ctrl Pts',(-4.406998304746,5.664250402887,-8.39122687889));
#45269=CARTESIAN_POINT('Ctrl Pts',(-4.275820969953,5.338196002922,-8.379138040623));
#45270=CARTESIAN_POINT('Ctrl Pts',(-4.125918859847,5.059063976121,-8.369414768897));
#45271=CARTESIAN_POINT('Ctrl Pts',(-3.963230034915,4.81785346704,-8.361538711491));
#45272=CARTESIAN_POINT('Ctrl Pts',(-3.789148076767,4.605778526808,-8.355086998769));
#45273=CARTESIAN_POINT('Ctrl Pts',(-3.603102197143,4.416865877513,-8.349795833183));
#45274=CARTESIAN_POINT('Ctrl Pts',(-3.404816945335,4.248374826253,-8.34553936651));
#45275=CARTESIAN_POINT('Ctrl Pts',(-3.194612641259,4.099379337421,-8.342263036106));
#45276=CARTESIAN_POINT('Ctrl Pts',(-2.972311875782,3.969365921545,-8.339939216805));
#45277=CARTESIAN_POINT('Ctrl Pts',(-2.7372726709,3.858355006536,-8.338571196862));
#45278=CARTESIAN_POINT('Ctrl Pts',(-2.486539606334,3.766286063129,-8.338192764716));
#45279=CARTESIAN_POINT('Ctrl Pts',(-2.213451223554,3.693832607777,-8.338920550267));
#45280=CARTESIAN_POINT('Ctrl Pts',(-1.907815402646,3.644575726475,-8.341042072484));
#45281=CARTESIAN_POINT('Ctrl Pts',(-1.675073037896,3.633188818873,-8.343736117257));
#45282=CARTESIAN_POINT('Ctrl Pts',(-1.544341556226,3.635522541957,-8.34561460226));
#45283=CARTESIAN_POINT('Ctrl Pts',(-1.528410670948,3.635936933942,-8.345849180363));
#45284=CARTESIAN_POINT('Ctrl Pts',(-4.944357460806,6.754958137238,-8.02454051063));
#45285=CARTESIAN_POINT('Ctrl Pts',(-4.950178879718,6.648164231245,-8.021927553065));
#45286=CARTESIAN_POINT('Ctrl Pts',(-4.952314090325,6.376150039691,-8.015454344926));
#45287=CARTESIAN_POINT('Ctrl Pts',(-4.905540054373,5.957982614761,-8.006227774445));
#45288=CARTESIAN_POINT('Ctrl Pts',(-4.79557736435,5.525814961368,-7.997480967033));
#45289=CARTESIAN_POINT('Ctrl Pts',(-4.650154913714,5.154049620586,-7.990543071787));
#45290=CARTESIAN_POINT('Ctrl Pts',(-4.482325211086,4.835109890624,-7.985035586605));
#45291=CARTESIAN_POINT('Ctrl Pts',(-4.29905970525,4.559051487263,-7.980622885206));
#45292=CARTESIAN_POINT('Ctrl Pts',(-4.102123502363,4.316038923001,-7.977041098496));
#45293=CARTESIAN_POINT('Ctrl Pts',(-3.890984442267,4.099374026924,-7.974126196536));
#45294=CARTESIAN_POINT('Ctrl Pts',(-3.665406689107,3.90602233631,-7.97179632394));
#45295=CARTESIAN_POINT('Ctrl Pts',(-3.425821445495,3.735009363527,-7.970012165066));
#45296=CARTESIAN_POINT('Ctrl Pts',(-3.172091618693,3.585819602461,-7.968751607297));
#45297=CARTESIAN_POINT('Ctrl Pts',(-2.9035510228,3.458540431353,-7.968011444657));
#45298=CARTESIAN_POINT('Ctrl Pts',(-2.616895030684,3.353162131553,-7.967806962617));
#45299=CARTESIAN_POINT('Ctrl Pts',(-2.304590451932,3.270525568452,-7.968200269829));
#45300=CARTESIAN_POINT('Ctrl Pts',(-1.955097738855,3.214834608574,-7.96934911048));
#45301=CARTESIAN_POINT('Ctrl Pts',(-1.689114387761,3.202622899529,-7.97081316528));
#45302=CARTESIAN_POINT('Ctrl Pts',(-1.539811653485,3.205845373877,-7.971839221048));
#45303=CARTESIAN_POINT('Ctrl Pts',(-1.521619260623,3.206388153424,-7.971967698541));
#45304=CARTESIAN_POINT('Ctrl Pts',(-5.513310479943,6.763731920509,-8.00086707723));
#45305=CARTESIAN_POINT('Ctrl Pts',(-5.519503750751,6.639379390508,-8.000689974857));
#45306=CARTESIAN_POINT('Ctrl Pts',(-5.520479581067,6.322735001717,-8.000308619381));
#45307=CARTESIAN_POINT('Ctrl Pts',(-5.463673401723,5.836300034902,-8.00001310954));
#45308=CARTESIAN_POINT('Ctrl Pts',(-5.333278766416,5.333931092847,-7.999978096344));
#45309=CARTESIAN_POINT('Ctrl Pts',(-5.162027786566,4.902000836767,-8.000120924242));
#45310=CARTESIAN_POINT('Ctrl Pts',(-4.965069797,4.531581584195,-8.000348053384));
#45311=CARTESIAN_POINT('Ctrl Pts',(-4.750450918913,4.211041986036,-8.000606793039));
#45312=CARTESIAN_POINT('Ctrl Pts',(-4.520159124177,3.928909404814,-8.000869476857));
#45313=CARTESIAN_POINT('Ctrl Pts',(-4.273528000303,3.6773715762,-8.001119738332));
#45314=CARTESIAN_POINT('Ctrl Pts',(-4.010254167232,3.452877657092,-8.001344213877));
#45315=CARTESIAN_POINT('Ctrl Pts',(-3.730818261462,3.25427257492,-8.001531208702));
#45316=CARTESIAN_POINT('Ctrl Pts',(-3.435039708917,3.080936742835,-8.001671398203));
#45317=CARTESIAN_POINT('Ctrl Pts',(-3.122122169926,2.932951596962,-8.001756889332));
#45318=CARTESIAN_POINT('Ctrl Pts',(-2.788195105891,2.810283344696,-8.001780950925));
#45319=CARTESIAN_POINT('Ctrl Pts',(-2.424463009301,2.713875693873,-8.001734762281));
#45320=CARTESIAN_POINT('Ctrl Pts',(-2.017461124553,2.648557530889,-8.001603722034));
#45321=CARTESIAN_POINT('Ctrl Pts',(-1.707705622985,2.633761592545,-8.001445312088));
#45322=CARTESIAN_POINT('Ctrl Pts',(-1.533816508689,2.637120023378,-8.001342891059));
#45323=CARTESIAN_POINT('Ctrl Pts',(-1.512628024633,2.637703018638,-8.001330637038));
#45324=CARTESIAN_POINT('',(-4.56872735814743,6.21817739199662,-8.68455045311303));
#45325=CARTESIAN_POINT('Ctrl Pts',(-4.09999994889581,3.59647863419517,-7.9999999943637));
#45326=CARTESIAN_POINT('Ctrl Pts',(-4.10784885595024,3.63493711424939,-7.99999999507475));
#45327=CARTESIAN_POINT('Ctrl Pts',(-4.11563766356533,3.67273218799167,-8.00090976440895));
#45328=CARTESIAN_POINT('Ctrl Pts',(-4.12336776546972,3.7098404370961,-8.0025577781243));
#45329=CARTESIAN_POINT('Ctrl Pts',(-4.13082795095019,3.74565295607691,-8.00414824719481));
#45330=CARTESIAN_POINT('Ctrl Pts',(-4.13823314028214,3.78082671080731,-8.00642597730379));
#45331=CARTESIAN_POINT('Ctrl Pts',(-4.14556120029949,3.81537188993273,-8.00926132268278));
#45332=CARTESIAN_POINT('Ctrl Pts',(-4.14961303631167,3.83447263426291,-8.01082904381039));
#45333=CARTESIAN_POINT('Ctrl Pts',(-4.1536408997682,3.85338168668975,-8.01256771249665));
#45334=CARTESIAN_POINT('Ctrl Pts',(-4.15763848499059,3.87210352808029,-8.01445918360056));
#45335=CARTESIAN_POINT('Ctrl Pts',(-4.16604335298257,3.91146594231295,-8.01843597560237));
#45336=CARTESIAN_POINT('Ctrl Pts',(-4.1743216333607,3.94998873082823,-8.02308440620833));
#45337=CARTESIAN_POINT('Ctrl Pts',(-4.18247881285424,3.98770631964574,-8.02824998531657));
#45338=CARTESIAN_POINT('Ctrl Pts',(-4.1909009272832,4.02664892833259,-8.0335833359405));
#45339=CARTESIAN_POINT('Ctrl Pts',(-4.1991936928912,4.06473395988767,-8.03946758096497));
#45340=CARTESIAN_POINT('Ctrl Pts',(-4.20733446973179,4.10202191456589,-8.04577395397839));
#45341=CARTESIAN_POINT('Ctrl Pts',(-4.20886954901462,4.10905318048147,-8.04696312581693));
#45342=CARTESIAN_POINT('Ctrl Pts',(-4.21039915134647,4.1160561479542,-8.04816743038948));
#45343=CARTESIAN_POINT('Ctrl Pts',(-4.21192302832599,4.12303127501757,-8.04938617576649));
#45344=CARTESIAN_POINT('Ctrl Pts',(-4.21726041505002,4.14746169235889,-8.05365483753029));
#45345=CARTESIAN_POINT('Ctrl Pts',(-4.22253071088453,4.17154825128124,-8.05809915532785));
#45346=CARTESIAN_POINT('Ctrl Pts',(-4.22773274177579,4.19529368186173,-8.06268543417868));
#45347=CARTESIAN_POINT('Ctrl Pts',(-4.23698174367817,4.2375121033211,-8.07083965369463));
#45348=CARTESIAN_POINT('Ctrl Pts',(-4.24601616520686,4.27865162459762,-8.07943996562046));
#45349=CARTESIAN_POINT('Ctrl Pts',(-4.25481156728255,4.31874039069041,-8.08833311795105));
#45350=CARTESIAN_POINT('Ctrl Pts',(-4.25722631479631,4.32974662410862,-8.09077470246248));
#45351=CARTESIAN_POINT('Ctrl Pts',(-4.2596229178289,4.34067372356152,-8.0932386297565));
#45352=CARTESIAN_POINT('Ctrl Pts',(-4.26200060082954,4.35152238842346,-8.09572233653976));
#45353=CARTESIAN_POINT('Ctrl Pts',(-4.27113966826723,4.39322125229864,-8.10526892613202));
#45354=CARTESIAN_POINT('Ctrl Pts',(-4.2800021224755,4.43375752535204,-8.11510280598522));
#45355=CARTESIAN_POINT('Ctrl Pts',(-4.28859717867311,4.47321716789487,-8.12509676633268));
#45356=CARTESIAN_POINT('Ctrl Pts',(-4.29404107442491,4.49820992832222,-8.13142669333121));
#45357=CARTESIAN_POINT('Ctrl Pts',(-4.29937709674632,4.5227709357553,-8.13782181610565));
#45358=CARTESIAN_POINT('Ctrl Pts',(-4.3046026461297,4.54692215970033,-8.14425930542139));
#45359=CARTESIAN_POINT('Ctrl Pts',(-4.30548872710659,4.55101741142147,-8.14535089147351));
#45360=CARTESIAN_POINT('Ctrl Pts',(-4.30637162427403,4.55510087926121,-8.14644371200622));
#45361=CARTESIAN_POINT('Ctrl Pts',(-4.30725131830165,4.5591726673425,-8.14753767543186));
#45362=CARTESIAN_POINT('Ctrl Pts',(-4.31619737143733,4.60058073809078,-8.15866274236079));
#45363=CARTESIAN_POINT('Ctrl Pts',(-4.32481660242633,4.64077948467494,-8.16990037622455));
#45364=CARTESIAN_POINT('Ctrl Pts',(-4.33313053238231,4.67989643024333,-8.18116017355279));
#45365=CARTESIAN_POINT('Ctrl Pts',(-4.33806753938206,4.70312499183843,-8.18784650583121));
#45366=CARTESIAN_POINT('Ctrl Pts',(-4.34289632261169,4.72597200984736,-8.19454158619059));
#45367=CARTESIAN_POINT('Ctrl Pts',(-4.34761742866533,4.74846286165763,-8.20123397235553));
#45368=CARTESIAN_POINT('Ctrl Pts',(-4.35611858405088,4.78896147020831,-8.21328475326194));
#45369=CARTESIAN_POINT('Ctrl Pts',(-4.364273915394,4.82830494345656,-8.22532315857519));
#45370=CARTESIAN_POINT('Ctrl Pts',(-4.37211914663514,4.86667596289883,-8.23730455666148));
#45371=CARTESIAN_POINT('Ctrl Pts',(-4.37368661971269,4.87434247241082,-8.23969843370021));
#45372=CARTESIAN_POINT('Ctrl Pts',(-4.37524162712662,4.88197012218228,-8.242090172428));
#45373=CARTESIAN_POINT('Ctrl Pts',(-4.37678433287212,4.88956030660734,-8.2444796159815));
#45374=CARTESIAN_POINT('Ctrl Pts',(-4.37902935186565,4.90060590506209,-8.2479568482257));
#45375=CARTESIAN_POINT('Ctrl Pts',(-4.38124832515402,4.91157216617416,-8.25142920855899));
#45376=CARTESIAN_POINT('Ctrl Pts',(-4.38344168155448,4.92246328084618,-8.25489644172617));
#45377=CARTESIAN_POINT('Ctrl Pts',(-4.39166806457672,4.96331139874085,-8.26790061562817));
#45378=CARTESIAN_POINT('Ctrl Pts',(-4.39953784164126,5.00310352140156,-8.28082847158412));
#45379=CARTESIAN_POINT('Ctrl Pts',(-4.40710031519932,5.0420845185481,-8.29367497391344));
#45380=CARTESIAN_POINT('Ctrl Pts',(-4.40987453259679,5.05638430546631,-8.29838758414408));
#45381=CARTESIAN_POINT('Ctrl Pts',(-4.41260709492868,5.07057477963414,-8.30308964658198));
#45382=CARTESIAN_POINT('Ctrl Pts',(-4.41529949361838,5.08466746076063,-8.30778221778098));
#45383=CARTESIAN_POINT('Ctrl Pts',(-4.42221585975252,5.12086943294823,-8.31983672540163));
#45384=CARTESIAN_POINT('Ctrl Pts',(-4.42886821819497,5.15642611577934,-8.33182742100887));
#45385=CARTESIAN_POINT('Ctrl Pts',(-4.43533386389712,5.19175782809657,-8.34384585123646));
#45386=CARTESIAN_POINT('Ctrl Pts',(-4.43824630695621,5.20767295939887,-8.34925954003258));
#45387=CARTESIAN_POINT('Ctrl Pts',(-4.44112032917328,5.22354220343738,-8.3546793029189));
#45388=CARTESIAN_POINT('Ctrl Pts',(-4.44396054595061,5.2394028053282,-8.36011551828689));
#45389=CARTESIAN_POINT('Ctrl Pts',(-4.44405208094427,5.23991396352748,-8.36029071756857));
#45390=CARTESIAN_POINT('Ctrl Pts',(-4.4441435811585,5.24042511291043,-8.36046593366695));
#45391=CARTESIAN_POINT('Ctrl Pts',(-4.44423504674774,5.24093625444961,-8.36064116678035));
#45392=CARTESIAN_POINT('Ctrl Pts',(-4.45126642086968,5.28023001968963,-8.37411212989425));
#45393=CARTESIAN_POINT('Ctrl Pts',(-4.4580969244534,5.31947864261195,-8.38768154521493));
#45394=CARTESIAN_POINT('Ctrl Pts',(-4.46477647644197,5.35911589791667,-8.40145256371401));
#45395=CARTESIAN_POINT('Ctrl Pts',(-4.46669136199904,5.37047905637922,-8.40540042196486));
#45396=CARTESIAN_POINT('Ctrl Pts',(-4.46859356314506,5.38187406300918,-8.40936500143831));
#45397=CARTESIAN_POINT('Ctrl Pts',(-4.47048359648073,5.39331091775106,-8.41334907958716));
#45398=CARTESIAN_POINT('Ctrl Pts',(-4.47856333289223,5.44220252719894,-8.43038068462712));
#45399=CARTESIAN_POINT('Ctrl Pts',(-4.4864278178208,5.49186297696528,-8.4477622190913));
#45400=CARTESIAN_POINT('Ctrl Pts',(-4.49394679880183,5.5418615608125,-8.46523514881534));
#45401=CARTESIAN_POINT('Ctrl Pts',(-4.4944017865307,5.54488706947768,-8.46629246876759));
#45402=CARTESIAN_POINT('Ctrl Pts',(-4.49485551848749,5.54791382557571,-8.46735011515994));
#45403=CARTESIAN_POINT('Ctrl Pts',(-4.49530796933741,5.55094173716409,-8.46840802772342));
#45404=CARTESIAN_POINT('Ctrl Pts',(-4.49842936112357,5.57183085332511,-8.47570641071172));
#45405=CARTESIAN_POINT('Ctrl Pts',(-4.50148971645701,5.59277488701679,-8.48301746154873));
#45406=CARTESIAN_POINT('Ctrl Pts',(-4.50448016791163,5.61373871123014,-8.49031968227011));
#45407=CARTESIAN_POINT('Ctrl Pts',(-4.50908658699107,5.64603087891788,-8.50156784642317));
#45408=CARTESIAN_POINT('Ctrl Pts',(-4.51352685215888,5.67836985658108,-8.51279513010456));
#45409=CARTESIAN_POINT('Ctrl Pts',(-4.51777558989158,5.71063032301425,-8.52392064421601));
#45410=CARTESIAN_POINT('Ctrl Pts',(-4.52302272751204,5.75047159299255,-8.53766051410537));
#45411=CARTESIAN_POINT('Ctrl Pts',(-4.52797840478413,5.7901902785537,-8.55124943731126));
#45412=CARTESIAN_POINT('Ctrl Pts',(-4.5326783182324,5.83017642858429,-8.56472139707146));
#45413=CARTESIAN_POINT('Ctrl Pts',(-4.53425463127801,5.84358746064495,-8.56923978366596));
#45414=CARTESIAN_POINT('Ctrl Pts',(-4.53580175308728,5.85702853586363,-8.57374510959597));
#45415=CARTESIAN_POINT('Ctrl Pts',(-4.5373197575171,5.87051423416948,-8.57823892982017));
#45416=CARTESIAN_POINT('Ctrl Pts',(-4.5407839353761,5.90128941279634,-8.58849409918404));
#45417=CARTESIAN_POINT('Ctrl Pts',(-4.54409817423199,5.93229529921562,-8.59869252527202));
#45418=CARTESIAN_POINT('Ctrl Pts',(-4.54729858503435,5.96400552331454,-8.60889569284174));
#45419=CARTESIAN_POINT('Ctrl Pts',(-4.54906917871499,5.98154887192456,-8.61454048819366));
#45420=CARTESIAN_POINT('Ctrl Pts',(-4.55080405929922,5.99930777943827,-8.62018683029092));
#45421=CARTESIAN_POINT('Ctrl Pts',(-4.55250246845951,6.01736224798488,-8.62584575846157));
#45422=CARTESIAN_POINT('Ctrl Pts',(-4.5530903412421,6.02361146690753,-8.62780449133231));
#45423=CARTESIAN_POINT('Ctrl Pts',(-4.55367379927466,6.02989609461737,-8.62976473564345));
#45424=CARTESIAN_POINT('Ctrl Pts',(-4.55425268031317,6.03621944303901,-8.6317269597769));
#45425=CARTESIAN_POINT('Ctrl Pts',(-4.55790067810912,6.07606797766111,-8.64409252167612));
#45426=CARTESIAN_POINT('Ctrl Pts',(-4.56137444979074,6.11745813508607,-8.65653174714067));
#45427=CARTESIAN_POINT('Ctrl Pts',(-4.56459141140092,6.16021282589141,-8.66862512082167));
#45428=CARTESIAN_POINT('Ctrl Pts',(-4.56602514958334,6.17926777279885,-8.67401490587408));
#45429=CARTESIAN_POINT('Ctrl Pts',(-4.56740721900955,6.19859409140341,-8.67933586498138));
#45430=CARTESIAN_POINT('Ctrl Pts',(-4.56872735814743,6.21817739199662,-8.68455045311303));
#45431=CARTESIAN_POINT('',(-4.55640048587279,6.70157635552431,-8.9543685982643));
#45432=CARTESIAN_POINT('Ctrl Pts',(-4.55640048587279,6.70157635552431,-8.9543685982643));
#45433=CARTESIAN_POINT('Ctrl Pts',(-4.55718941624934,6.67123679535193,-8.93709741994231));
#45434=CARTESIAN_POINT('Ctrl Pts',(-4.55798670386089,6.64094052514093,-8.9197505370997));
#45435=CARTESIAN_POINT('Ctrl Pts',(-4.56052339181447,6.54280654655596,-8.86421763865645));
#45436=CARTESIAN_POINT('Ctrl Pts',(-4.56140069340555,6.50873740836523,-8.84501184706769));
#45437=CARTESIAN_POINT('Ctrl Pts',(-4.56478339758665,6.37642811190917,-8.77095805283272));
#45438=CARTESIAN_POINT('Ctrl Pts',(-4.56675535639669,6.29828421554187,-8.72778814374827));
#45439=CARTESIAN_POINT('Ctrl Pts',(-4.56873070446287,6.21818495489539,-8.68454403743452));
#45440=CARTESIAN_POINT('Origin',(-1.55120871661933,6.72678389660421,-8.99999785420734));
#45441=CARTESIAN_POINT('Ctrl Pts',(-4.045081305886,3.570670526222,-7.997140252951));
#45442=CARTESIAN_POINT('Ctrl Pts',(-4.046812898614,3.579264725453,-7.997221249461));
#45443=CARTESIAN_POINT('Ctrl Pts',(-4.067641295895,3.682284597448,-7.998756172751));
#45444=CARTESIAN_POINT('Ctrl Pts',(-4.107485147684,3.871753164572,-8.0136447426));
#45445=CARTESIAN_POINT('Ctrl Pts',(-4.164985230409,4.131365060025,-8.057273037248));
#45446=CARTESIAN_POINT('Ctrl Pts',(-4.218249503093,4.365529545906,-8.111730462255));
#45447=CARTESIAN_POINT('Ctrl Pts',(-4.266684104315,4.577338170023,-8.170825174353));
#45448=CARTESIAN_POINT('Ctrl Pts',(-4.310160116143,4.769912949898,-8.230914655747));
#45449=CARTESIAN_POINT('Ctrl Pts',(-4.349046949732,4.946950105447,-8.290246855678));
#45450=CARTESIAN_POINT('Ctrl Pts',(-4.384026666367,5.112794198023,-8.348441680794));
#45451=CARTESIAN_POINT('Ctrl Pts',(-4.416117162443,5.273132430747,-8.406311113417));
#45452=CARTESIAN_POINT('Ctrl Pts',(-4.446085672278,5.433323459631,-8.464981611408));
#45453=CARTESIAN_POINT('Ctrl Pts',(-4.473991447656,5.595899742481,-8.52460059918));
#45454=CARTESIAN_POINT('Ctrl Pts',(-4.499372620983,5.761043207801,-8.584261950216));
#45455=CARTESIAN_POINT('Ctrl Pts',(-4.522096645264,5.931133599072,-8.643540441466));
#45456=CARTESIAN_POINT('Ctrl Pts',(-4.539342084936,6.086914371239,-8.694069503927));
#45457=CARTESIAN_POINT('Ctrl Pts',(-4.548382886192,6.188750654892,-8.723456408556));
#45458=CARTESIAN_POINT('Ctrl Pts',(-4.551596987486,6.22933872244,-8.734309456469));
#45459=CARTESIAN_POINT('Ctrl Pts',(-4.38444310932,3.571151919152,-8.034638616021));
#45460=CARTESIAN_POINT('Ctrl Pts',(-4.386305205191,3.579569394099,-8.033539372566));
#45461=CARTESIAN_POINT('Ctrl Pts',(-4.408629897612,3.68066734286,-8.020861884741));
#45462=CARTESIAN_POINT('Ctrl Pts',(-4.449669636584,3.870894091304,-8.008352060743));
#45463=CARTESIAN_POINT('Ctrl Pts',(-4.504232539929,4.140353391516,-8.013736794392));
#45464=CARTESIAN_POINT('Ctrl Pts',(-4.55063177438,4.389097996571,-8.034425921765));
#45465=CARTESIAN_POINT('Ctrl Pts',(-4.589150445557,4.617533446599,-8.064277722446));
#45466=CARTESIAN_POINT('Ctrl Pts',(-4.620473992277,4.827070553768,-8.099234200262));
#45467=CARTESIAN_POINT('Ctrl Pts',(-4.645574637769,5.020459022684,-8.136859011721));
#45468=CARTESIAN_POINT('Ctrl Pts',(-4.665466157709,5.201634738077,-8.176014130233));
#45469=CARTESIAN_POINT('Ctrl Pts',(-4.681108266095,5.376219387118,-8.216640487237));
#45470=CARTESIAN_POINT('Ctrl Pts',(-4.693013028977,5.549502857778,-8.259177343643));
#45471=CARTESIAN_POINT('Ctrl Pts',(-4.701160151981,5.723479739884,-8.303369398396));
#45472=CARTESIAN_POINT('Ctrl Pts',(-4.705392710052,5.897297469717,-8.348024465499));
#45473=CARTESIAN_POINT('Ctrl Pts',(-4.70577776434,6.071962157169,-8.39204144798));
#45474=CARTESIAN_POINT('Ctrl Pts',(-4.702814699302,6.225389199561,-8.427814383606));
#45475=CARTESIAN_POINT('Ctrl Pts',(-4.699547889202,6.319867306073,-8.446724606978));
#45476=CARTESIAN_POINT('Ctrl Pts',(-4.698140530724,6.356053961272,-8.453204386312));
#45477=CARTESIAN_POINT('Ctrl Pts',(-4.628389217157,3.568085518823,-7.795779646061));
#45478=CARTESIAN_POINT('Ctrl Pts',(-4.629418893889,3.577521107695,-7.79381729154));
#45479=CARTESIAN_POINT('Ctrl Pts',(-4.641684342718,3.690860050951,-7.770895214064));
#45480=CARTESIAN_POINT('Ctrl Pts',(-4.662425768587,3.904374357362,-7.741811913326));
#45481=CARTESIAN_POINT('Ctrl Pts',(-4.684742285256,4.205673471946,-7.730144464707));
#45482=CARTESIAN_POINT('Ctrl Pts',(-4.698645983965,4.481620469159,-7.740018549965));
#45483=CARTESIAN_POINT('Ctrl Pts',(-4.705289198756,4.732378398938,-7.7636822036));
#45484=CARTESIAN_POINT('Ctrl Pts',(-4.705941242827,4.959625634746,-7.795795708981));
#45485=CARTESIAN_POINT('Ctrl Pts',(-4.701760894077,5.16663338348,-7.832943907084));
#45486=CARTESIAN_POINT('Ctrl Pts',(-4.693611570147,5.357939474718,-7.873319066008));
#45487=CARTESIAN_POINT('Ctrl Pts',(-4.681878224428,5.539622768666,-7.916425840639));
#45488=CARTESIAN_POINT('Ctrl Pts',(-4.666505871274,5.717138279957,-7.962487458925));
#45489=CARTESIAN_POINT('Ctrl Pts',(-4.647392526364,5.892143191488,-8.010987241641));
#45490=CARTESIAN_POINT('Ctrl Pts',(-4.624818466659,6.063207414259,-8.060275721544));
#45491=CARTESIAN_POINT('Ctrl Pts',(-4.599047213946,6.230443318226,-8.108633744215));
#45492=CARTESIAN_POINT('Ctrl Pts',(-4.574172291028,6.371245573819,-8.146796806519));
#45493=CARTESIAN_POINT('Ctrl Pts',(-4.558333187126,6.452902211151,-8.165676958464));
#45494=CARTESIAN_POINT('Ctrl Pts',(-4.552300465109,6.482885359553,-8.171767808125));
#45495=CARTESIAN_POINT('Ctrl Pts',(-4.59801848,3.563720111035,-7.455733771689));
#45496=CARTESIAN_POINT('Ctrl Pts',(-4.597863281049,3.574622004543,-7.453858409074));
#45497=CARTESIAN_POINT('Ctrl Pts',(-4.595891028734,3.705387762562,-7.432172570609));
#45498=CARTESIAN_POINT('Ctrl Pts',(-4.589725981319,3.947640760677,-7.409495091648));
#45499=CARTESIAN_POINT('Ctrl Pts',(-4.574135224093,4.279421944416,-7.414472286021));
#45500=CARTESIAN_POINT('Ctrl Pts',(-4.553743926439,4.57524436771,-7.444415940845));
#45501=CARTESIAN_POINT('Ctrl Pts',(-4.529928451882,4.83764994122,-7.489484372422));
#45502=CARTESIAN_POINT('Ctrl Pts',(-4.503883313521,5.07036714669,-7.543129868468));
#45503=CARTESIAN_POINT('Ctrl Pts',(-4.476400774158,5.278274260209,-7.601381759125));
#45504=CARTESIAN_POINT('Ctrl Pts',(-4.447822088052,5.467080233349,-7.662341972482));
#45505=CARTESIAN_POINT('Ctrl Pts',(-4.417862378173,5.643508514361,-7.725833610458));
#45506=CARTESIAN_POINT('Ctrl Pts',(-4.38600357872,5.813292041393,-7.792493462698));
#45507=CARTESIAN_POINT('Ctrl Pts',(-4.352119780053,5.978198493352,-7.861876504293));
#45508=CARTESIAN_POINT('Ctrl Pts',(-4.316740092663,6.137100758815,-7.932040118318));
#45509=CARTESIAN_POINT('Ctrl Pts',(-4.280177274426,6.290352797616,-8.001158170104));
#45510=CARTESIAN_POINT('Ctrl Pts',(-4.247756495264,6.41751776608,-8.057104781149));
#45511=CARTESIAN_POINT('Ctrl Pts',(-4.228300475361,6.490292438545,-8.086423524783));
#45512=CARTESIAN_POINT('Ctrl Pts',(-4.221030558413,6.516819410599,-8.096395010467));
#45513=CARTESIAN_POINT('',(-4.59947917151011,5.30712985987108,-8.01140192098629));
#45514=CARTESIAN_POINT('Ctrl Pts',(-4.56872994952894,6.2181719957563,-8.68456056436646));
#45515=CARTESIAN_POINT('Ctrl Pts',(-4.57549039229006,5.94407403599775,-8.53656168229868));
#45516=CARTESIAN_POINT('Ctrl Pts',(-4.58829230843072,5.57742483423423,-8.25630351813582));
#45517=CARTESIAN_POINT('Ctrl Pts',(-4.59463727532969,5.39767807259543,-8.1174001887258));
#45518=CARTESIAN_POINT('Ctrl Pts',(-4.59661627982459,5.34707828533855,-8.07407603627248));
#45519=CARTESIAN_POINT('Ctrl Pts',(-4.59817842627609,5.31873497780432,-8.03987769503683));
#45520=CARTESIAN_POINT('Ctrl Pts',(-4.59846257897685,5.31405574435703,-8.03365705483116));
#45521=CARTESIAN_POINT('Ctrl Pts',(-4.59885735472505,5.30945783900961,-8.02501466682989));
#45522=CARTESIAN_POINT('Ctrl Pts',(-4.59898970613569,5.3081737583618,-8.02211724405618));
#45523=CARTESIAN_POINT('Ctrl Pts',(-4.59918120343943,5.30709898285999,-8.01792500578503));
#45524=CARTESIAN_POINT('Ctrl Pts',(-4.59924313552705,5.30686343682691,-8.01656919521855));
#45525=CARTESIAN_POINT('Ctrl Pts',(-4.59936367370055,5.30673568281945,-8.01393038655558));
#45526=CARTESIAN_POINT('Ctrl Pts',(-4.59942203451764,5.3068253754564,-8.01265275785716));
#45527=CARTESIAN_POINT('Ctrl Pts',(-4.59947916602947,5.30713035297914,-8.01140204097648));
#45528=CARTESIAN_POINT('Origin',(-4.100000000002,3.596479003779,-7.500000152636));
#45529=CARTESIAN_POINT('Origin',(-4.16921629989938,5.30178033932293,-7.99516079097523));
#45530=CARTESIAN_POINT('Origin',(-4.6,0.,-8.));
#45531=CARTESIAN_POINT('',(-4.59947849846395,10.4125163640988,-8.01141603935184));
#45532=CARTESIAN_POINT('',(-4.599479171875,5.307129343005,-8.011401913));
#45533=CARTESIAN_POINT('',(-4.23,10.14289693909,-16.1));
#45534=CARTESIAN_POINT('',(-4.556403751801,6.701576438348,-8.954368601956));
#45535=CARTESIAN_POINT('Origin',(-3.762822538146,0.03215126727281,39.41676));
#45536=CARTESIAN_POINT('Origin',(0.2082147951869,9.091108462706,-47.51676));
#45537=CARTESIAN_POINT('',(-1.60105661523759,13.4097223134493,-8.00833023504569));
#45538=CARTESIAN_POINT('Ctrl Pts',(-4.59947852653901,10.4125163641,-8.01141604063367));
#45539=CARTESIAN_POINT('Ctrl Pts',(-4.59937714658466,10.5053599489842,-8.01363546696004));
#45540=CARTESIAN_POINT('Ctrl Pts',(-4.59496139431105,10.5981056187004,-8.01571294302175));
#45541=CARTESIAN_POINT('Ctrl Pts',(-4.58628390044264,10.6903162581727,-8.01764532333119));
#45542=CARTESIAN_POINT('Ctrl Pts',(-4.57759483258553,10.7826498876368,-8.01958028103776));
#45543=CARTESIAN_POINT('Ctrl Pts',(-4.56463275739157,10.8744466105326,-8.02136974578396));
#45544=CARTESIAN_POINT('Ctrl Pts',(-4.54750132154224,10.9652793145299,-8.02301327200983));
#45545=CARTESIAN_POINT('Ctrl Pts',(-4.54553480512527,10.9757059947673,-8.02320193227936));
#45546=CARTESIAN_POINT('Ctrl Pts',(-4.54351340395201,10.9861199893966,-8.0233886725801));
#45547=CARTESIAN_POINT('Ctrl Pts',(-4.54143731634338,10.9965206663834,-8.02357349460259));
#45548=CARTESIAN_POINT('Ctrl Pts',(-4.51373868008413,11.1352838705519,-8.02603934332322));
#45549=CARTESIAN_POINT('Ctrl Pts',(-4.47631109928855,11.2716724237222,-8.02816384317182));
#45550=CARTESIAN_POINT('Ctrl Pts',(-4.42949368679031,11.4047754243669,-8.02995529417993));
#45551=CARTESIAN_POINT('Ctrl Pts',(-4.41170336822207,11.4553537168761,-8.03063603415323));
#45552=CARTESIAN_POINT('Ctrl Pts',(-4.39255663241803,11.5054576939607,-8.03126866081907));
#45553=CARTESIAN_POINT('Ctrl Pts',(-4.37207018210256,11.5550370833454,-8.03185353288804));
#45554=CARTESIAN_POINT('Ctrl Pts',(-4.33487064946315,11.6450639101143,-8.03291555033294));
#45555=CARTESIAN_POINT('Ctrl Pts',(-4.29325008333227,11.7333572007709,-8.03381981135128));
#45556=CARTESIAN_POINT('Ctrl Pts',(-4.24739909147331,11.8194638381191,-8.03456476480664));
#45557=CARTESIAN_POINT('Ctrl Pts',(-4.20154809961434,11.9055704754674,-8.03530971826199));
#45558=CARTESIAN_POINT('Ctrl Pts',(-4.15146687069939,11.9894900264455,-8.03589535833731));
#45559=CARTESIAN_POINT('Ctrl Pts',(-4.09739699750768,12.070792842957,-8.03632324514469));
#45560=CARTESIAN_POINT('Ctrl Pts',(-4.04332712431596,12.1520956594685,-8.03675113195206));
#45561=CARTESIAN_POINT('Ctrl Pts',(-3.98526494673421,12.2307867534014,-8.03702126536406));
#45562=CARTESIAN_POINT('Ctrl Pts',(-3.92350391936216,12.306459541199,-8.03713533101613));
#45563=CARTESIAN_POINT('Ctrl Pts',(-3.8617428919901,12.3821323289966,-8.0372493966682));
#45564=CARTESIAN_POINT('Ctrl Pts',(-3.79628334587537,12.4547864053715,-8.03720739617268));
#45565=CARTESIAN_POINT('Ctrl Pts',(-3.7274646744854,12.5240527119111,-8.03701436444527));
#45566=CARTESIAN_POINT('Ctrl Pts',(-3.61008311621264,12.6421977855254,-8.03668511709856));
#45567=CARTESIAN_POINT('Ctrl Pts',(-3.48294186288595,12.7504976082822,-8.03591742735363));
#45568=CARTESIAN_POINT('Ctrl Pts',(-3.34726077786289,12.8477785188959,-8.03473979822533));
#45569=CARTESIAN_POINT('Ctrl Pts',(-3.32384716110428,12.86456566324,-8.0345365823011));
#45570=CARTESIAN_POINT('Ctrl Pts',(-3.30017927632364,12.8810245622901,-8.03432115655264));
#45571=CARTESIAN_POINT('Ctrl Pts',(-3.27626347960308,12.8971490029899,-8.03409366538231));
#45572=CARTESIAN_POINT('Ctrl Pts',(-3.19500998112919,12.9519315065,-8.03332076813462));
#45573=CARTESIAN_POINT('Ctrl Pts',(-3.11089288436003,13.0028487928325,-8.03240835728523));
#45574=CARTESIAN_POINT('Ctrl Pts',(-3.02431349873321,13.0495898432854,-8.03136655596011));
#45575=CARTESIAN_POINT('Ctrl Pts',(-2.93773411310639,13.0963308937382,-8.03032475463499));
#45576=CARTESIAN_POINT('Ctrl Pts',(-2.84869282192845,13.1388953619482,-8.02915356879778));
#45577=CARTESIAN_POINT('Ctrl Pts',(-2.75762808262276,13.1770189882356,-8.02786637709185));
#45578=CARTESIAN_POINT('Ctrl Pts',(-2.6767553243985,13.2108758117974,-8.02672324810016));
#45579=CARTESIAN_POINT('Ctrl Pts',(-2.59428155331456,13.2412318658843,-8.02548844708348));
#45580=CARTESIAN_POINT('Ctrl Pts',(-2.51057491999558,13.2679253202654,-8.02417544528473));
#45581=CARTESIAN_POINT('Ctrl Pts',(-2.42689667427439,13.2946097220419,-8.02286288876689));
#45582=CARTESIAN_POINT('Ctrl Pts',(-2.3419868696778,13.3176338274672,-8.02147219982988));
#45583=CARTESIAN_POINT('Ctrl Pts',(-2.25623169518505,13.3368846145964,-8.02001929854991));
#45584=CARTESIAN_POINT('Ctrl Pts',(-2.23458069613051,13.341744948406,-8.01965247795366));
#45585=CARTESIAN_POINT('Ctrl Pts',(-2.21287588198184,13.3463650071242,-8.01928170330574));
#45586=CARTESIAN_POINT('Ctrl Pts',(-2.19112359772689,13.3507434805461,-8.01890725370485));
#45587=CARTESIAN_POINT('Ctrl Pts',(-2.08550224293537,13.3720037900068,-8.01708905963921));
#45588=CARTESIAN_POINT('Ctrl Pts',(-1.97875576869714,13.3875653723446,-8.01518385709241));
#45589=CARTESIAN_POINT('Ctrl Pts',(-1.87146594973527,13.3973435107752,-8.01324431200059));
#45590=CARTESIAN_POINT('Ctrl Pts',(-1.781595528025,13.4055340868504,-8.01161966823649));
#45591=CARTESIAN_POINT('Ctrl Pts',(-1.6913440848234,13.4096676346005,-8.0099709675611));
#45592=CARTESIAN_POINT('Ctrl Pts',(-1.601056615238,13.4097223254853,-8.00833023544683));
#45593=CARTESIAN_POINT('',(-1.231437138339,13.14,-16.1));
#45594=CARTESIAN_POINT('Ctrl Pts',(-4.598789897208,10.36225164745,-8.016476101857));
#45595=CARTESIAN_POINT('Ctrl Pts',(-4.59904872628,10.37845482038,-8.016780636338));
#45596=CARTESIAN_POINT('Ctrl Pts',(-4.600707128738,10.59084307586,-8.020727567036));
#45597=CARTESIAN_POINT('Ctrl Pts',(-4.560432831713,10.99871853828,-8.027206255404));
#45598=CARTESIAN_POINT('Ctrl Pts',(-4.389548448443,11.56244686259,-8.033690401801));
#45599=CARTESIAN_POINT('Ctrl Pts',(-4.113161687858,12.08156245964,-8.03737709449));
#45600=CARTESIAN_POINT('Ctrl Pts',(-3.740911740519,12.53762144943,-8.038338406857));
#45601=CARTESIAN_POINT('Ctrl Pts',(-3.285897948442,12.91378212525,-8.036724743215));
#45602=CARTESIAN_POINT('Ctrl Pts',(-2.763990158324,13.19524941593,-8.032801897215));
#45603=CARTESIAN_POINT('Ctrl Pts',(-2.194549095368,13.36974564586,-8.027048720184));
#45604=CARTESIAN_POINT('Ctrl Pts',(-1.782256775266,13.41072702305,-8.022378740496));
#45605=CARTESIAN_POINT('Ctrl Pts',(-1.568450922092,13.40904708803,-8.020131894078));
#45606=CARTESIAN_POINT('Ctrl Pts',(-1.552548505891,13.40879470923,-8.019965863476));
#45607=CARTESIAN_POINT('Ctrl Pts',(-4.599357509043,10.36246318279,-8.006699568108));
#45608=CARTESIAN_POINT('Ctrl Pts',(-4.599615170043,10.37866779227,-8.007004055868));
#45609=CARTESIAN_POINT('Ctrl Pts',(-4.60125828296,10.59107480655,-8.010950502452));
#45610=CARTESIAN_POINT('Ctrl Pts',(-4.560955080986,10.99898457628,-8.017428460088));
#45611=CARTESIAN_POINT('Ctrl Pts',(-4.39003073768,11.56275691357,-8.0239118523));
#45612=CARTESIAN_POINT('Ctrl Pts',(-4.113605718657,12.08191367378,-8.027598129646));
#45613=CARTESIAN_POINT('Ctrl Pts',(-3.741317226717,12.53801415694,-8.028559340472));
#45614=CARTESIAN_POINT('Ctrl Pts',(-3.286260517087,12.91421890722,-8.026945846688));
#45615=CARTESIAN_POINT('Ctrl Pts',(-2.764299375992,13.19573306602,-8.023023342469));
#45616=CARTESIAN_POINT('Ctrl Pts',(-2.194786161204,13.37027585393,-8.017270521009));
#45617=CARTESIAN_POINT('Ctrl Pts',(-1.782422450544,13.41128407841,-8.012600588629));
#45618=CARTESIAN_POINT('Ctrl Pts',(-1.568567787561,13.40961256521,-8.010353640725));
#45619=CARTESIAN_POINT('Ctrl Pts',(-1.552661674054,13.40936077555,-8.01018761061));
#45620=CARTESIAN_POINT('Ctrl Pts',(-4.599637634666,10.36267951191,-7.996910682916));
#45621=CARTESIAN_POINT('Ctrl Pts',(-4.599894101587,10.37888400298,-7.997215123896));
#45622=CARTESIAN_POINT('Ctrl Pts',(-4.601521750683,10.59128939393,-8.001161085754));
#45623=CARTESIAN_POINT('Ctrl Pts',(-4.561193484141,10.99919432699,-8.007638311736));
#45624=CARTESIAN_POINT('Ctrl Pts',(-4.390245555465,11.56295657265,-8.01412094881));
#45625=CARTESIAN_POINT('Ctrl Pts',(-4.113808788278,12.08210467379,-8.017806810288));
#45626=CARTESIAN_POINT('Ctrl Pts',(-3.741517469637,12.53820288521,-8.018767919443));
#45627=CARTESIAN_POINT('Ctrl Pts',(-3.286461505785,12.91441562184,-8.017154595732));
#45628=CARTESIAN_POINT('Ctrl Pts',(-2.764497092176,13.19594965895,-8.013232433727));
#45629=CARTESIAN_POINT('Ctrl Pts',(-2.194966351295,13.37052228964,-8.007479968285));
#45630=CARTESIAN_POINT('Ctrl Pts',(-1.782570781966,13.41155345129,-8.002810083274));
#45631=CARTESIAN_POINT('Ctrl Pts',(-1.568687797996,13.40989052953,-8.000563033756));
#45632=CARTESIAN_POINT('Ctrl Pts',(-1.552779511032,13.40963935383,-8.000397004128));
#45633=CARTESIAN_POINT('Ctrl Pts',(-4.59963003227,10.36290044807,-7.987117896224));
#45634=CARTESIAN_POINT('Ctrl Pts',(-4.599885280135,10.37910326588,-7.987422290406));
#45635=CARTESIAN_POINT('Ctrl Pts',(-4.601497304476,10.59148665279,-7.991367767344));
#45636=CARTESIAN_POINT('Ctrl Pts',(-4.561147835383,10.99934760934,-7.997844261379));
#45637=CARTESIAN_POINT('Ctrl Pts',(-4.390192716364,11.56304566748,-8.004326143015));
#45638=CARTESIAN_POINT('Ctrl Pts',(-4.113770721428,12.08213529482,-8.00801158846));
#45639=CARTESIAN_POINT('Ctrl Pts',(-3.741512296425,12.53818747134,-8.008972595904));
#45640=CARTESIAN_POINT('Ctrl Pts',(-3.286500741038,12.91437209929,-8.007359442333));
#45641=CARTESIAN_POINT('Ctrl Pts',(-2.764583136204,13.19589900775,-8.003437622678));
#45642=CARTESIAN_POINT('Ctrl Pts',(-2.1950895101,13.37048474024,-7.997685513398));
#45643=CARTESIAN_POINT('Ctrl Pts',(-1.78270164149,13.41153490917,-7.993015675774));
#45644=CARTESIAN_POINT('Ctrl Pts',(-1.568810849802,13.40988074104,-7.990768524601));
#45645=CARTESIAN_POINT('Ctrl Pts',(-1.552901915106,13.4096302036,-7.99060249546));
#45646=CARTESIAN_POINT('Origin',(-4.16374842361929,10.412721159634,-7.98938980904604));
#45647=CARTESIAN_POINT('',(-1.59999999919565,13.4100000197175,-7.99166557366509));
#45648=CARTESIAN_POINT('Ctrl Pts',(-4.60000007096128,10.4099999970624,-7.98856626783489));
#45649=CARTESIAN_POINT('Ctrl Pts',(-4.60000004790308,10.4105031362908,-7.98857551592105));
#45650=CARTESIAN_POINT('Ctrl Pts',(-4.59999989765145,10.4110062701598,-7.98858476064926));
#45651=CARTESIAN_POINT('Ctrl Pts',(-4.59999962022458,10.4115093985946,-7.98859400202004));
#45652=CARTESIAN_POINT('Ctrl Pts',(-4.59993230689588,10.5335857136227,-7.99083627737669));
#45653=CARTESIAN_POINT('Ctrl Pts',(-4.59237725989827,10.6553379562347,-7.99288087440913));
#45654=CARTESIAN_POINT('Ctrl Pts',(-4.57759893061383,10.7757227708346,-7.99473560830003));
#45655=CARTESIAN_POINT('Ctrl Pts',(-4.56846846564521,10.8500998747211,-7.99588151474798));
#45656=CARTESIAN_POINT('Ctrl Pts',(-4.55658096803786,10.923955981217,-7.99695495345506));
#45657=CARTESIAN_POINT('Ctrl Pts',(-4.54200043259281,10.9970548991584,-7.99795781611259));
#45658=CARTESIAN_POINT('Ctrl Pts',(-4.52558397978909,11.0793581136673,-7.99908695485703));
#45659=CARTESIAN_POINT('Ctrl Pts',(-4.50575945226007,11.1606958296678,-8.0001261358151));
#45660=CARTESIAN_POINT('Ctrl Pts',(-4.48262123061731,11.2409571557528,-8.0010784943899));
#45661=CARTESIAN_POINT('Ctrl Pts',(-4.45934493853253,11.3216974173819,-8.00203653588067));
#45662=CARTESIAN_POINT('Ctrl Pts',(-4.43271510472733,11.4013490785121,-8.0029067152227));
#45663=CARTESIAN_POINT('Ctrl Pts',(-4.40277644619052,11.4797889721212,-8.00369093516911));
#45664=CARTESIAN_POINT('Ctrl Pts',(-4.39308369326812,11.5051841816988,-8.00394482931631));
#45665=CARTESIAN_POINT('Ctrl Pts',(-4.38304373262649,11.5304522553539,-8.00418970349656));
#45666=CARTESIAN_POINT('Ctrl Pts',(-4.3726569846437,11.5555886022102,-8.00442559364283));
#45667=CARTESIAN_POINT('Ctrl Pts',(-4.32570548047689,11.6692131260859,-8.0054918943949));
#45668=CARTESIAN_POINT('Ctrl Pts',(-4.27166654431615,11.780135431829,-8.00637598720223));
#45669=CARTESIAN_POINT('Ctrl Pts',(-4.21097666130231,11.8874037929216,-8.00707791501786));
#45670=CARTESIAN_POINT('Ctrl Pts',(-4.1755470119615,11.9500251101847,-8.00748768770377));
#45671=CARTESIAN_POINT('Ctrl Pts',(-4.13785171758996,12.0114012978217,-8.00783540238063));
#45672=CARTESIAN_POINT('Ctrl Pts',(-4.09798539657222,12.0713455265286,-8.00812126625666));
#45673=CARTESIAN_POINT('Ctrl Pts',(-4.01821661670886,12.1912883218939,-8.00869325313722));
#45674=CARTESIAN_POINT('Ctrl Pts',(-3.92974727531656,12.3055066806468,-8.0090173854157));
#45675=CARTESIAN_POINT('Ctrl Pts',(-3.83357869973105,12.4127697983396,-8.00910502114443));
#45676=CARTESIAN_POINT('Ctrl Pts',(-3.79935520257316,12.450941508601,-8.0091362080586));
#45677=CARTESIAN_POINT('Ctrl Pts',(-3.76415703204153,12.4882326737266,-8.00913745552344));
#45678=CARTESIAN_POINT('Ctrl Pts',(-3.7280304834056,12.5245889108034,-8.009109311589));
#45679=CARTESIAN_POINT('Ctrl Pts',(-3.65853132117118,12.5945299407175,-8.00905516913865));
#45680=CARTESIAN_POINT('Ctrl Pts',(-3.58560242986534,12.6610112485787,-8.00889192038084));
#45681=CARTESIAN_POINT('Ctrl Pts',(-3.50950976494343,12.7238085936419,-8.00862540876549));
#45682=CARTESIAN_POINT('Ctrl Pts',(-3.43490130270294,12.7853810639024,-8.00836409551261));
#45683=CARTESIAN_POINT('Ctrl Pts',(-3.35725059062315,12.843412269591,-8.00800349515826));
#45684=CARTESIAN_POINT('Ctrl Pts',(-3.27678144871871,12.8976502915845,-8.00754815778184));
#45685=CARTESIAN_POINT('Ctrl Pts',(-3.17058765355902,12.9692273118077,-8.00694725658));
#45686=CARTESIAN_POINT('Ctrl Pts',(-3.05948306544671,13.0341866726464,-8.0061819433219));
#45687=CARTESIAN_POINT('Ctrl Pts',(-2.94441965585415,13.0918749035054,-8.00527351756899));
#45688=CARTESIAN_POINT('Ctrl Pts',(-2.88336825523829,13.1224836548492,-8.00479151668994));
#45689=CARTESIAN_POINT('Ctrl Pts',(-2.82120321813055,13.1510457395272,-8.00426925202656));
#45690=CARTESIAN_POINT('Ctrl Pts',(-2.7580719769513,13.1774662231341,-8.00371006450633));
#45691=CARTESIAN_POINT('Ctrl Pts',(-2.64703765376743,13.2239341914599,-8.00272657350122));
#45692=CARTESIAN_POINT('Ctrl Pts',(-2.5330062475374,13.2637771321126,-8.00162880440515));
#45693=CARTESIAN_POINT('Ctrl Pts',(-2.41686575149847,13.2966459179422,-8.00044945974601));
#45694=CARTESIAN_POINT('Ctrl Pts',(-2.34251676502126,13.317687337572,-7.99969448552853));
#45695=CARTESIAN_POINT('Ctrl Pts',(-2.26730415745375,13.335871528974,-7.99890610901898));
#45696=CARTESIAN_POINT('Ctrl Pts',(-2.19146614940064,13.3511167596878,-7.9980931203695));
#45697=CARTESIAN_POINT('Ctrl Pts',(-2.08209765432325,13.3731024101957,-7.99692068259864));
#45698=CARTESIAN_POINT('Ctrl Pts',(-1.9714303709993,13.3889811469719,-7.9956970407022));
#45699=CARTESIAN_POINT('Ctrl Pts',(-1.86013185012544,13.3986735280725,-7.9944767393174));
#45700=CARTESIAN_POINT('Ctrl Pts',(-1.77390717570491,13.4061823646519,-7.9935313530825));
#45701=CARTESIAN_POINT('Ctrl Pts',(-1.68730334299757,13.4099772619015,-7.99258795667504));
#45702=CARTESIAN_POINT('Ctrl Pts',(-1.6006338528752,13.4099999330244,-7.99167226999386));
#45703=CARTESIAN_POINT('Ctrl Pts',(-1.60042256870131,13.4099999882924,-7.99167003771923));
#45704=CARTESIAN_POINT('Ctrl Pts',(-1.6002112841401,13.4100000211329,-7.99166780560954));
#45705=CARTESIAN_POINT('Ctrl Pts',(-1.59999999919616,13.4100000315449,-7.99166557366517));
#45706=CARTESIAN_POINT('Origin',(-1.59956987618261,12.9080292250358,-7.99148759263989));
#45707=CARTESIAN_POINT('Origin',(-1.655461430999,12.91,-7.991668980196));
#45708=CARTESIAN_POINT('',(-1.601056615238,13.40972231748,-8.00833023518));
#45709=CARTESIAN_POINT('',(2.2378444969905,13.41,-7.99166898016762));
#45710=CARTESIAN_POINT('',(-1.599999999195,13.41000000789,-7.991665573665));
#45711=CARTESIAN_POINT('Origin',(2.23784449531,12.91,-7.991668980205));
#45712=CARTESIAN_POINT('Origin',(-4.6,13.14,-16.1));
#45713=CARTESIAN_POINT('Ctrl Pts',(2.237584879956,13.40969719968,-8.009067185702));
#45714=CARTESIAN_POINT('Ctrl Pts',(2.237671468845,13.40969719968,-8.009067401558));
#45715=CARTESIAN_POINT('Ctrl Pts',(2.239198787813,13.40969719969,-8.009069273182));
#45716=CARTESIAN_POINT('Ctrl Pts',(2.24216509334,13.40969719965,-8.009006600652));
#45717=CARTESIAN_POINT('Ctrl Pts',(2.246462362136,13.40969719977,-8.008735050859));
#45718=CARTESIAN_POINT('Ctrl Pts',(2.24940692538,13.40969719947,-8.008431649983));
#45719=CARTESIAN_POINT('Ctrl Pts',(2.250913040081,13.40969719947,-8.0082427628));
#45720=CARTESIAN_POINT('Ctrl Pts',(2.251000426241,13.40969719947,-8.008231688651));
#45721=CARTESIAN_POINT('Ctrl Pts',(2.23759991999,13.40990301476,-8.003156059809));
#45722=CARTESIAN_POINT('Ctrl Pts',(2.237681494666,13.40990301476,-8.003156262383));
#45723=CARTESIAN_POINT('Ctrl Pts',(2.239120381434,13.40990301476,-8.003158014987));
#45724=CARTESIAN_POINT('Ctrl Pts',(2.241915466341,13.40990301475,-8.003099040079));
#45725=CARTESIAN_POINT('Ctrl Pts',(2.245971217721,13.40990301479,-8.002842672911));
#45726=CARTESIAN_POINT('Ctrl Pts',(2.248749025408,13.40990301469,-8.002556661255));
#45727=CARTESIAN_POINT('Ctrl Pts',(2.250172844306,13.40990301469,-8.002378138397));
#45728=CARTESIAN_POINT('Ctrl Pts',(2.250255466462,13.40990301469,-8.002367670494));
#45729=CARTESIAN_POINT('Ctrl Pts',(2.237614966948,13.41000391998,-7.997242212746));
#45730=CARTESIAN_POINT('Ctrl Pts',(2.237691525102,13.41000391998,-7.997242402031));
#45731=CARTESIAN_POINT('Ctrl Pts',(2.239041938962,13.41000391998,-7.99724403556));
#45732=CARTESIAN_POINT('Ctrl Pts',(2.241665724427,13.41000391998,-7.997188759977));
#45733=CARTESIAN_POINT('Ctrl Pts',(2.245479847208,13.41000391997,-7.996947582423));
#45734=CARTESIAN_POINT('Ctrl Pts',(2.248090822574,13.41000391998,-7.996678967993));
#45735=CARTESIAN_POINT('Ctrl Pts',(2.249432307784,13.41000391998,-7.996510814231));
#45736=CARTESIAN_POINT('Ctrl Pts',(2.249510163744,13.41000391998,-7.996500952852));
#45737=CARTESIAN_POINT('Ctrl Pts',(2.237630016093,13.40999988357,-7.991327506279));
#45738=CARTESIAN_POINT('Ctrl Pts',(2.237701556996,13.40999988357,-7.991327682274));
#45739=CARTESIAN_POINT('Ctrl Pts',(2.238963485089,13.40999988357,-7.991329196711));
#45740=CARTESIAN_POINT('Ctrl Pts',(2.24141594622,13.40999988357,-7.991277620989));
#45741=CARTESIAN_POINT('Ctrl Pts',(2.24498840529,13.40999988357,-7.991051635257));
#45742=CARTESIAN_POINT('Ctrl Pts',(2.247432524089,13.40999988357,-7.990800420582));
#45743=CARTESIAN_POINT('Ctrl Pts',(2.248691663647,13.40999988357,-7.990642637421));
#45744=CARTESIAN_POINT('Ctrl Pts',(2.248764752717,13.40999988357,-7.990633382656));
#45745=CARTESIAN_POINT('',(2.24859000193236,13.4099999999984,-7.99099916821552));
#45746=CARTESIAN_POINT('Origin',(2.24555455540351,13.4100000000148,-7.97888459757615));
#45747=CARTESIAN_POINT('Origin',(2.248590003289,12.90999965096,-7.990999166063));
#45748=CARTESIAN_POINT('Ctrl Pts',(2.278075340984,13.15718819574,-8.425336826683));
#45749=CARTESIAN_POINT('Ctrl Pts',(2.286140753447,13.15718819272,-8.424319735027));
#45750=CARTESIAN_POINT('Ctrl Pts',(2.35388291064,13.15718818874,-8.415807036881));
#45751=CARTESIAN_POINT('Ctrl Pts',(2.483820341006,13.15718844103,-8.399846720424));
#45752=CARTESIAN_POINT('Ctrl Pts',(2.655713713522,13.15718835356,-8.378231657577));
#45753=CARTESIAN_POINT('Ctrl Pts',(2.814178657447,13.15718837421,-8.358041618531));
#45754=CARTESIAN_POINT('Ctrl Pts',(2.958673491815,13.15718836941,-8.339207395949));
#45755=CARTESIAN_POINT('Ctrl Pts',(3.089582223425,13.15718837051,-8.321679161787));
#45756=CARTESIAN_POINT('Ctrl Pts',(3.208956769851,13.15718837026,-8.305254092409));
#45757=CARTESIAN_POINT('Ctrl Pts',(3.320120581901,13.15718837032,-8.289476173224));
#45758=CARTESIAN_POINT('Ctrl Pts',(3.426484163409,13.1571883703,-8.273855324399));
#45759=CARTESIAN_POINT('Ctrl Pts',(3.530967273143,13.15718837031,-8.257942363676));
#45760=CARTESIAN_POINT('Ctrl Pts',(3.635235631839,13.15718837031,-8.24140149434));
#45761=CARTESIAN_POINT('Ctrl Pts',(3.740376492139,13.15718837031,-8.223909889447));
#45762=CARTESIAN_POINT('Ctrl Pts',(3.848559055294,13.1571883703,-8.204917648829));
#45763=CARTESIAN_POINT('Ctrl Pts',(3.963755801124,13.15718837033,-8.183374059621));
#45764=CARTESIAN_POINT('Ctrl Pts',(4.05254074859,13.15718837025,-8.165401404086));
#45765=CARTESIAN_POINT('Ctrl Pts',(4.103430937961,13.15718837026,-8.154442560125));
#45766=CARTESIAN_POINT('Ctrl Pts',(4.112378765212,13.15718837026,-8.152494402827));
#45767=CARTESIAN_POINT('Ctrl Pts',(2.265371289856,13.33424242924,-8.325443171538));
#45768=CARTESIAN_POINT('Ctrl Pts',(2.273525484251,13.33424242834,-8.324414990892));
#45769=CARTESIAN_POINT('Ctrl Pts',(2.341879625082,13.33424242715,-8.315825860922));
#45770=CARTESIAN_POINT('Ctrl Pts',(2.471265663326,13.33424250275,-8.299934497874));
#45771=CARTESIAN_POINT('Ctrl Pts',(2.643103570828,13.33424247653,-8.278326401));
#45772=CARTESIAN_POINT('Ctrl Pts',(2.801329586393,13.33424248272,-8.258166691294));
#45773=CARTESIAN_POINT('Ctrl Pts',(2.945496865447,13.33424248129,-8.239375100594));
#45774=CARTESIAN_POINT('Ctrl Pts',(3.076049794216,13.33424248162,-8.221894455168));
#45775=CARTESIAN_POINT('Ctrl Pts',(3.195038588614,13.33424248154,-8.20552238341));
#45776=CARTESIAN_POINT('Ctrl Pts',(3.305742731698,13.33424248156,-8.189809589949));
#45777=CARTESIAN_POINT('Ctrl Pts',(3.411596899129,13.33424248155,-8.174263494606));
#45778=CARTESIAN_POINT('Ctrl Pts',(3.51551924109,13.33424248155,-8.158435800941));
#45779=CARTESIAN_POINT('Ctrl Pts',(3.619104977514,13.33424248155,-8.142002990221));
#45780=CARTESIAN_POINT('Ctrl Pts',(3.723429040626,13.33424248155,-8.124647006269));
#45781=CARTESIAN_POINT('Ctrl Pts',(3.830626058125,13.33424248155,-8.105827356883));
#45782=CARTESIAN_POINT('Ctrl Pts',(3.944552759001,13.33424248156,-8.08452044384));
#45783=CARTESIAN_POINT('Ctrl Pts',(4.032102539776,13.33424248154,-8.066796360282));
#45784=CARTESIAN_POINT('Ctrl Pts',(4.082151021483,13.33424248154,-8.056018666363));
#45785=CARTESIAN_POINT('Ctrl Pts',(4.09094646625,13.33424248154,-8.054103647986));
#45786=CARTESIAN_POINT('Ctrl Pts',(2.242543304394,13.42776922549,-8.145943665092));
#45787=CARTESIAN_POINT('Ctrl Pts',(2.250857031574,13.4277692257,-8.144895558574));
#45788=CARTESIAN_POINT('Ctrl Pts',(2.320310849465,13.42776922598,-8.136169087801));
#45789=CARTESIAN_POINT('Ctrl Pts',(2.448706087905,13.42776920825,-8.120401627548));
#45790=CARTESIAN_POINT('Ctrl Pts',(2.620444329994,13.4277692144,-8.098806047871));
#45791=CARTESIAN_POINT('Ctrl Pts',(2.778241013758,13.42776921295,-8.078700837139));
#45792=CARTESIAN_POINT('Ctrl Pts',(2.921819706712,13.42776921328,-8.059985851922));
#45793=CARTESIAN_POINT('Ctrl Pts',(3.051733291228,13.42776921321,-8.042590718981));
#45794=CARTESIAN_POINT('Ctrl Pts',(3.170028925497,13.42776921323,-8.026313878963));
#45795=CARTESIAN_POINT('Ctrl Pts',(3.279907086667,13.42776921322,-8.010718110303));
#45796=CARTESIAN_POINT('Ctrl Pts',(3.384845884895,13.42776921322,-7.995306339941));
#45797=CARTESIAN_POINT('Ctrl Pts',(3.487760579892,13.42776921322,-7.979631863162));
#45798=CARTESIAN_POINT('Ctrl Pts',(3.590119708273,13.42776921322,-7.963393223616));
#45799=CARTESIAN_POINT('Ctrl Pts',(3.692976063632,13.42776921322,-7.946280937741));
#45800=CARTESIAN_POINT('Ctrl Pts',(3.798402148244,13.42776921322,-7.927771418573));
#45801=CARTESIAN_POINT('Ctrl Pts',(3.910046697746,13.42776921322,-7.906889790346));
#45802=CARTESIAN_POINT('Ctrl Pts',(3.995377000107,13.42776921323,-7.889612367263));
#45803=CARTESIAN_POINT('Ctrl Pts',(4.043913012279,13.42776921323,-7.879160182937));
#45804=CARTESIAN_POINT('Ctrl Pts',(4.052434640046,13.42776921323,-7.877304712087));
#45805=CARTESIAN_POINT('Ctrl Pts',(2.216973445714,13.40752410553,-7.94488444239));
#45806=CARTESIAN_POINT('Ctrl Pts',(2.225465867189,13.4075241055,-7.9438140167));
#45807=CARTESIAN_POINT('Ctrl Pts',(2.296151444539,13.40752410546,-7.934933709098));
#45808=CARTESIAN_POINT('Ctrl Pts',(2.423436878043,13.40752410793,-7.919305033624));
#45809=CARTESIAN_POINT('Ctrl Pts',(2.595063483889,13.40752410708,-7.897723474586));
#45810=CARTESIAN_POINT('Ctrl Pts',(2.752379268737,13.40752410728,-7.87767930871));
#45811=CARTESIAN_POINT('Ctrl Pts',(2.895298680413,13.40752410723,-7.859050130073));
#45812=CARTESIAN_POINT('Ctrl Pts',(3.024496128928,13.40752410724,-7.841750780536));
#45813=CARTESIAN_POINT('Ctrl Pts',(3.142015347489,13.40752410724,-7.82558061056));
#45814=CARTESIAN_POINT('Ctrl Pts',(3.250968317917,13.40752410724,-7.810115922569));
#45815=CARTESIAN_POINT('Ctrl Pts',(3.354881801791,13.40752410724,-7.794854610983));
#45816=CARTESIAN_POINT('Ctrl Pts',(3.456667821175,13.40752410724,-7.779351753998));
#45817=CARTESIAN_POINT('Ctrl Pts',(3.557653013413,13.40752410724,-7.763330607559));
#45818=CARTESIAN_POINT('Ctrl Pts',(3.65886537439,13.40752410724,-7.746491290379));
#45819=CARTESIAN_POINT('Ctrl Pts',(3.762307819065,13.40752410724,-7.728329151223));
#45820=CARTESIAN_POINT('Ctrl Pts',(3.871396107604,13.40752410724,-7.707923888843));
#45821=CARTESIAN_POINT('Ctrl Pts',(3.954240349621,13.40752410724,-7.6911467747));
#45822=CARTESIAN_POINT('Ctrl Pts',(4.001082229283,13.40752410724,-7.68105919698));
#45823=CARTESIAN_POINT('Ctrl Pts',(4.009297151845,13.40752410724,-7.679270425919));
#45824=CARTESIAN_POINT('Ctrl Pts',(2.25070093407567,13.4097088394601,-8.00792902136249));
#45825=CARTESIAN_POINT('Ctrl Pts',(2.25070142686699,13.4097088356214,-8.00792907293275));
#45826=CARTESIAN_POINT('Ctrl Pts',(2.25070191965817,13.4097088317827,-8.007929124503));
#45827=CARTESIAN_POINT('Ctrl Pts',(2.25070241244921,13.4097088279439,-8.00792917607324));
#45828=CARTESIAN_POINT('Ctrl Pts',(2.27794362486571,13.4094966216791,-8.01077995025102));
#45829=CARTESIAN_POINT('Ctrl Pts',(2.30476118430153,13.4091718850223,-8.01360907290453));
#45830=CARTESIAN_POINT('Ctrl Pts',(2.33118325787516,13.4087450676421,-8.0163942422403));
#45831=CARTESIAN_POINT('Ctrl Pts',(2.35999938229403,13.408279577199,-8.01943177015739));
#45832=CARTESIAN_POINT('Ctrl Pts',(2.38834468584762,13.4076926978792,-8.02241701648861));
#45833=CARTESIAN_POINT('Ctrl Pts',(2.41619478593185,13.4069965329008,-8.02533510968307));
#45834=CARTESIAN_POINT('Ctrl Pts',(2.42477884851803,13.406781958313,-8.02623453534179));
#45835=CARTESIAN_POINT('Ctrl Pts',(2.43331548901635,13.4065569900252,-8.02712767440583));
#45836=CARTESIAN_POINT('Ctrl Pts',(2.44180307769693,13.4063219516077,-8.02801432599494));
#45837=CARTESIAN_POINT('Ctrl Pts',(2.48538791449942,13.4051149997328,-8.03256739357004));
#45838=CARTESIAN_POINT('Ctrl Pts',(2.52773990785003,13.4036436248157,-8.03693549898386));
#45839=CARTESIAN_POINT('Ctrl Pts',(2.56891103034342,13.4019523661277,-8.04113042432577));
#45840=CARTESIAN_POINT('Ctrl Pts',(2.58562190995613,13.4012659039033,-8.04283309571599));
#45841=CARTESIAN_POINT('Ctrl Pts',(2.60213891571461,13.4005431591336,-8.04450719695673));
#45842=CARTESIAN_POINT('Ctrl Pts',(2.61846777138499,13.3997868594101,-8.04615339980819));
#45843=CARTESIAN_POINT('Ctrl Pts',(2.67502654508264,13.397167240144,-8.05185540467708));
#45844=CARTESIAN_POINT('Ctrl Pts',(2.7293135332922,13.3941445132716,-8.05722302128092));
#45845=CARTESIAN_POINT('Ctrl Pts',(2.78107106661417,13.3908432614605,-8.06222510384196));
#45846=CARTESIAN_POINT('Ctrl Pts',(2.83282859993615,13.3875420096493,-8.06722718640301));
#45847=CARTESIAN_POINT('Ctrl Pts',(2.88205673194293,13.3839633579127,-8.07186414347928));
#45848=CARTESIAN_POINT('Ctrl Pts',(2.92878849763644,13.380217612112,-8.07613720207639));
#45849=CARTESIAN_POINT('Ctrl Pts',(2.97552026332994,13.3764718663113,-8.0804102606735));
#45850=CARTESIAN_POINT('Ctrl Pts',(3.01975576917847,13.372561337648,-8.0843202277642));
#45851=CARTESIAN_POINT('Ctrl Pts',(3.06193261059204,13.3685399555076,-8.08792588768494));
#45852=CARTESIAN_POINT('Ctrl Pts',(3.10410945200556,13.3645185733671,-8.09153154760569));
#45853=CARTESIAN_POINT('Ctrl Pts',(3.14422766443156,13.3603870338277,-8.09483316581655));
#45854=CARTESIAN_POINT('Ctrl Pts',(3.18291144942371,13.3561410864198,-8.09789654337337));
#45855=CARTESIAN_POINT('Ctrl Pts',(3.22159523441592,13.3518951390118,-8.1009599209302));
#45856=CARTESIAN_POINT('Ctrl Pts',(3.25884458823385,13.3475347577083,-8.10378503371712));
#45857=CARTESIAN_POINT('Ctrl Pts',(3.29532012225226,13.3430188597012,-8.10641940803316));
#45858=CARTESIAN_POINT('Ctrl Pts',(3.33179565627067,13.3385029616941,-8.10905378234921));
#45859=CARTESIAN_POINT('Ctrl Pts',(3.36749736453129,13.3338314262824,-8.11149737027822));
#45860=CARTESIAN_POINT('Ctrl Pts',(3.40302221319701,13.3289360949713,-8.11378048183653));
#45861=CARTESIAN_POINT('Ctrl Pts',(3.43854706186268,13.3240407636603,-8.11606359339485));
#45862=CARTESIAN_POINT('Ctrl Pts',(3.47389500089121,13.3189213316682,-8.11818593114135));
#45863=CARTESIAN_POINT('Ctrl Pts',(3.50947489449939,13.3134962224709,-8.12015680508066));
#45864=CARTESIAN_POINT('Ctrl Pts',(3.54505478810762,13.3080711132736,-8.12212767901997));
#45865=CARTESIAN_POINT('Ctrl Pts',(3.58086623287029,13.3023365335503,-8.12394444876931));
#45866=CARTESIAN_POINT('Ctrl Pts',(3.61654311190259,13.2963278639491,-8.12555585329945));
#45867=CARTESIAN_POINT('Ctrl Pts',(3.65221999093489,13.2903191943479,-8.12716725782958));
#45868=CARTESIAN_POINT('Ctrl Pts',(3.68776288736539,13.2840406765724,-8.12857684740129));
#45869=CARTESIAN_POINT('Ctrl Pts',(3.72363861368408,13.2773820882215,-8.12976222303873));
#45870=CARTESIAN_POINT('Ctrl Pts',(3.75236529817654,13.2720503727039,-8.13071138603656));
#45871=CARTESIAN_POINT('Ctrl Pts',(3.78130602030519,13.2664765012613,-8.13151659935786));
#45872=CARTESIAN_POINT('Ctrl Pts',(3.81091149710654,13.2605331055368,-8.13215612642615));
#45873=CARTESIAN_POINT('Ctrl Pts',(3.81827923883093,13.2590540074308,-8.13231528178435));
#45874=CARTESIAN_POINT('Ctrl Pts',(3.82568817679555,13.2575519470327,-8.13246394080603));
#45875=CARTESIAN_POINT('Ctrl Pts',(3.83314531426046,13.2560248155579,-8.13260127222032));
#45876=CARTESIAN_POINT('Ctrl Pts',(3.85778472246543,13.2509789630487,-8.13305503410844));
#45877=CARTESIAN_POINT('Ctrl Pts',(3.88295097129545,13.2456623141355,-8.13338659784483));
#45878=CARTESIAN_POINT('Ctrl Pts',(3.90899354542653,13.2399434928449,-8.13356657373334));
#45879=CARTESIAN_POINT('Ctrl Pts',(3.92250390029888,13.2369766853128,-8.13365994154369));
#45880=CARTESIAN_POINT('Ctrl Pts',(3.93625018293504,13.2339014430577,-8.13371178145361));
#45881=CARTESIAN_POINT('Ctrl Pts',(3.95028185158443,13.2306982824754,-8.13371247872827));
#45882=CARTESIAN_POINT('Ctrl Pts',(3.98739045364131,13.2222271010112,-8.13371432276327));
#45883=CARTESIAN_POINT('Ctrl Pts',(4.02649097892153,13.212856018128,-8.13336322175475));
#45884=CARTESIAN_POINT('Ctrl Pts',(4.06694679202954,13.202515578365,-8.13245141709027));
#45885=CARTESIAN_POINT('Ctrl Pts',(4.07127546077212,13.2014091777035,-8.13235385631848));
#45886=CARTESIAN_POINT('Ctrl Pts',(4.07561965073057,13.2002917055087,-8.13224983579308));
#45887=CARTESIAN_POINT('Ctrl Pts',(4.07997858462006,13.1991630971381,-8.13213907538709));
#45888=CARTESIAN_POINT('',(3.99496190950109,13.4099999999998,-7.73319438214748));
#45889=CARTESIAN_POINT('Ctrl Pts',(2.24859000168769,13.4099999999975,-7.99099916626274));
#45890=CARTESIAN_POINT('Ctrl Pts',(2.30138639266896,13.409999999997,-7.98438415500106));
#45891=CARTESIAN_POINT('Ctrl Pts',(2.35261444485792,13.4099999999934,-7.97807171786754));
#45892=CARTESIAN_POINT('Ctrl Pts',(2.40222264371354,13.4099999999962,-7.97192548958838));
#45893=CARTESIAN_POINT('Ctrl Pts',(2.41299850134135,13.4099999999968,-7.9705904102585));
#45894=CARTESIAN_POINT('Ctrl Pts',(2.42369792263813,13.4099999999977,-7.96926336922857));
#45895=CARTESIAN_POINT('Ctrl Pts',(2.43432037163303,13.4099999999979,-7.96794328908766));
#45896=CARTESIAN_POINT('Ctrl Pts',(2.493845504109,13.4099999999988,-7.96054594170533));
#45897=CARTESIAN_POINT('Ctrl Pts',(2.55095381197397,13.4100000000006,-7.95335804203067));
#45898=CARTESIAN_POINT('Ctrl Pts',(2.60584016881678,13.4100000000012,-7.94640684095368));
#45899=CARTESIAN_POINT('Ctrl Pts',(2.66072652565963,13.4100000000018,-7.93945563987667));
#45900=CARTESIAN_POINT('Ctrl Pts',(2.71339093148032,13.4100000000012,-7.93274113739734));
#45901=CARTESIAN_POINT('Ctrl Pts',(2.76354134874866,13.4100000000003,-7.92627486699083));
#45902=CARTESIAN_POINT('Ctrl Pts',(2.813691766017,13.4099999999995,-7.91980859658434));
#45903=CARTESIAN_POINT('Ctrl Pts',(2.861328194733,13.4099999999983,-7.91359055825067));
#45904=CARTESIAN_POINT('Ctrl Pts',(2.90650757886068,13.4099999999979,-7.90761729845183));
#45905=CARTESIAN_POINT('Ctrl Pts',(2.95168696298835,13.4099999999975,-7.901644038653));
#45906=CARTESIAN_POINT('Ctrl Pts',(2.99440930252771,13.4099999999978,-7.895915557389));
#45907=CARTESIAN_POINT('Ctrl Pts',(3.03509758705189,13.4099999999984,-7.89038857294066));
#45908=CARTESIAN_POINT('Ctrl Pts',(3.07578587157602,13.4099999999989,-7.88486158849233));
#45909=CARTESIAN_POINT('Ctrl Pts',(3.11444010108498,13.4099999999997,-7.87953610085967));
#45910=CARTESIAN_POINT('Ctrl Pts',(3.15164810591261,13.4099999999997,-7.87433282904934));
#45911=CARTESIAN_POINT('Ctrl Pts',(3.1888561107403,13.4099999999998,-7.869129557239));
#45912=CARTESIAN_POINT('Ctrl Pts',(3.22461789088665,13.4099999999993,-7.864048501251));
#45913=CARTESIAN_POINT('Ctrl Pts',(3.25957932564517,13.409999999999,-7.85899818299083));
#45914=CARTESIAN_POINT('Ctrl Pts',(3.29454076040368,13.4099999999987,-7.85394786473066));
#45915=CARTESIAN_POINT('Ctrl Pts',(3.32870184977437,13.4099999999986,-7.84892828419833));
#45916=CARTESIAN_POINT('Ctrl Pts',(3.36263775530638,13.4099999999986,-7.84385152101549));
#45917=CARTESIAN_POINT('Ctrl Pts',(3.39657366083835,13.4099999999986,-7.83877475783267));
#45918=CARTESIAN_POINT('Ctrl Pts',(3.43028438253165,13.4099999999986,-7.83364081199933));
#45919=CARTESIAN_POINT('Ctrl Pts',(3.46411762057695,13.4099999999986,-7.82838032187151));
#45920=CARTESIAN_POINT('Ctrl Pts',(3.4979508586223,13.4099999999986,-7.82311983174367));
#45921=CARTESIAN_POINT('Ctrl Pts',(3.53190661301965,13.4099999999986,-7.81773279732134));
#45922=CARTESIAN_POINT('Ctrl Pts',(3.56562768693499,13.4099999999986,-7.81225344182417));
#45923=CARTESIAN_POINT('Ctrl Pts',(3.59934876085033,13.4099999999986,-7.806774086327));
#45924=CARTESIAN_POINT('Ctrl Pts',(3.63283515428367,13.4099999999986,-7.801202409755));
#45925=CARTESIAN_POINT('Ctrl Pts',(3.66649691169818,13.4099999999986,-7.79544915546967));
#45926=CARTESIAN_POINT('Ctrl Pts',(3.70015866911268,13.4099999999986,-7.78969590118433));
#45927=CARTESIAN_POINT('Ctrl Pts',(3.73399579050837,13.4099999999986,-7.78376106918566));
#45928=CARTESIAN_POINT('Ctrl Pts',(3.76882549197522,13.4099999999986,-7.77745371488882));
#45929=CARTESIAN_POINT('Ctrl Pts',(3.79950885807498,13.4099999999986,-7.77189722566095));
#45930=CARTESIAN_POINT('Ctrl Pts',(3.83096170362461,13.4099999999984,-7.76605064457506));
#45931=CARTESIAN_POINT('Ctrl Pts',(3.86372916609635,13.4099999999989,-7.75974007885942));
#45932=CARTESIAN_POINT('Ctrl Pts',(3.86815713166221,13.409999999999,-7.75888731317107));
#45933=CARTESIAN_POINT('Ctrl Pts',(3.87260905245847,13.409999999999,-7.75802601485461));
#45934=CARTESIAN_POINT('Ctrl Pts',(3.8770862219782,13.4099999999991,-7.75715569492626));
#45935=CARTESIAN_POINT('Ctrl Pts',(3.91190350686239,13.4099999999994,-7.75038754001229));
#45936=CARTESIAN_POINT('Ctrl Pts',(3.94825130413398,13.4100000000001,-7.7430782376179));
#45937=CARTESIAN_POINT('Ctrl Pts',(3.98588409196118,13.4100000000003,-7.73512119656737));
#45938=CARTESIAN_POINT('Ctrl Pts',(3.98890128591575,13.4100000000003,-7.73448324393244));
#45939=CARTESIAN_POINT('Ctrl Pts',(3.99192671687108,13.4100000000003,-7.73384111172618));
#45940=CARTESIAN_POINT('Ctrl Pts',(3.99496024621,13.4100000000004,-7.733194736626));
#45941=CARTESIAN_POINT('Origin',(3.994963573291,12.9099999999,-7.733194027536));
#45942=CARTESIAN_POINT('Ctrl Pts',(3.739203750449,12.9180458811,-8.891362475312));
#45943=CARTESIAN_POINT('Ctrl Pts',(3.73146660992,12.92315978193,-8.889112682545));
#45944=CARTESIAN_POINT('Ctrl Pts',(3.643055660205,12.98106721331,-8.862733317068));
#45945=CARTESIAN_POINT('Ctrl Pts',(3.462068739991,13.08744838347,-8.79359290624));
#45946=CARTESIAN_POINT('Ctrl Pts',(3.185389292547,13.21644881828,-8.656430471233));
#45947=CARTESIAN_POINT('Ctrl Pts',(2.87990332086,13.32045340503,-8.478983152178));
#45948=CARTESIAN_POINT('Ctrl Pts',(2.552976861821,13.38969339755,-8.270214273238));
#45949=CARTESIAN_POINT('Ctrl Pts',(2.32535497479,13.40826165724,-8.117787218622));
#45950=CARTESIAN_POINT('Ctrl Pts',(2.20750057804,13.40989482807,-8.038538555201));
#45951=CARTESIAN_POINT('Ctrl Pts',(2.203441286853,13.40994161843,-8.03580865607));
#45952=CARTESIAN_POINT('Ctrl Pts',(3.803158684465,12.89472761344,-8.566360772745));
#45953=CARTESIAN_POINT('Ctrl Pts',(3.796388461278,12.89934439347,-8.564337486772));
#45954=CARTESIAN_POINT('Ctrl Pts',(3.718914974065,12.95177154022,-8.540571264521));
#45955=CARTESIAN_POINT('Ctrl Pts',(3.55770110028,13.05139891642,-8.477273832003));
#45956=CARTESIAN_POINT('Ctrl Pts',(3.304530173815,13.17905954386,-8.348467736982));
#45957=CARTESIAN_POINT('Ctrl Pts',(3.017846351306,13.2886957054,-8.178410744612));
#45958=CARTESIAN_POINT('Ctrl Pts',(2.703644178881,13.36890354346,-7.974894308892));
#45959=CARTESIAN_POINT('Ctrl Pts',(2.479858161105,13.39690127167,-7.824049236676));
#45960=CARTESIAN_POINT('Ctrl Pts',(2.362668879712,13.40348799783,-7.745039942689));
#45961=CARTESIAN_POINT('Ctrl Pts',(2.358630951334,13.40370547786,-7.742317582132));
#45962=CARTESIAN_POINT('Ctrl Pts',(3.942747596141,13.00246573178,-8.284993708305));
#45963=CARTESIAN_POINT('Ctrl Pts',(3.9364609035,13.00688490927,-8.283135183149));
#45964=CARTESIAN_POINT('Ctrl Pts',(3.864406309965,13.05720985831,-8.261272807038));
#45965=CARTESIAN_POINT('Ctrl Pts',(3.711790014713,13.15598759483,-8.202287599445));
#45966=CARTESIAN_POINT('Ctrl Pts',(3.465401337309,13.28883036506,-8.079461983691));
#45967=CARTESIAN_POINT('Ctrl Pts',(3.17947995917,13.40871254137,-7.914244697299));
#45968=CARTESIAN_POINT('Ctrl Pts',(2.859189437579,13.50224374698,-7.71339622914));
#45969=CARTESIAN_POINT('Ctrl Pts',(2.626512259222,13.53963961786,-7.562459200681));
#45970=CARTESIAN_POINT('Ctrl Pts',(2.503505827146,13.55074997021,-7.482859510525));
#45971=CARTESIAN_POINT('Ctrl Pts',(2.499266117154,13.55112284234,-7.48011615425));
#45972=CARTESIAN_POINT('Ctrl Pts',(4.126573294533,13.21702712022,-8.110548081366));
#45973=CARTESIAN_POINT('Ctrl Pts',(4.120177986995,13.22159265941,-8.10875551204));
#45974=CARTESIAN_POINT('Ctrl Pts',(4.046804867636,13.27366633679,-8.087659460274));
#45975=CARTESIAN_POINT('Ctrl Pts',(3.889676863125,13.37768969408,-8.030485792242));
#45976=CARTESIAN_POINT('Ctrl Pts',(3.631818657962,13.52107095805,-7.909919629098));
#45977=CARTESIAN_POINT('Ctrl Pts',(3.32844852574,13.65350899285,-7.745902851738));
#45978=CARTESIAN_POINT('Ctrl Pts',(2.984626447899,13.75972231478,-7.544537779912));
#45979=CARTESIAN_POINT('Ctrl Pts',(2.73233093329,13.80437111482,-7.391855539927));
#45980=CARTESIAN_POINT('Ctrl Pts',(2.598333513568,13.81855768255,-7.310968483515));
#45981=CARTESIAN_POINT('Ctrl Pts',(2.593714263493,13.81903569747,-7.308180319716));
#45982=CARTESIAN_POINT('Ctrl Pts',(4.049148071614,13.05937723215,-8.208772713831));
#45983=CARTESIAN_POINT('Ctrl Pts',(4.064894678394,13.05937723208,-8.205946355611));
#45984=CARTESIAN_POINT('Ctrl Pts',(4.100886611793,13.05937723204,-8.198815606686));
#45985=CARTESIAN_POINT('Ctrl Pts',(4.153076125832,13.05937723217,-8.186493455414));
#45986=CARTESIAN_POINT('Ctrl Pts',(4.208582748717,13.05937723213,-8.171878615881));
#45987=CARTESIAN_POINT('Ctrl Pts',(4.264585919179,13.05937723214,-8.156133113951));
#45988=CARTESIAN_POINT('Ctrl Pts',(4.323333002791,13.05937723213,-8.139058904706));
#45989=CARTESIAN_POINT('Ctrl Pts',(4.372134051461,13.05937723214,-8.124730690516));
#45990=CARTESIAN_POINT('Ctrl Pts',(4.40143305218,13.05937723213,-8.116204585805));
#45991=CARTESIAN_POINT('Ctrl Pts',(4.410246257208,13.05937723213,-8.113652741193));
#45992=CARTESIAN_POINT('Ctrl Pts',(4.036444039793,13.29564346116,-8.135894285009));
#45993=CARTESIAN_POINT('Ctrl Pts',(4.051118792472,13.29564346114,-8.133268259165));
#45994=CARTESIAN_POINT('Ctrl Pts',(4.084982381981,13.29564346112,-8.126565695879));
#45995=CARTESIAN_POINT('Ctrl Pts',(4.135046057456,13.29564346117,-8.114753411066));
#45996=CARTESIAN_POINT('Ctrl Pts',(4.189047146895,13.29564346115,-8.100538275903));
#45997=CARTESIAN_POINT('Ctrl Pts',(4.24416519593,13.29564346116,-8.085043648133));
#45998=CARTESIAN_POINT('Ctrl Pts',(4.302523744979,13.29564346116,-8.068083020918));
#45999=CARTESIAN_POINT('Ctrl Pts',(4.351341025745,13.29564346116,-8.053750009283));
#46000=CARTESIAN_POINT('Ctrl Pts',(4.380795426626,13.29564346116,-8.045178569442));
#46001=CARTESIAN_POINT('Ctrl Pts',(4.389668354159,13.29564346116,-8.042609311642));
#46002=CARTESIAN_POINT('Ctrl Pts',(4.000966626673,13.43213122111,-7.9323732168));
#46003=CARTESIAN_POINT('Ctrl Pts',(4.012648108297,13.43213122111,-7.930306641258));
#46004=CARTESIAN_POINT('Ctrl Pts',(4.040568062233,13.43213122111,-7.9247998337));
#46005=CARTESIAN_POINT('Ctrl Pts',(4.084695098534,13.4321312211,-7.914411407335));
#46006=CARTESIAN_POINT('Ctrl Pts',(4.134491819411,13.43213122111,-7.901312490802));
#46007=CARTESIAN_POINT('Ctrl Pts',(4.187138069023,13.43213122111,-7.886518456859));
#46008=CARTESIAN_POINT('Ctrl Pts',(4.244411592357,13.43213122111,-7.869875020014));
#46009=CARTESIAN_POINT('Ctrl Pts',(4.293274203046,13.43213122111,-7.855528610986));
#46010=CARTESIAN_POINT('Ctrl Pts',(4.323162576058,13.43213122111,-7.846830567784));
#46011=CARTESIAN_POINT('Ctrl Pts',(4.332202285286,13.43213122111,-7.844212681733));
#46012=CARTESIAN_POINT('Ctrl Pts',(3.958653872581,13.40752410724,-7.689640273377));
#46013=CARTESIAN_POINT('Ctrl Pts',(3.966765377397,13.40752410724,-7.688240935973));
#46014=CARTESIAN_POINT('Ctrl Pts',(3.987596550943,13.40752410724,-7.684160267291));
#46015=CARTESIAN_POINT('Ctrl Pts',(4.024643151232,13.40752410724,-7.67547003048));
#46016=CARTESIAN_POINT('Ctrl Pts',(4.069425458784,13.40752410724,-7.663702391521));
#46017=CARTESIAN_POINT('Ctrl Pts',(4.119123673802,13.40752410724,-7.649743932995));
#46018=CARTESIAN_POINT('Ctrl Pts',(4.175103122337,13.40752410724,-7.633478798764));
#46019=CARTESIAN_POINT('Ctrl Pts',(4.224019796546,13.40752410724,-7.619116411102));
#46020=CARTESIAN_POINT('Ctrl Pts',(4.254425753972,13.40752410724,-7.610267372199));
#46021=CARTESIAN_POINT('Ctrl Pts',(4.263664378291,13.40752410724,-7.607591488817));
#46022=CARTESIAN_POINT('Ctrl Pts',(3.99496190950166,13.41,-7.73319438213609));
#46023=CARTESIAN_POINT('Ctrl Pts',(4.00851215418661,13.41,-7.730306466485));
#46024=CARTESIAN_POINT('Ctrl Pts',(4.03662735941919,13.41,-7.72369650207739));
#46025=CARTESIAN_POINT('Ctrl Pts',(4.080565611154,13.41,-7.7121736621));
#46026=CARTESIAN_POINT('Ctrl Pts',(4.130494585122,13.41,-7.698184085465));
#46027=CARTESIAN_POINT('Ctrl Pts',(4.186228983442,13.41,-7.682004638378));
#46028=CARTESIAN_POINT('Ctrl Pts',(4.227999624963,13.41,-7.66974072988));
#46029=CARTESIAN_POINT('Ctrl Pts',(4.24999999921,13.41,-7.66332099539));
#46030=CARTESIAN_POINT('Origin',(-4.6,13.41,-8.));
#46031=CARTESIAN_POINT('',(-1.599999999708,13.41,7.5));
#46032=CARTESIAN_POINT('',(4.249999999336,13.41,7.5));
#46033=CARTESIAN_POINT('',(-1.599999999708,13.41,7.5));
#46034=CARTESIAN_POINT('Origin',(4.345740905029,12.91,7.5));
#46035=CARTESIAN_POINT('Origin',(-1.6,12.91,7.5));
#46036=CARTESIAN_POINT('Origin',(-1.6,10.41,7.5));
#46037=CARTESIAN_POINT('Origin',(-1.6,10.41,7.5));
#46038=CARTESIAN_POINT('Origin',(-4.1,10.41,7.5));
#46039=CARTESIAN_POINT('Origin',(-4.1,10.465461431,7.5));
#46040=CARTESIAN_POINT('Origin',(-4.1,1.41,7.5));
#46041=CARTESIAN_POINT('Origin',(-4.1,1.41,0.));
#46042=CARTESIAN_POINT('Origin',(-4.1,1.41,-7.5));
#46043=CARTESIAN_POINT('Origin',(-4.1,1.343139657048,-7.5));
#46044=CARTESIAN_POINT('Origin',(-1.6,10.41,39.41676));
#46045=CARTESIAN_POINT('Origin',(-4.1,-39.88672151809,-7.988586197742));
#46046=CARTESIAN_POINT('Origin',(4.75,1.348669871537,7.5));
#52143=UNCERTAINTY_MEASURE_WITH_UNIT(LENGTH_MEASURE(0.01),#52165,
'DISTANCE_ACCURACY_VALUE',
'Maximum model space distance between geometric entities at asserted c
onnectivities');
#52149=UNCERTAINTY_MEASURE_WITH_UNIT(LENGTH_MEASURE(0.01),#52165,
'DISTANCE_ACCURACY_VALUE',
'Maximum model space distance between geometric entities at asserted c
onnectivities');
#52158=(
GEOMETRIC_REPRESENTATION_CONTEXT(3)
GLOBAL_UNCERTAINTY_ASSIGNED_CONTEXT((#52143))
GLOBAL_UNIT_ASSIGNED_CONTEXT((#52165,#52167,#52168))
REPRESENTATION_CONTEXT('','3D')
);
#52164=(
GEOMETRIC_REPRESENTATION_CONTEXT(3)
GLOBAL_UNCERTAINTY_ASSIGNED_CONTEXT((#52149))
GLOBAL_UNIT_ASSIGNED_CONTEXT((#52165,#52167,#52168))
REPRESENTATION_CONTEXT('','3D')
);
#52165=(
LENGTH_UNIT()
NAMED_UNIT(*)
SI_UNIT(.MILLI.,.METRE.)
);
#52167=(
NAMED_UNIT(*)
PLANE_ANGLE_UNIT()
SI_UNIT($,.RADIAN.)
);
#52168=(
NAMED_UNIT(*)
SI_UNIT($,.STERADIAN.)
SOLID_ANGLE_UNIT()
);
#52177=SHAPE_DEFINITION_REPRESENTATION(#52191,#52218);
#52191=PRODUCT_DEFINITION_SHAPE('',$,#52233);
#52218=SHAPE_REPRESENTATION('',(#9987),#52158);
#52224=PRODUCT_DEFINITION_CONTEXT('part definition',#52268,'design');
#52233=PRODUCT_DEFINITION('Housing / Gear Box Body',
'Housing / Gear Box Body',#52247,#52224);
#52247=PRODUCT_DEFINITION_FORMATION('',$,#52278);
#52268=APPLICATION_CONTEXT('Managed model based 3d engineering');
#52269=PRODUCT_CONTEXT('part definition',#52268,'mechanical');
#52278=PRODUCT('Housing / Gear Box Body','Housing / Gear Box Body',
'NOT SPECIFIED',(#52269));
#52291=COLOUR_RGB('Dark Blue',0.08,0.2,0.34);
#52292=FILL_AREA_STYLE_COLOUR('',#52291);
#52293=FILL_AREA_STYLE('',(#52292));
#52294=SURFACE_STYLE_FILL_AREA(#52293);
#52295=SURFACE_SIDE_STYLE('',(#52294));
#52296=SURFACE_STYLE_USAGE(.BOTH.,#52295);
#52297=PRESENTATION_STYLE_ASSIGNMENT((#52296));
ENDSEC;
END-ISO-10303-21;
